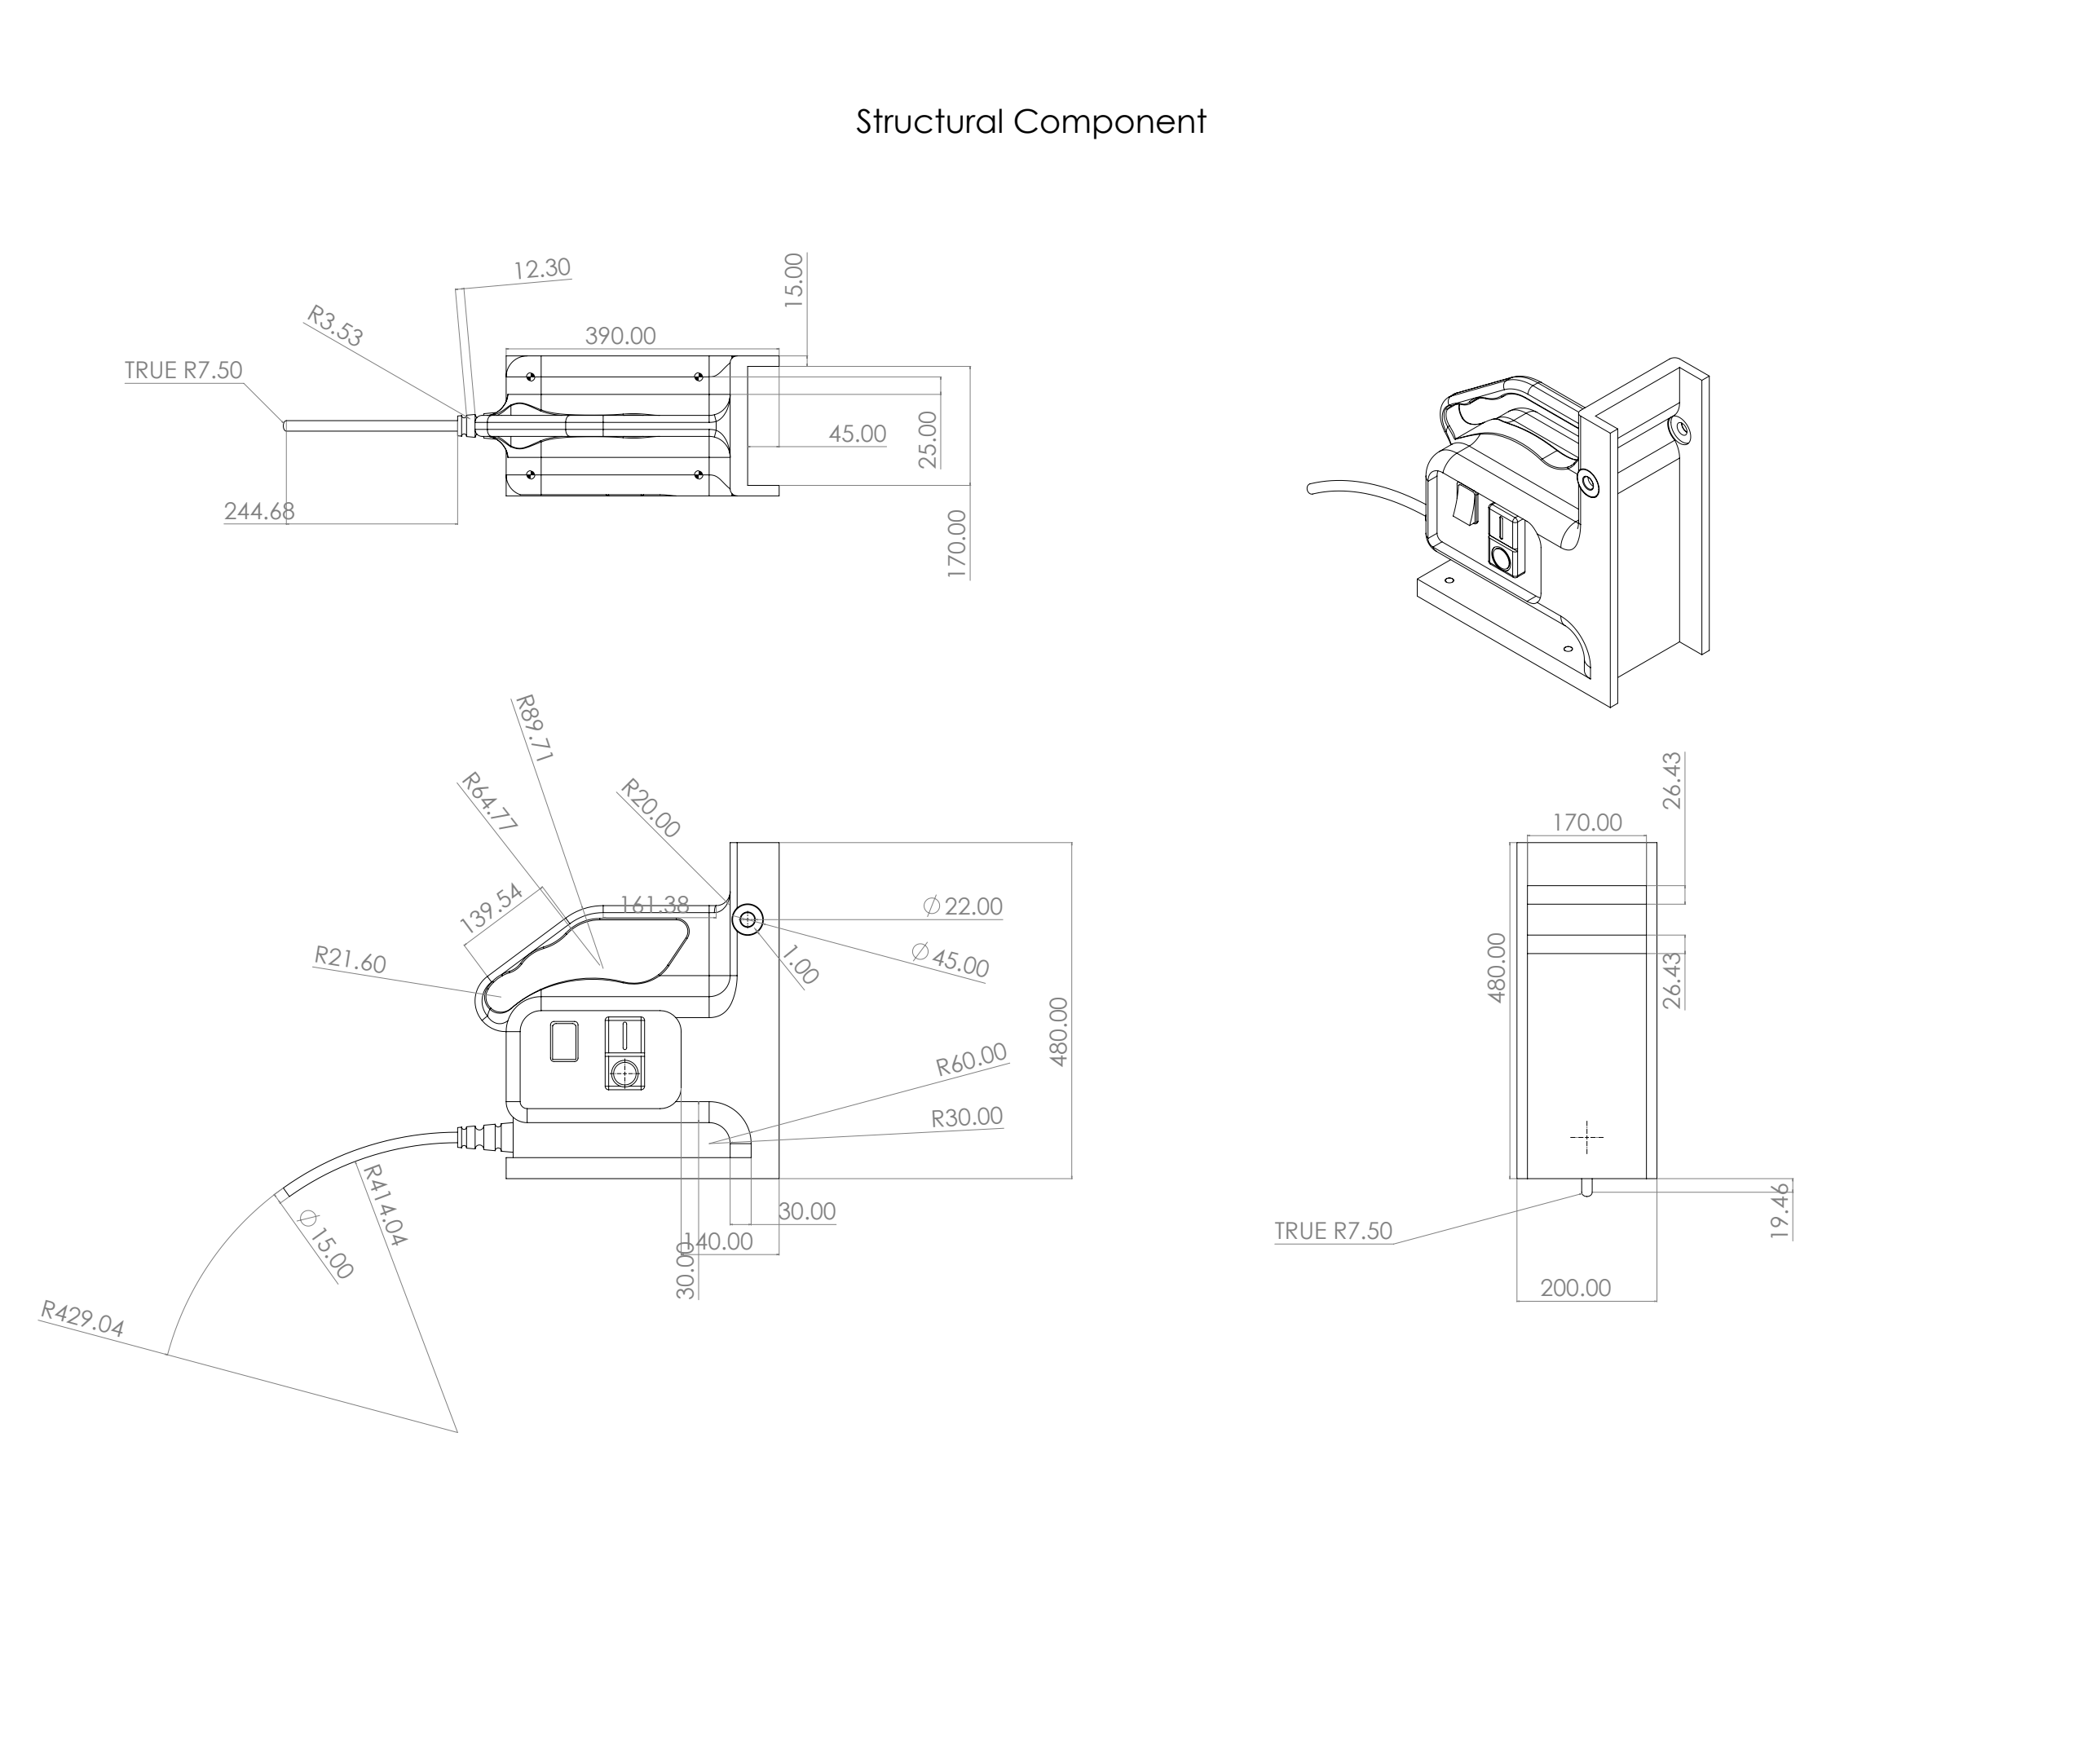
ISO-10303-21;
HEADER;
FILE_DESCRIPTION (('STEP AP214'),
    '1' );
FILE_NAME ('Structural Component.step',
    '2026-10-24T00:09:50',
    ( '' ),
    ( '' ),
    'SwSTEP 2.0',
    'SolidWorks 2025',
    '' );
FILE_SCHEMA (( 'AUTOMOTIVE_DESIGN' ));
ENDSEC;

DATA;
#1=CARTESIAN_POINT ( 'NONE',  ( -209.5848783976569507, 66.48002492874486791, 33.34538701106990288 ) ) ;
#3=DIRECTION ( 'NONE',  ( 0.000000000000000000, 0.000000000000000000, 1.000000000000000000 ) ) ;
#5=EDGE_LOOP ( 'NONE', ( #5978, #27245, #13781, #25937 ) ) ;
#6=CARTESIAN_POINT ( 'NONE',  ( -167.9302994091366088, 116.8073761394556271, 25.31690238253929337 ) ) ;
#7=CARTESIAN_POINT ( 'NONE',  ( -110.7275636018716654, 68.51688903468615877, 83.00000000000001421 ) ) ;
#9=ADVANCED_FACE ( 'NONE', ( #20080 ), #15026, .T. ) ;
#11=ORIENTED_EDGE ( 'NONE', *, *, #16841, .T. ) ;
#13=FACE_OUTER_BOUND ( 'NONE', #24456, .T. ) ;
#15=DIRECTION ( 'NONE',  ( -1.850371707708594316E-16, 1.000000000000000000, 0.000000000000000000 ) ) ;
#18=AXIS2_PLACEMENT_3D ( 'NONE', #21734, #15134, #6353 ) ;
#21=ORIENTED_EDGE ( 'NONE', *, *, #17846, .F. ) ;
#22=CARTESIAN_POINT ( 'NONE',  ( -225.2031547890646266, 89.29438079543466245, 14.16277051160506417 ) ) ;
#24=EDGE_CURVE ( 'NONE', #6807, #15188, #4704, .T. ) ;
#28=AXIS2_PLACEMENT_3D ( 'NONE', #2667, #6838, #19914 ) ;
#38=DIRECTION ( 'NONE',  ( -1.541976423090495387E-16, 1.000000000000000000, -0.000000000000000000 ) ) ;
#43=CARTESIAN_POINT ( 'NONE',  ( -192.2110555254130020, 101.5793329107164027, -32.81765284612617251 ) ) ;
#44=EDGE_LOOP ( 'NONE', ( #26670, #4164, #18942, #22598 ) ) ;
#45=ORIENTED_EDGE ( 'NONE', *, *, #2403, .F. ) ;
#47=AXIS2_PLACEMENT_3D ( 'NONE', #22544, #2851, #8648 ) ;
#50=EDGE_LOOP ( 'NONE', ( #21785, #9635, #7693, #13143 ) ) ;
#52=EDGE_CURVE ( 'NONE', #5857, #12779, #18225, .T. ) ;
#55=DIRECTION ( 'NONE',  ( 1.000000000000000000, 0.000000000000000000, 0.000000000000000000 ) ) ;
#63=CARTESIAN_POINT ( 'NONE',  ( -112.3221550338875687, 74.54464929955099706, 83.00000000000001421 ) ) ;
#66=ORIENTED_EDGE ( 'NONE', *, *, #15793, .T. ) ;
#67=EDGE_CURVE ( 'NONE', #4321, #27397, #9743, .T. ) ;
#69=ORIENTED_EDGE ( 'NONE', *, *, #8545, .T. ) ;
#72=CARTESIAN_POINT ( 'NONE',  ( -242.2383635333241614, 73.34843395317835757, -5.047097023363151358 ) ) ;
#73=CARTESIAN_POINT ( 'NONE',  ( -40.40953891503691153, 36.92584315232891612, 99.00000000000000000 ) ) ;
#84=EDGE_CURVE ( 'NONE', #1460, #15527, #3074, .T. ) ;
#86=DIRECTION ( 'NONE',  ( 0.000000000000000000, 1.000000000000000000, -1.224646799147353207E-16 ) ) ;
#88=VERTEX_POINT ( 'NONE', #22953 ) ;
#90=CARTESIAN_POINT ( 'NONE',  ( 100.8286702512290418, 242.7181571222456284, 23.14229345413787442 ) ) ;
#93=CYLINDRICAL_SURFACE ( 'NONE', #27056, 5.999999999999991118 ) ;
#97=LINE ( 'NONE', #21929, #236 ) ;
#98=CARTESIAN_POINT ( 'NONE',  ( -210.7172313291012529, 103.7585653882801182, 5.000000000000002665 ) ) ;
#99=DIRECTION ( 'NONE',  ( -1.000000000000000000, 0.000000000000000000, 0.000000000000000000 ) ) ;
#101=CARTESIAN_POINT ( 'NONE',  ( 134.9999999999998579, 220.0000000000000284, -99.00000000000001421 ) ) ;
#103=DIRECTION ( 'NONE',  ( 0.5975062131282554700, -0.8018642810807398158, 0.000000000000000000 ) ) ;
#104=ORIENTED_EDGE ( 'NONE', *, *, #18254, .F. ) ;
#115=CARTESIAN_POINT ( 'NONE',  ( -25.41017935548559947, 129.2224694249450181, -15.66087358766781534 ) ) ;
#118=ORIENTED_EDGE ( 'NONE', *, *, #15885, .F. ) ;
#121=ORIENTED_EDGE ( 'NONE', *, *, #12188, .T. ) ;
#122=DIRECTION ( 'NONE',  ( -1.850371707708594316E-16, 1.000000000000000000, -0.000000000000000000 ) ) ;
#124=EDGE_CURVE ( 'NONE', #26591, #26642, #21635, .T. ) ;
#126=DIRECTION ( 'NONE',  ( -1.000000000000000000, 0.000000000000000000, 0.000000000000000000 ) ) ;
#128=CARTESIAN_POINT ( 'NONE',  ( -216.1549772618016334, 59.20708407665082262, 28.62293862808999734 ) ) ;
#132=ADVANCED_FACE ( 'NONE', ( #14200 ), #4989, .F. ) ;
#133=DIRECTION ( 'NONE',  ( 0.000000000000000000, 0.000000000000000000, 1.000000000000000000 ) ) ;
#134=DIRECTION ( 'NONE',  ( -8.673617379884073683E-17, -1.000000000000000000, 0.000000000000000000 ) ) ;
#135=CIRCLE ( 'NONE', #13922, 19.07743405327024888 ) ;
#136=CARTESIAN_POINT ( 'NONE',  ( -203.1779787704217313, 93.05164332230201296, -28.77272332722132475 ) ) ;
#139=DIRECTION ( 'NONE',  ( 0.000000000000000000, 0.000000000000000000, 1.000000000000000000 ) ) ;
#142=EDGE_CURVE ( 'NONE', #11100, #5099, #795, .T. ) ;
#147=LINE ( 'NONE', #4014, #25212 ) ;
#149=EDGE_CURVE ( 'NONE', #7691, #16820, #7209, .T. ) ;
#155=TOROIDAL_SURFACE ( 'NONE', #2900, 39.99999999999999289, 9.999999999999996447 ) ;
#157=CARTESIAN_POINT ( 'NONE',  ( -107.7774523778934253, 133.6573832689441019, 15.67481254453494088 ) ) ;
#158=ORIENTED_EDGE ( 'NONE', *, *, #7014, .F. ) ;
#160=CARTESIAN_POINT ( 'NONE',  ( 94.38583646779612479, 113.6320904522268336, -99.99999999997839950 ) ) ;
#163=CARTESIAN_POINT ( 'NONE',  ( -209.0375512581602493, 88.61097887464748624, 26.00739845333608358 ) ) ;
#165=CARTESIAN_POINT ( 'NONE',  ( -205.7061355896894383, 146.0477147645469813, 12.99999999999999822 ) ) ;
#171=AXIS2_PLACEMENT_3D ( 'NONE', #10028, #18512, #2846 ) ;
#177=CARTESIAN_POINT ( 'NONE',  ( 48.45469728424487244, 192.9461374953035033, 12.99999999999999822 ) ) ;
#182=LINE ( 'NONE', #19713, #24117 ) ;
#183=ORIENTED_EDGE ( 'NONE', *, *, #24834, .F. ) ;
#185=ORIENTED_EDGE ( 'NONE', *, *, #10567, .T. ) ;
#188=CARTESIAN_POINT ( 'NONE',  ( -196.6905515939650400, 98.40619709718011165, -31.75569965019813523 ) ) ;
#192=CARTESIAN_POINT ( 'NONE',  ( -111.8131014667890213, 70.11474204378114905, 82.89209462293977992 ) ) ;
#193=CARTESIAN_POINT ( 'NONE',  ( 109.9999999999998863, 330.0000000000000000, 90.00000000000002842 ) ) ;
#195=ORIENTED_EDGE ( 'NONE', *, *, #27994, .T. ) ;
#197=CARTESIAN_POINT ( 'NONE',  ( -200.0000000000000284, -91.18033988749901653, 21.20097097723064294 ) ) ;
#203=CARTESIAN_POINT ( 'NONE',  ( -209.9813599551185916, 61.38898174817780529, -24.60129468178291035 ) ) ;
#204=CARTESIAN_POINT ( 'NONE',  ( -63.57415822541634043, -18.01420295945611727, 95.00000000000000000 ) ) ;
#205=EDGE_CURVE ( 'NONE', #9863, #2501, #3463, .T. ) ;
#206=EDGE_CURVE ( 'NONE', #17779, #12189, #27834, .T. ) ;
#210=CARTESIAN_POINT ( 'NONE',  ( 184.9999999999999432, 330.0000000000000000, 84.99999999999995737 ) ) ;
#215=EDGE_LOOP ( 'NONE', ( #22439, #1141, #3307, #4955, #12631, #20188 ) ) ;
#218=DIRECTION ( 'NONE',  ( -1.541976423090495387E-16, 1.000000000000000000, 0.000000000000000000 ) ) ;
#223=VERTEX_POINT ( 'NONE', #1394 ) ;
#225=CARTESIAN_POINT ( 'NONE',  ( -210.1746890037166793, 73.83603441591317562, 34.06685219078467242 ) ) ;
#227=ADVANCED_FACE ( 'NONE', ( #3967, #12753 ), #21493, .F. ) ;
#230=VERTEX_POINT ( 'NONE', #6412 ) ;
#235=CARTESIAN_POINT ( 'NONE',  ( -220.9647007329185158, 136.4514858755404987, 12.97939780113086705 ) ) ;
#236=VECTOR ( 'NONE', #2100, 1000.000000000000000 ) ;
#239=CARTESIAN_POINT ( 'NONE',  ( 103.5789823554282947, 245.2557385300782471, 18.86932834259753733 ) ) ;
#240=EDGE_CURVE ( 'NONE', #11439, #27657, #27406, .T. ) ;
#250=DIRECTION ( 'NONE',  ( 8.659560562354934091E-17, 0.7071067811865474617, -0.7071067811865476838 ) ) ;
#253=DIRECTION ( 'NONE',  ( 0.4163300014277677707, -0.9092135777204137792, 0.000000000000000000 ) ) ;
#255=DIRECTION ( 'NONE',  ( 0.000000000000000000, 0.000000000000000000, -1.000000000000000000 ) ) ;
#259=EDGE_CURVE ( 'NONE', #1752, #10216, #14126, .T. ) ;
#261=ORIENTED_EDGE ( 'NONE', *, *, #205, .F. ) ;
#264=AXIS2_PLACEMENT_3D ( 'NONE', #19395, #6183, #2008 ) ;
#266=ORIENTED_EDGE ( 'NONE', *, *, #2989, .F. ) ;
#267=ORIENTED_EDGE ( 'NONE', *, *, #6042, .T. ) ;
#269=DIRECTION ( 'NONE',  ( 0.000000000000000000, 0.000000000000000000, 1.000000000000000000 ) ) ;
#270=CARTESIAN_POINT ( 'NONE',  ( -180.0000000000000284, -40.00000000000004974, 70.00000000000001421 ) ) ;
#277=FACE_OUTER_BOUND ( 'NONE', #22057, .T. ) ;
#279=CARTESIAN_POINT ( 'NONE',  ( -212.2468527728169931, 60.00277588997245459, 15.59298365948827225 ) ) ;
#282=B_SPLINE_CURVE_WITH_KNOTS ( 'NONE', 3,
 ( #2142, #28138, #4579, #11204, #26414, #10916, #13506, #17233, #1, #2281, #25992, #19677, #22257, #19813, #6311, #13087, #23849, #13365 ),
 .UNSPECIFIED., .F., .F.,
 ( 4, 2, 2, 2, 2, 2, 2, 2, 4 ),
 ( -3.464102035643382632E-05, 0.004053789758800030972, 0.008142220537956495682, 0.01223065131711295953, 0.01631908209626942510, 0.02449594365458239789, 0.02654015904416063762, 0.02858437443373887041, 0.03267280521289535333 ),
 .UNSPECIFIED. ) ;
#285=ADVANCED_FACE ( 'NONE', ( #4393 ), #15978, .T. ) ;
#291=CARTESIAN_POINT ( 'NONE',  ( -160.0000000000000284, 119.7660240611718763, 22.85081902853005431 ) ) ;
#292=DIRECTION ( 'NONE',  ( 1.000000000000000000, 0.000000000000000000, 0.000000000000000000 ) ) ;
#294=ORIENTED_EDGE ( 'NONE', *, *, #2530, .T. ) ;
#295=CARTESIAN_POINT ( 'NONE',  ( -222.7702326850704821, 86.58333552780506182, -17.42169760653345634 ) ) ;
#297=CARTESIAN_POINT ( 'NONE',  ( -204.4166662746044665, 91.57150914865317759, -29.20755859028324508 ) ) ;
#303=CARTESIAN_POINT ( 'NONE',  ( -156.4144565615572731, 122.2051147660285579, 19.70699073531202572 ) ) ;
#305=AXIS2_PLACEMENT_3D ( 'NONE', #16749, #21045, #18753 ) ;
#308=CYLINDRICAL_SURFACE ( 'NONE', #13262, 19.07743405327024888 ) ;
#310=ADVANCED_FACE ( 'NONE', ( #4526 ), #6410, .T. ) ;
#311=CARTESIAN_POINT ( 'NONE',  ( -207.4306580894464389, 90.17638659202999918, 25.66226923892150324 ) ) ;
#313=EDGE_CURVE ( 'NONE', #4881, #7087, #25948, .T. ) ;
#318=CIRCLE ( 'NONE', #8106, 1.999999999999994893 ) ;
#319=CARTESIAN_POINT ( 'NONE',  ( -218.1276041038538551, 59.80742093790404112, -25.66002785714302803 ) ) ;
#320=ORIENTED_EDGE ( 'NONE', *, *, #18339, .T. ) ;
#322=CARTESIAN_POINT ( 'NONE',  ( -225.9601317720483280, 132.4444111280268430, -15.07876772300364010 ) ) ;
#323=DIRECTION ( 'NONE',  ( 0.000000000000000000, 0.000000000000000000, 1.000000000000000000 ) ) ;
#328=CARTESIAN_POINT ( 'NONE',  ( -138.6428522700808230, 71.54464929955099706, 82.80879831960034210 ) ) ;
#331=DIRECTION ( 'NONE',  ( -0.6343833064826072121, 0.7730186417261841747, 0.000000000000000000 ) ) ;
#332=CARTESIAN_POINT ( 'NONE',  ( 0.000000000000000000, 0.000000000000000000, 100.0000000000000000 ) ) ;
#335=ORIENTED_EDGE ( 'NONE', *, *, #12580, .F. ) ;
#336=FACE_OUTER_BOUND ( 'NONE', #23638, .T. ) ;
#337=ADVANCED_FACE ( 'NONE', ( #27449 ), #5770, .T. ) ;
#339=DIRECTION ( 'NONE',  ( 0.000000000000000000, 0.000000000000000000, 1.000000000000000000 ) ) ;
#342=DIRECTION ( 'NONE',  ( 1.000000000000000000, 0.000000000000000000, 0.000000000000000000 ) ) ;
#347=CARTESIAN_POINT ( 'NONE',  ( -20.36124356129798940, 129.6266993258962259, -15.48147584998389448 ) ) ;
#349=CARTESIAN_POINT ( 'NONE',  ( -200.0000000000000284, -62.36067977499792647, -25.00000000000000000 ) ) ;
#361=CARTESIAN_POINT ( 'NONE',  ( -212.8228108689317253, 60.01962377528476367, -15.18702394368705910 ) ) ;
#362=DIRECTION ( 'NONE',  ( -0.000000000000000000, -0.000000000000000000, 1.000000000000000000 ) ) ;
#366=VERTEX_POINT ( 'NONE', #3605 ) ;
#373=DIRECTION ( 'NONE',  ( 1.000000000000000000, 0.000000000000000000, 0.000000000000000000 ) ) ;
#377=AXIS2_PLACEMENT_3D ( 'NONE', #16713, #14560, #19139 ) ;
#380=CARTESIAN_POINT ( 'NONE',  ( 93.89426149341781525, 239.9406732612975475, 18.26413231115399682 ) ) ;
#383=DIRECTION ( 'NONE',  ( 0.000000000000000000, 0.000000000000000000, 1.000000000000000000 ) ) ;
#384=DIRECTION ( 'NONE',  ( -0.000000000000000000, -0.000000000000000000, -1.000000000000000000 ) ) ;
#385=DIRECTION ( 'NONE',  ( 0.000000000000000000, 0.000000000000000000, 1.000000000000000000 ) ) ;
#393=DIRECTION ( 'NONE',  ( -0.8498245983676009363, -0.3891357156574876686, 0.3554877590144011057 ) ) ;
#401=DIRECTION ( 'NONE',  ( 0.000000000000000000, 0.000000000000000000, -1.000000000000000000 ) ) ;
#402=ORIENTED_EDGE ( 'NONE', *, *, #11663, .T. ) ;
#406=EDGE_CURVE ( 'NONE', #3986, #26642, #16284, .T. ) ;
#407=VECTOR ( 'NONE', #3303, 1000.000000000000000 ) ;
#408=EDGE_LOOP ( 'NONE', ( #9219, #25469, #5579, #24964 ) ) ;
#411=ORIENTED_EDGE ( 'NONE', *, *, #8546, .F. ) ;
#415=AXIS2_PLACEMENT_3D ( 'NONE', #13536, #20551, #20125 ) ;
#416=CYLINDRICAL_SURFACE ( 'NONE', #20614, 5.000000000000004441 ) ;
#417=CARTESIAN_POINT ( 'NONE',  ( -8.428214953819216149, 132.5195342171013806, 14.39912748063941983 ) ) ;
#419=CARTESIAN_POINT ( 'NONE',  ( -217.7467898461135576, 60.55642267084821384, 12.19614748119721703 ) ) ;
#425=CARTESIAN_POINT ( 'NONE',  ( -42.99650729631200363, 71.03850157808263077, 100.0000000000000000 ) ) ;
#428=AXIS2_PLACEMENT_3D ( 'NONE', #23182, #1479, #8092 ) ;
#429=CARTESIAN_POINT ( 'NONE',  ( 8.117852850209660076, 141.5785587194356481, 12.99999999999999467 ) ) ;
#430=CARTESIAN_POINT ( 'NONE',  ( 109.9999999999999005, 260.0000000000000000, 45.00000000000000000 ) ) ;
#438=VECTOR ( 'NONE', #7033, 1000.000000000000000 ) ;
#439=CARTESIAN_POINT ( 'NONE',  ( -175.0000000000000000, -120.0250000000001904, -76.00000000000000000 ) ) ;
#440=CARTESIAN_POINT ( 'NONE',  ( -203.3278902001933659, 92.92226908766613747, -29.32321494459340627 ) ) ;
#441=ORIENTED_EDGE ( 'NONE', *, *, #25815, .T. ) ;
#442=ORIENTED_EDGE ( 'NONE', *, *, #67, .F. ) ;
#443=ADVANCED_FACE ( 'NONE', ( #16699 ), #5898, .T. ) ;
#445=EDGE_CURVE ( 'NONE', #15077, #27477, #22877, .T. ) ;
#446=CYLINDRICAL_SURFACE ( 'NONE', #26258, 30.00000000000000000 ) ;
#449=ORIENTED_EDGE ( 'NONE', *, *, #2534, .F. ) ;
#453=ORIENTED_EDGE ( 'NONE', *, *, #4349, .T. ) ;
#459=CARTESIAN_POINT ( 'NONE',  ( -213.5622695550096353, 60.06483686772719466, -14.69413405016890017 ) ) ;
#462=CARTESIAN_POINT ( 'NONE',  ( -224.0127348693990257, 134.1242697789267027, -15.11921763785539774 ) ) ;
#466=DIRECTION ( 'NONE',  ( 1.000000000000000000, -0.000000000000000000, 0.000000000000000000 ) ) ;
#467=VECTOR ( 'NONE', #25215, 1000.000000000000000 ) ;
#471=ORIENTED_EDGE ( 'NONE', *, *, #8870, .T. ) ;
#474=VECTOR ( 'NONE', #16394, 1000.000000000000000 ) ;
#476=DIRECTION ( 'NONE',  ( -1.000000000000000000, -9.251858538542961967E-16, 0.000000000000000000 ) ) ;
#480=FACE_OUTER_BOUND ( 'NONE', #21815, .T. ) ;
#483=ORIENTED_EDGE ( 'NONE', *, *, #21141, .F. ) ;
#484=CARTESIAN_POINT ( 'NONE',  ( -40.77925748874363165, 129.1862645484492020, 17.01096724815181460 ) ) ;
#489=CARTESIAN_POINT ( 'NONE',  ( 8.117852850209603233, 141.5785587194356197, -15.00000000000000000 ) ) ;
#490=DIRECTION ( 'NONE',  ( -1.000000000000000000, 0.000000000000000000, 0.000000000000000000 ) ) ;
#492=CIRCLE ( 'NONE', #5533, 1.999999999999996669 ) ;
#493=FACE_OUTER_BOUND ( 'NONE', #792, .T. ) ;
#494=ORIENTED_EDGE ( 'NONE', *, *, #19922, .T. ) ;
#498=DIRECTION ( 'NONE',  ( 1.000000000000000000, -0.000000000000000000, -0.000000000000000000 ) ) ;
#501=LINE ( 'NONE', #24916, #3156 ) ;
#504=FACE_OUTER_BOUND ( 'NONE', #21590, .T. ) ;
#508=EDGE_CURVE ( 'NONE', #26994, #8764, #18328, .T. ) ;
#512=CARTESIAN_POINT ( 'NONE',  ( -207.5836773499184176, 75.53976764568116664, 42.88623166414009091 ) ) ;
#517=ORIENTED_EDGE ( 'NONE', *, *, #21468, .T. ) ;
#520=VECTOR ( 'NONE', #1855, 1000.000000000000000 ) ;
#521=ORIENTED_EDGE ( 'NONE', *, *, #18351, .F. ) ;
#523=CARTESIAN_POINT ( 'NONE',  ( 94.98941689213133088, 231.7050943134730687, 19.00901305069102065 ) ) ;
#527=CARTESIAN_POINT ( 'NONE',  ( -110.3221550338875687, 20.24192588826928585, 83.00000000000001421 ) ) ;
#528=CYLINDRICAL_SURFACE ( 'NONE', #15262, 22.49999999999999289 ) ;
#529=TOROIDAL_SURFACE ( 'NONE', #23467, 19.29759039828519818, 4.355764593064427537 ) ;
#530=CARTESIAN_POINT ( 'NONE',  ( -190.0000000000000284, 59.99999999999995026, 110.0000000000000284 ) ) ;
#533=CARTESIAN_POINT ( 'NONE',  ( 22.58950924271104554, 154.2349915562422780, 12.99999999999999822 ) ) ;
#536=ORIENTED_EDGE ( 'NONE', *, *, #7121, .T. ) ;
#538=CIRCLE ( 'NONE', #24856, 60.90601976618767566 ) ;
#541=CARTESIAN_POINT ( 'NONE',  ( 139.9999999999999716, -120.0000000000000995, 100.0000000000000142 ) ) ;
#544=CARTESIAN_POINT ( 'NONE',  ( 108.8501248000116277, 253.0299650808884735, -36.51570041470898076 ) ) ;
#549=EDGE_CURVE ( 'NONE', #10475, #4407, #3984, .T. ) ;
#554=VECTOR ( 'NONE', #22307, 1000.000000000000000 ) ;
#555=CARTESIAN_POINT ( 'NONE',  ( -92.89766067256680060, 136.4115285999503158, 13.49165197499294599 ) ) ;
#556=DIRECTION ( 'NONE',  ( 1.000000000000000000, 0.000000000000000000, 0.000000000000000000 ) ) ;
#559=CARTESIAN_POINT ( 'NONE',  ( -97.83215868775270962, 136.0971436861518669, -15.20870553203125120 ) ) ;
#562=CARTESIAN_POINT ( 'NONE',  ( -218.4636426211929177, 60.67881959240470735, 11.81164476506740790 ) ) ;
#565=DIRECTION ( 'NONE',  ( 0.5975062131282562472, -0.8018642810807392607, 0.000000000000000000 ) ) ;
#566=CARTESIAN_POINT ( 'NONE',  ( -229.8938360676123978, 91.85985842061924700, -13.11794914285764690 ) ) ;
#567=DIRECTION ( 'NONE',  ( -0.8142945039115421224, -0.5804519453834706688, 0.000000000000000000 ) ) ;
#568=DIRECTION ( 'NONE',  ( 1.000000000000000000, -0.000000000000000000, -0.000000000000000000 ) ) ;
#572=CARTESIAN_POINT ( 'NONE',  ( -18.11108351247773385, 129.9683555792950358, 15.33266781369627907 ) ) ;
#575=CARTESIAN_POINT ( 'NONE',  ( -107.3221550338875687, 17.24192588826928585, 83.00000000000001421 ) ) ;
#576=AXIS2_PLACEMENT_3D ( 'NONE', #27144, #7193, #11366 ) ;
#578=ORIENTED_EDGE ( 'NONE', *, *, #27825, .F. ) ;
#581=DIRECTION ( 'NONE',  ( 1.000000000000000000, 0.000000000000000000, 0.000000000000000000 ) ) ;
#584=EDGE_LOOP ( 'NONE', ( #16630, #25625, #9572, #10611, #8685 ) ) ;
#587=EDGE_CURVE ( 'NONE', #6088, #15077, #9133, .T. ) ;
#589=ORIENTED_EDGE ( 'NONE', *, *, #6265, .F. ) ;
#593=DIRECTION ( 'NONE',  ( 0.000000000000000000, 0.000000000000000000, -1.000000000000000000 ) ) ;
#595=DIRECTION ( 'NONE',  ( 0.000000000000000000, 0.000000000000000000, 1.000000000000000000 ) ) ;
#597=CARTESIAN_POINT ( 'NONE',  ( -205.5646887631684763, 90.70208198090838891, 28.50398098557788273 ) ) ;
#600=EDGE_CURVE ( 'NONE', #17042, #11042, #25180, .T. ) ;
#601=VECTOR ( 'NONE', #28078, 1000.000000000000000 ) ;
#604=CARTESIAN_POINT ( 'NONE',  ( 109.9999999999999005, 240.0000000000000284, 15.00000000000000000 ) ) ;
#605=CARTESIAN_POINT ( 'NONE',  ( -214.3579997887104298, 72.01340221155322752, -27.44224251620622113 ) ) ;
#606=VERTEX_POINT ( 'NONE', #11525 ) ;
#611=CARTESIAN_POINT ( 'NONE',  ( -200.0000000000000284, 0.000000000000000000, -25.00000000000000000 ) ) ;
#614=CARTESIAN_POINT ( 'NONE',  ( 46.79174272583949801, 194.0572550123460474, 12.99999999999999822 ) ) ;
#616=FACE_OUTER_BOUND ( 'NONE', #8502, .T. ) ;
#621=CARTESIAN_POINT ( 'NONE',  ( 81.45493510940914916, 110.0000000000000142, 70.00000000030220804 ) ) ;
#622=CARTESIAN_POINT ( 'NONE',  ( -266.5839533485339530, -91.18033988749901653, -15.26911010665567225 ) ) ;
#623=ORIENTED_EDGE ( 'NONE', *, *, #7231, .T. ) ;
#625=CARTESIAN_POINT ( 'NONE',  ( 134.9999999999998579, 220.0000000000000284, 99.00000000000001421 ) ) ;
#634=DIRECTION ( 'NONE',  ( 0.000000000000000000, 0.000000000000000000, -1.000000000000000000 ) ) ;
#635=CARTESIAN_POINT ( 'NONE',  ( 0.6797495551325769547, 136.5999822166548370, -13.39362083918624968 ) ) ;
#639=CARTESIAN_POINT ( 'NONE',  ( 179.9999999999999147, -150.0000000000000284, 84.99999999999995737 ) ) ;
#644=DIRECTION ( 'NONE',  ( -0.000000000000000000, -0.000000000000000000, -1.000000000000000000 ) ) ;
#647=DIRECTION ( 'NONE',  ( 0.5555587585212683477, 0.8314772792026894344, -0.000000000000000000 ) ) ;
#653=CARTESIAN_POINT ( 'NONE',  ( 109.9999999999999005, 260.0000000000000000, 45.00000000000000000 ) ) ;
#654=ORIENTED_EDGE ( 'NONE', *, *, #6112, .T. ) ;
#656=FACE_OUTER_BOUND ( 'NONE', #25895, .T. ) ;
#657=ORIENTED_EDGE ( 'NONE', *, *, #26807, .T. ) ;
#658=CARTESIAN_POINT ( 'NONE',  ( 91.94652509811839991, 240.0740392588532757, 7.116191647120904129 ) ) ;
#661=ORIENTED_EDGE ( 'NONE', *, *, #5035, .T. ) ;
#665=EDGE_LOOP ( 'NONE', ( #21, #21281, #16990, #8206, #12330, #23398, #10718, #5703 ) ) ;
#667=CARTESIAN_POINT ( 'NONE',  ( 101.4665947576538372, 243.5985648160911410, 15.64809332289330435 ) ) ;
#671=CARTESIAN_POINT ( 'NONE',  ( 65.00000000000000000, -150.0000000000000568, -69.99999999999998579 ) ) ;
#672=CIRCLE ( 'NONE', #14906, 1.999999999999998890 ) ;
#673=ADVANCED_FACE ( 'NONE', ( #13529 ), #308, .F. ) ;
#675=CARTESIAN_POINT ( 'NONE',  ( 81.45493510941093973, 110.0000000000000142, -70.00000000034538061 ) ) ;
#677=FACE_OUTER_BOUND ( 'NONE', #5, .T. ) ;
#682=DIRECTION ( 'NONE',  ( 1.000000000000000000, 0.000000000000000000, 0.000000000000000000 ) ) ;
#683=DIRECTION ( 'NONE',  ( 1.000000000000000000, 0.000000000000000000, 0.000000000000000000 ) ) ;
#687=CYLINDRICAL_SURFACE ( 'NONE', #19940, 10.00000000000000888 ) ;
#688=DIRECTION ( 'NONE',  ( 0.000000000000000000, -1.000000000000000000, 0.000000000000000000 ) ) ;
#691=ORIENTED_EDGE ( 'NONE', *, *, #13967, .F. ) ;
#698=DIRECTION ( 'NONE',  ( 0.000000000000000000, 0.000000000000000000, -1.000000000000000000 ) ) ;
#700=CARTESIAN_POINT ( 'NONE',  ( 87.49999999999990052, 230.0000000000000284, 15.95262490344436657 ) ) ;
#702=ADVANCED_FACE ( 'NONE', ( #13675 ), #26432, .T. ) ;
#703=CARTESIAN_POINT ( 'NONE',  ( -101.5016674773769694, 134.2040548686907755, -15.56499774383584622 ) ) ;
#704=DIRECTION ( 'NONE',  ( -0.000000000000000000, -0.000000000000000000, -1.000000000000000000 ) ) ;
#705=CARTESIAN_POINT ( 'NONE',  ( -195.1986077931981356, 62.83738171803135231, 37.97438512083786577 ) ) ;
#707=CARTESIAN_POINT ( 'NONE',  ( 14.21936997543395798, -49.77566109691134955, 98.36633331184400220 ) ) ;
#708=EDGE_CURVE ( 'NONE', #12779, #28035, #2160, .T. ) ;
#714=VECTOR ( 'NONE', #4678, 1000.000000000000000 ) ;
#715=CARTESIAN_POINT ( 'NONE',  ( 109.9999999999999147, 140.0000000000000000, 90.00000000000002842 ) ) ;
#717=CARTESIAN_POINT ( 'NONE',  ( 65.00000000000000000, -120.0000000000000711, 70.00000000000001421 ) ) ;
#719=CARTESIAN_POINT ( 'NONE',  ( 118.4313905927012343, 122.3304618272157569, -100.0000000000000142 ) ) ;
#724=CARTESIAN_POINT ( 'NONE',  ( -207.1027104522468392, 89.68341047235171004, -27.43904842249505194 ) ) ;
#726=ORIENTED_EDGE ( 'NONE', *, *, #26630, .F. ) ;
#728=CARTESIAN_POINT ( 'NONE',  ( -144.8818860832173527, 126.6487520769749580, 16.84620022481251311 ) ) ;
#731=CARTESIAN_POINT ( 'NONE',  ( -173.1201715254111662, 113.5802963645813151, -28.20029687320744216 ) ) ;
#737=CARTESIAN_POINT ( 'NONE',  ( -203.3278902001933375, 92.92226908766613747, 29.32321494459339561 ) ) ;
#739=LINE ( 'NONE', #24727, #13957 ) ;
#742=CARTESIAN_POINT ( 'NONE',  ( -213.9337484054510128, 55.48171494544713056, -43.35284082257812344 ) ) ;
#746=CARTESIAN_POINT ( 'NONE',  ( -227.8378063125350366, 130.6400894613935577, -13.00000000000000178 ) ) ;
#752=CARTESIAN_POINT ( 'NONE',  ( -236.2622743973914510, 68.21227378728754331, 5.744226217424930780 ) ) ;
#755=AXIS2_PLACEMENT_3D ( 'NONE', #22509, #5114, #11751 ) ;
#757=EDGE_CURVE ( 'NONE', #11653, #6227, #3168, .T. ) ;
#760=FACE_OUTER_BOUND ( 'NONE', #17355, .T. ) ;
#763=CARTESIAN_POINT ( 'NONE',  ( -63.57415822541634043, 0.000000000000000000, 95.00000000000000000 ) ) ;
#764=CARTESIAN_POINT ( 'NONE',  ( -76.25760768171836901, 154.8982798170083299, 12.99999999999999822 ) ) ;
#766=ORIENTED_EDGE ( 'NONE', *, *, #9211, .F. ) ;
#769=CIRCLE ( 'NONE', #28282, 17.46154499483315448 ) ;
#770=DIRECTION ( 'NONE',  ( -0.000000000000000000, -0.000000000000000000, 1.000000000000000000 ) ) ;
#771=CARTESIAN_POINT ( 'NONE',  ( 33.10302365956999182, 219.6666220619077876, -13.00000000000000000 ) ) ;
#773=CARTESIAN_POINT ( 'NONE',  ( -7.443950587159290144, 132.8771115358387931, -14.28760955781909381 ) ) ;
#774=FACE_OUTER_BOUND ( 'NONE', #27445, .T. ) ;
#777=DIRECTION ( 'NONE',  ( 1.000000000000000000, 0.000000000000000000, 0.000000000000000000 ) ) ;
#782=FACE_OUTER_BOUND ( 'NONE', #22813, .T. ) ;
#783=DIRECTION ( 'NONE',  ( 0.000000000000000000, 0.000000000000000000, -1.000000000000000000 ) ) ;
#786=ORIENTED_EDGE ( 'NONE', *, *, #2510, .F. ) ;
#792=EDGE_LOOP ( 'NONE', ( #26456, #9388, #18385, #15458, #18561, #10831 ) ) ;
#795=CIRCLE ( 'NONE', #16840, 9.999999999999994671 ) ;
#796=FACE_OUTER_BOUND ( 'NONE', #27107, .T. ) ;
#801=EDGE_CURVE ( 'NONE', #19503, #8160, #22570, .T. ) ;
#804=EDGE_CURVE ( 'NONE', #2005, #223, #27933, .T. ) ;
#807=CARTESIAN_POINT ( 'NONE',  ( 109.9999999999999005, 259.1520133602594456, 44.26562200907745392 ) ) ;
#808=DIRECTION ( 'NONE',  ( -8.673617379884036705E-17, 1.000000000000000000, 0.000000000000000000 ) ) ;
#811=CARTESIAN_POINT ( 'NONE',  ( 85.90765579575543143, 110.5723347142871091, -70.58593750016461854 ) ) ;
#815=CARTESIAN_POINT ( 'NONE',  ( 65.00000000000000000, -150.0000000000000568, 70.00000000000001421 ) ) ;
#820=ORIENTED_EDGE ( 'NONE', *, *, #24259, .F. ) ;
#822=LINE ( 'NONE', #541, #8481 ) ;
#823=CARTESIAN_POINT ( 'NONE',  ( -273.6211430000234373, -91.18033988749901653, 0.000000000000000000 ) ) ;
#827=ORIENTED_EDGE ( 'NONE', *, *, #20728, .F. ) ;
#830=EDGE_CURVE ( 'NONE', #12559, #10408, #23836, .T. ) ;
#832=ORIENTED_EDGE ( 'NONE', *, *, #20807, .T. ) ;
#834=ORIENTED_EDGE ( 'NONE', *, *, #1618, .F. ) ;
#835=CARTESIAN_POINT ( 'NONE',  ( -151.8667954808881291, 124.0669258736115523, 18.37961917418349955 ) ) ;
#841=CARTESIAN_POINT ( 'NONE',  ( -31.50743868999440167, 129.2243496464543284, 15.65998950894569752 ) ) ;
#842=CARTESIAN_POINT ( 'NONE',  ( -195.0250397031994112, 62.90385929084195737, 38.63509848415888115 ) ) ;
#846=CARTESIAN_POINT ( 'NONE',  ( 79.99999999999994316, 109.9999999999999716, -71.96349540849364246 ) ) ;
#847=VECTOR ( 'NONE', #18718, 1000.000000000000114 ) ;
#848=CARTESIAN_POINT ( 'NONE',  ( -207.3935809773778942, 90.19561752971078761, -25.69361353241580304 ) ) ;
#850=DIRECTION ( 'NONE',  ( 0.000000000000000000, 0.000000000000000000, 1.000000000000000000 ) ) ;
#851=CARTESIAN_POINT ( 'NONE',  ( 87.74278500247204704, 111.0010834413667453, 71.13281249985656984 ) ) ;
#853=CARTESIAN_POINT ( 'NONE',  ( 113.4920585194047078, 104.4775165427241461, -100.0000000000000142 ) ) ;
#859=DIRECTION ( 'NONE',  ( -1.000000000000000000, 0.000000000000000000, 0.000000000000000000 ) ) ;
#861=ORIENTED_EDGE ( 'NONE', *, *, #22149, .F. ) ;
#866=EDGE_CURVE ( 'NONE', #16598, #10685, #5021, .T. ) ;
#871=DIRECTION ( 'NONE',  ( 1.000000000000000000, 3.469446951953614189E-16, -0.000000000000000000 ) ) ;
#877=CARTESIAN_POINT ( 'NONE',  ( -199.5809478526699650, 61.42778479158862126, -28.44561038857050761 ) ) ;
#887=DIRECTION ( 'NONE',  ( -0.000000000000000000, 1.000000000000000000, -0.000000000000000000 ) ) ;
#888=EDGE_LOOP ( 'NONE', ( #23960, #2470, #23686, #8733 ) ) ;
#891=CARTESIAN_POINT ( 'NONE',  ( -279.3160071107327553, -91.18033988749901653, 0.000000000000000000 ) ) ;
#896=AXIS2_PLACEMENT_3D ( 'NONE', #9883, #3402, #7727 ) ;
#903=ORIENTED_EDGE ( 'NONE', *, *, #6405, .T. ) ;
#907=CIRCLE ( 'NONE', #10544, 30.00000000000000000 ) ;
#910=CARTESIAN_POINT ( 'NONE',  ( 7.502017008525952768, 138.6551571308461348, -15.00000000000000000 ) ) ;
#912=EDGE_CURVE ( 'NONE', #25311, #7612, #22460, .T. ) ;
#917=FACE_OUTER_BOUND ( 'NONE', #15898, .T. ) ;
#919=LINE ( 'NONE', #10110, #24476 ) ;
#922=CIRCLE ( 'NONE', #10088, 68.83858790703926900 ) ;
#928=ORIENTED_EDGE ( 'NONE', *, *, #17521, .F. ) ;
#929=DIRECTION ( 'NONE',  ( 1.000000000000000000, 0.000000000000000000, 0.000000000000000000 ) ) ;
#933=EDGE_LOOP ( 'NONE', ( #25332, #26932, #17589, #8882, #1061, #19824, #4317, #18042 ) ) ;
#937=ADVANCED_FACE ( 'NONE', ( #14514, #19097, #8178, #25421, #14651 ), #23838, .F. ) ;
#938=CIRCLE ( 'NONE', #21121, 18.91107291867258411 ) ;
#943=VECTOR ( 'NONE', #21161, 1000.000000000000000 ) ;
#944=DIRECTION ( 'NONE',  ( -0.000000000000000000, -1.000000000000000000, -0.000000000000000000 ) ) ;
#945=DIRECTION ( 'NONE',  ( 1.000000000000000000, 0.000000000000000000, 0.000000000000000000 ) ) ;
#946=EDGE_CURVE ( 'NONE', #12013, #2614, #5471, .T. ) ;
#947=CARTESIAN_POINT ( 'NONE',  ( 104.1118574119011555, 122.0584436052145918, -84.84374999967577935 ) ) ;
#955=ORIENTED_EDGE ( 'NONE', *, *, #8077, .T. ) ;
#960=ADVANCED_FACE ( 'NONE', ( #5736 ), #3715, .T. ) ;
#961=FACE_OUTER_BOUND ( 'NONE', #3277, .T. ) ;
#970=VERTEX_POINT ( 'NONE', #8325 ) ;
#971=CARTESIAN_POINT ( 'NONE',  ( -81.43952348080793513, 136.3896988708861215, 13.49547953233103392 ) ) ;
#977=AXIS2_PLACEMENT_3D ( 'NONE', #1019, #14248, #3304 ) ;
#980=CARTESIAN_POINT ( 'NONE',  ( -122.9477694338266360, 132.7606495686108872, -14.33686514723054373 ) ) ;
#986=CARTESIAN_POINT ( 'NONE',  ( 33.10302365956999182, 203.2034914284457159, -15.00000000000000000 ) ) ;
#987=ADVANCED_FACE ( 'NONE', ( #25840 ), #26568, .T. ) ;
#989=CARTESIAN_POINT ( 'NONE',  ( 119.9999999999999147, 140.0000000000000000, -100.0000000000000142 ) ) ;
#990=DIRECTION ( 'NONE',  ( 0.000000000000000000, 0.000000000000000000, 1.000000000000000000 ) ) ;
#993=CIRCLE ( 'NONE', #27137, 166.0121251338587172 ) ;
#997=EDGE_LOOP ( 'NONE', ( #19109, #27348, #25490, #11756, #45, #10235 ) ) ;
#998=CIRCLE ( 'NONE', #19800, 5.000000000000004441 ) ;
#1000=ORIENTED_EDGE ( 'NONE', *, *, #28394, .T. ) ;
#1001=DIRECTION ( 'NONE',  ( -1.850371707708594316E-16, 1.000000000000000000, 0.000000000000000000 ) ) ;
#1004=DIRECTION ( 'NONE',  ( -0.7892793597178160425, -0.6140342761796236948, 0.000000000000000000 ) ) ;
#1006=CARTESIAN_POINT ( 'NONE',  ( -20.22388308534250712, 128.4000958562204460, -17.33254599016412101 ) ) ;
#1008=DIRECTION ( 'NONE',  ( -0.5555587585212683477, -0.8314772792026894344, -0.000000000000000000 ) ) ;
#1009=EDGE_CURVE ( 'NONE', #27752, #3252, #23271, .T. ) ;
#1010=AXIS2_PLACEMENT_3D ( 'NONE', #4400, #24228, #2669 ) ;
#1014=EDGE_CURVE ( 'NONE', #9382, #18102, #26729, .T. ) ;
#1015=AXIS2_PLACEMENT_3D ( 'NONE', #23644, #1520, #25373 ) ;
#1019=CARTESIAN_POINT ( 'NONE',  ( 139.9999999999999716, -120.0000000000000284, 70.00000000000001421 ) ) ;
#1020=FACE_OUTER_BOUND ( 'NONE', #12119, .T. ) ;
#1024=CARTESIAN_POINT ( 'NONE',  ( -242.2202452113856737, 73.32912780459425051, 5.047888127315641960 ) ) ;
#1026=ORIENTED_EDGE ( 'NONE', *, *, #13555, .T. ) ;
#1030=AXIS2_PLACEMENT_3D ( 'NONE', #19427, #23883, #12979 ) ;
#1031=CARTESIAN_POINT ( 'NONE',  ( 84.91648909967247505, 110.3843228249417479, 70.37109374985131183 ) ) ;
#1036=FACE_OUTER_BOUND ( 'NONE', #18183, .T. ) ;
#1037=TOROIDAL_SURFACE ( 'NONE', #14808, 18.46313063346208239, 2.000000000000000000 ) ;
#1038=DIRECTION ( 'NONE',  ( 0.000000000000000000, 0.000000000000000000, 1.000000000000000000 ) ) ;
#1045=ADVANCED_FACE ( 'NONE', ( #24257 ), #7016, .F. ) ;
#1046=ADVANCED_FACE ( 'NONE', ( #26122 ), #416, .T. ) ;
#1050=FACE_OUTER_BOUND ( 'NONE', #10538, .T. ) ;
#1053=DIRECTION ( 'NONE',  ( 0.000000000000000000, -1.000000000000000000, 0.000000000000000000 ) ) ;
#1054=ORIENTED_EDGE ( 'NONE', *, *, #15982, .F. ) ;
#1055=CIRCLE ( 'NONE', #14355, 15.26911010665567225 ) ;
#1058=CARTESIAN_POINT ( 'NONE',  ( -225.3736415174280978, 135.7651958811247539, 14.97905406095859426 ) ) ;
#1061=ORIENTED_EDGE ( 'NONE', *, *, #4761, .T. ) ;
#1062=LINE ( 'NONE', #26784, #6383 ) ;
#1063=VERTEX_POINT ( 'NONE', #2268 ) ;
#1065=CARTESIAN_POINT ( 'NONE',  ( -110.3221550338875687, 20.24192588826927164, 93.88690167569080813 ) ) ;
#1068=ORIENTED_EDGE ( 'NONE', *, *, #27119, .F. ) ;
#1071=CARTESIAN_POINT ( 'NONE',  ( -107.6172385141402259, 133.6752736189426969, 15.67102466709354935 ) ) ;
#1074=VECTOR ( 'NONE', #4601, 1000.000000000000000 ) ;
#1081=AXIS2_PLACEMENT_3D ( 'NONE', #9761, #10179, #23111 ) ;
#1082=CARTESIAN_POINT ( 'NONE',  ( 109.1380356258735134, 251.5976846382455676, 37.70750237629315649 ) ) ;
#1085=CARTESIAN_POINT ( 'NONE',  ( 9.999999999999738876, -50.00000000000004263, 98.28427124746191623 ) ) ;
#1087=CARTESIAN_POINT ( 'NONE',  ( -180.0000000000000000, -40.00000000000004974, -100.0000000000000142 ) ) ;
#1097=CARTESIAN_POINT ( 'NONE',  ( 90.99996269066551235, 240.0000000000000853, -6.657450422703546700 ) ) ;
#1098=DIRECTION ( 'NONE',  ( 1.000000000000000000, 0.000000000000000000, 0.000000000000000000 ) ) ;
#1100=CARTESIAN_POINT ( 'NONE',  ( -76.25760768171836901, 154.8982798170083299, -15.00000000000000000 ) ) ;
#1107=ADVANCED_FACE ( 'NONE', ( #10905 ), #6589, .F. ) ;
#1112=ORIENTED_EDGE ( 'NONE', *, *, #27771, .F. ) ;
#1113=CARTESIAN_POINT ( 'NONE',  ( -137.6741556889342633, 128.9596988076234823, 15.73777296567075901 ) ) ;
#1116=LINE ( 'NONE', #16360, #2392 ) ;
#1117=CARTESIAN_POINT ( 'NONE',  ( -47.64428992525972717, 132.2658675021500301, -15.94853873366968955 ) ) ;
#1123=DIRECTION ( 'NONE',  ( -0.000000000000000000, -0.000000000000000000, 1.000000000000000000 ) ) ;
#1124=FACE_OUTER_BOUND ( 'NONE', #12500, .T. ) ;
#1128=EDGE_CURVE ( 'NONE', #12217, #24673, #907, .T. ) ;
#1130=CARTESIAN_POINT ( 'NONE',  ( -186.0376809321689393, 105.9168515575387062, 32.47349478036296233 ) ) ;
#1136=ORIENTED_EDGE ( 'NONE', *, *, #1662, .T. ) ;
#1141=ORIENTED_EDGE ( 'NONE', *, *, #26039, .F. ) ;
#1143=ADVANCED_FACE ( 'NONE', ( #13642, #22387 ), #8608, .F. ) ;
#1145=EDGE_CURVE ( 'NONE', #3426, #23655, #17362, .T. ) ;
#1146=B_SPLINE_CURVE_WITH_KNOTS ( 'NONE', 3,
 ( #2986, #11778, #20518, #7017, #841, #18510, #9609, #18369, #24975, #11341, #5288, #27256, #7596, #417, #17936, #16878, #3261, #27389, #1643, #3936, #14876, #10412 ),
 .UNSPECIFIED., .F., .F.,
 ( 4, 2, 2, 2, 2, 2, 2, 2, 2, 2, 4 ),
 ( 0.000000000000000000, 0.006705097167734689993, 0.01341019433546937999, 0.01676274291933672195, 0.02011529150320406911, 0.02682038867093874610, 0.03352548583867343002, 0.03687803442254078412, 0.04023058300640813129, 0.04693568017414279786, 0.05364077734187745750 ),
 .UNSPECIFIED. ) ;
#1150=VECTOR ( 'NONE', #20971, 1000.000000000000000 ) ;
#1153=CARTESIAN_POINT ( 'NONE',  ( -21.33210486176665910, 0.000000000000000000, 99.00000000000000000 ) ) ;
#1156=CARTESIAN_POINT ( 'NONE',  ( -219.5652642369064722, 71.26897287455133778, -22.07429503402158488 ) ) ;
#1159=DIRECTION ( 'NONE',  ( 0.000000000000000000, 0.000000000000000000, -1.000000000000000000 ) ) ;
#1162=CARTESIAN_POINT ( 'NONE',  ( 116.8936292565958439, 233.3691281929210959, -99.51164200157825235 ) ) ;
#1164=EDGE_LOOP ( 'NONE', ( #14157, #27836 ) ) ;
#1166=VECTOR ( 'NONE', #3193, 1000.000000000000000 ) ;
#1174=EDGE_CURVE ( 'NONE', #22407, #11012, #9175, .T. ) ;
#1184=ORIENTED_EDGE ( 'NONE', *, *, #2530, .F. ) ;
#1185=CARTESIAN_POINT ( 'NONE',  ( -37.82257053376181233, 36.92584315232891612, 99.00000000000000000 ) ) ;
#1187=AXIS2_PLACEMENT_3D ( 'NONE', #15807, #5001, #8754 ) ;
#1190=AXIS2_PLACEMENT_3D ( 'NONE', #25235, #16624, #25381 ) ;
#1192=CARTESIAN_POINT ( 'NONE',  ( -185.4366074710545433, 106.2948058035834435, -32.30162111875018383 ) ) ;
#1196=DIRECTION ( 'NONE',  ( -0.000000000000000000, 1.000000000000000000, -1.387778780781445429E-16 ) ) ;
#1199=ORIENTED_EDGE ( 'NONE', *, *, #6700, .F. ) ;
#1206=ORIENTED_EDGE ( 'NONE', *, *, #3981, .T. ) ;
#1211=DIRECTION ( 'NONE',  ( 0.000000000000000000, 0.000000000000000000, 1.000000000000000000 ) ) ;
#1214=AXIS2_PLACEMENT_3D ( 'NONE', #8774, #10932, #19691 ) ;
#1219=ADVANCED_FACE ( 'NONE', ( #9748 ), #9363, .T. ) ;
#1222=ORIENTED_EDGE ( 'NONE', *, *, #3961, .F. ) ;
#1225=DIRECTION ( 'NONE',  ( 2.312964634635742464E-16, -1.000000000000000000, 2.139922160430262010E-31 ) ) ;
#1226=FACE_OUTER_BOUND ( 'NONE', #27486, .T. ) ;
#1227=CARTESIAN_POINT ( 'NONE',  ( 90.92319367352099846, 112.0484670279005570, -72.65625000014701129 ) ) ;
#1233=DIRECTION ( 'NONE',  ( 1.000000000000000000, 0.000000000000000000, 0.000000000000000000 ) ) ;
#1236=CARTESIAN_POINT ( 'NONE',  ( -20.04511428896995895, 128.4222523959858222, 17.32321537865083982 ) ) ;
#1239=CYLINDRICAL_SURFACE ( 'NONE', #18735, 49.99999999999998579 ) ;
#1241=EDGE_CURVE ( 'NONE', #27002, #15645, #1541, .T. ) ;
#1244=CARTESIAN_POINT ( 'NONE',  ( 134.9999999999998579, 220.0000000000000284, -84.99999999999997158 ) ) ;
#1249=ADVANCED_FACE ( 'NONE', ( #27949 ), #10306, .F. ) ;
#1250=ORIENTED_EDGE ( 'NONE', *, *, #17544, .T. ) ;
#1252=CARTESIAN_POINT ( 'NONE',  ( 115.1343022193454146, 230.6109841179907960, 98.75454612047967373 ) ) ;
#1254=FACE_OUTER_BOUND ( 'NONE', #3361, .T. ) ;
#1256=VECTOR ( 'NONE', #4847, 1000.000000000000000 ) ;
#1258=CARTESIAN_POINT ( 'NONE',  ( -151.7779492149703913, 124.0884682837862556, -18.38425441931939375 ) ) ;
#1266=CARTESIAN_POINT ( 'NONE',  ( -200.0000000000000284, -91.18033988749901653, 21.20097097723064294 ) ) ;
#1269=CIRCLE ( 'NONE', #23741, 30.00000000000000000 ) ;
#1270=DIRECTION ( 'NONE',  ( 1.000000000000000000, 0.000000000000000000, 0.000000000000000000 ) ) ;
#1271=CARTESIAN_POINT ( 'NONE',  ( -195.0490684805821502, 99.44477443395156513, 32.51470260376371613 ) ) ;
#1272=ORIENTED_EDGE ( 'NONE', *, *, #22671, .T. ) ;
#1275=ADVANCED_FACE ( 'NONE', ( #6416 ), #19630, .F. ) ;
#1277=ORIENTED_EDGE ( 'NONE', *, *, #5268, .T. ) ;
#1281=ORIENTED_EDGE ( 'NONE', *, *, #5887, .F. ) ;
#1285=AXIS2_PLACEMENT_3D ( 'NONE', #5855, #5577, #9897 ) ;
#1286=EDGE_CURVE ( 'NONE', #7257, #11179, #2231, .T. ) ;
#1288=DIRECTION ( 'NONE',  ( 0.000000000000000000, -1.387778780781445429E-16, -1.000000000000000000 ) ) ;
#1289=( BOUNDED_SURFACE ( )  B_SPLINE_SURFACE ( 3, 2, ( 
 ( #15390, #440, #21979 ),
 ( #2576, #8913, #24144 ),
 ( #297, #22269, #11067 ),
 ( #9054, #19823, #17667 ),
 ( #17808, #24277, #22122 ),
 ( #6892, #15673, #24422 ),
 ( #4731, #13516, #11361 ),
 ( #26712, #15822, #1683 ),
 ( #14914, #2101, #26237 ),
 ( #1819, #10451, #6564 ),
 ( #19636, #28098, #10881 ),
 ( #28373, #23668, #15196 ),
 ( #17055, #27954, #8720 ),
 ( #4262, #25670, #12625 ),
 ( #14770, #4117, #8297 ),
 ( #10311, #25812, #13047 ),
 ( #5993, #23809, #8584 ),
 ( #8442, #17473, #12482 ),
 ( #6139, #17198, #3974 ),
 ( #19070, #12761, #21501 ),
 ( #12902, #28240, #15051 ),
 ( #19209, #10593, #19349 ),
 ( #25956, #15342, #21796 ),
 ( #21363, #23523, #3689 ),
 ( #21222, #6277, #21649 ),
 ( #1545, #27815, #8153 ),
 ( #16914, #1959, #3836 ),
 ( #10742, #19496, #17333 ) ),
 .UNSPECIFIED., .F., .F., .F. ) 
 B_SPLINE_SURFACE_WITH_KNOTS ( ( 4, 2, 2, 2, 2, 2, 2, 2, 2, 2, 2, 2, 2, 4 ),
 ( 3, 3 ),
 ( -4.336808689942017736E-19, 0.002390588749581671821, 0.004781177499163344509, 0.007171766248745017197, 0.009562354998326689018, 0.01434353249749003439, 0.01912470999665337804, 0.02151529874623504812, 0.02390588749581672168, 0.02629647624539839523, 0.02868706499498006879, 0.03346824249414341590, 0.03585883124372508945, 0.03824941999330675607 ),
 ( 0.000000000000000000, 1.000000000000000000 ),
 .UNSPECIFIED. ) 
 GEOMETRIC_REPRESENTATION_ITEM ( )  RATIONAL_B_SPLINE_SURFACE ( (
 ( 1.000000000000000000, 0.9597817246759324794, 1.000000000000000000),
 ( 1.000000000000000000, 0.9562412905049657574, 1.000000000000000000),
 ( 1.000000000000000000, 0.9518158024554053132, 1.000000000000000000),
 ( 1.000000000000000000, 0.9416816922015391889, 1.000000000000000000),
 ( 1.000000000000000000, 0.9359714045868776644, 1.000000000000000000),
 ( 1.000000000000000000, 0.9235548114045784018, 1.000000000000000000),
 ( 1.000000000000000000, 0.9168457509165021113, 1.000000000000000000),
 ( 1.000000000000000000, 0.9026276550354167538, 1.000000000000000000),
 ( 1.000000000000000000, 0.8950913600786598590, 1.000000000000000000),
 ( 1.000000000000000000, 0.8718270562173044969, 1.000000000000000000),
 ( 1.000000000000000000, 0.8553941770535198330, 1.000000000000000000),
 ( 1.000000000000000000, 0.8221312774674292001, 1.000000000000000000),
 ( 1.000000000000000000, 0.8052879325280857259, 1.000000000000000000),
 ( 1.000000000000000000, 0.7809787548410676017, 1.000000000000000000),
 ( 1.000000000000000000, 0.7730264403491060587, 1.000000000000000000),
 ( 1.000000000000000000, 0.7580280365901805872, 1.000000000000000000),
 ( 1.000000000000000000, 0.7509406410103288687, 1.000000000000000000),
 ( 1.000000000000000000, 0.7378319876417124279, 1.000000000000000000),
 ( 1.000000000000000000, 0.7318106482057810114, 1.000000000000000000),
 ( 1.000000000000000000, 0.7210845397427231296, 1.000000000000000000),
 ( 1.000000000000000000, 0.7163689906379826500, 1.000000000000000000),
 ( 1.000000000000000000, 0.7048488289897706371, 1.000000000000000000),
 ( 1.000000000000000000, 0.7005414584674227729, 1.000000000000000000),
 ( 1.000000000000000000, 0.6992757048208856352, 1.000000000000000000),
 ( 1.000000000000000000, 0.6997273220235887825, 1.000000000000000000),
 ( 1.000000000000000000, 0.7022627928042818324, 1.000000000000000000),
 ( 1.000000000000000000, 0.7043340258885323335, 1.000000000000000000),
 ( 1.000000000000000000, 0.7071067811865493491, 1.000000000000000000) ) ) 
 REPRESENTATION_ITEM ( '' )  SURFACE ( )  );
#1294=CARTESIAN_POINT ( 'NONE',  ( -194.3369914945607491, 63.17511408073718826, -42.65718952139617670 ) ) ;
#1295=EDGE_CURVE ( 'NONE', #18743, #15118, #13304, .T. ) ;
#1300=FACE_OUTER_BOUND ( 'NONE', #3508, .T. ) ;
#1304=AXIS2_PLACEMENT_3D ( 'NONE', #14317, #27788, #3096 ) ;
#1305=AXIS2_PLACEMENT_3D ( 'NONE', #15444, #19733, #490 ) ;
#1306=FACE_OUTER_BOUND ( 'NONE', #8945, .T. ) ;
#1309=ORIENTED_EDGE ( 'NONE', *, *, #3636, .T. ) ;
#1311=CARTESIAN_POINT ( 'NONE',  ( 100.8904249506254018, 86.57652225510716448, 100.0000000000000142 ) ) ;
#1315=CARTESIAN_POINT ( 'NONE',  ( -175.0000000000000000, -150.0000000000000853, 70.00000000000001421 ) ) ;
#1316=DIRECTION ( 'NONE',  ( 1.000000000000000000, 0.000000000000000000, 0.000000000000000000 ) ) ;
#1321=CARTESIAN_POINT ( 'NONE',  ( 96.76194576697650973, 83.89264379418858653, 100.0000000000000142 ) ) ;
#1323=DIRECTION ( 'NONE',  ( -1.000000000000000000, 0.000000000000000000, 0.000000000000000000 ) ) ;
#1324=AXIS2_PLACEMENT_3D ( 'NONE', #25707, #23704, #14811 ) ;
#1326=CARTESIAN_POINT ( 'NONE',  ( 6.071532165918828775E-15, -70.00000000000002842, 25.00000000000000000 ) ) ;
#1331=LINE ( 'NONE', #16710, #7843 ) ;
#1333=VERTEX_POINT ( 'NONE', #6835 ) ;
#1335=DIRECTION ( 'NONE',  ( 0.000000000000000000, 0.000000000000000000, -1.000000000000000000 ) ) ;
#1342=VERTEX_POINT ( 'NONE', #15617 ) ;
#1343=CIRCLE ( 'NONE', #4083, 70.83858790703926900 ) ;
#1344=CARTESIAN_POINT ( 'NONE',  ( -173.6192398023450494, 113.7611339081862667, 27.04214115208617031 ) ) ;
#1346=FACE_OUTER_BOUND ( 'NONE', #4307, .T. ) ;
#1348=CARTESIAN_POINT ( 'NONE',  ( -37.82257053376181233, 71.03850157808263077, 100.0000000000000000 ) ) ;
#1352=AXIS2_PLACEMENT_3D ( 'NONE', #2714, #11503, #20243 ) ;
#1354=CARTESIAN_POINT ( 'NONE',  ( 109.9999999999998721, 259.8688628429572987, 44.77286377382201010 ) ) ;
#1357=AXIS2_PLACEMENT_3D ( 'NONE', #25698, #14796, #12504 ) ;
#1358=CARTESIAN_POINT ( 'NONE',  ( 22.58950924271108107, 154.2349915562422495, -15.00000000000000000 ) ) ;
#1359=ORIENTED_EDGE ( 'NONE', *, *, #25587, .T. ) ;
#1362=VERTEX_POINT ( 'NONE', #24090 ) ;
#1364=CIRCLE ( 'NONE', #18795, 9.999999999999994671 ) ;
#1369=CIRCLE ( 'NONE', #17420, 11.00000000000001066 ) ;
#1372=LINE ( 'NONE', #25920, #24620 ) ;
#1374=CARTESIAN_POINT ( 'NONE',  ( 9.999999999999749534, 90.00000000000001421, 98.28427124746191623 ) ) ;
#1376=DIRECTION ( 'NONE',  ( -1.000000000000000000, 0.000000000000000000, 0.000000000000000000 ) ) ;
#1381=CARTESIAN_POINT ( 'NONE',  ( 102.1958639858411004, 244.1335791876568919, -16.70126253799778482 ) ) ;
#1383=DIRECTION ( 'NONE',  ( -0.000000000000000000, -0.000000000000000000, -1.000000000000000000 ) ) ;
#1390=VERTEX_POINT ( 'NONE', #8577 ) ;
#1391=CARTESIAN_POINT ( 'NONE',  ( -75.10678314939089262, 136.1130475173332570, 15.20604832699645392 ) ) ;
#1393=VERTEX_POINT ( 'NONE', #17329 ) ;
#1394=CARTESIAN_POINT ( 'NONE',  ( -71.37541315349507443, 240.0000000000000000, -5.000000000000004441 ) ) ;
#1395=CARTESIAN_POINT ( 'NONE',  ( 79.99999999999990052, 140.0000000000000000, 45.00000000000000000 ) ) ;
#1396=DIRECTION ( 'NONE',  ( 0.000000000000000000, -1.000000000000000000, 0.000000000000000000 ) ) ;
#1397=CARTESIAN_POINT ( 'NONE',  ( -135.1444269713557560, 129.7101293712805443, -15.41478258222857001 ) ) ;
#1402=VECTOR ( 'NONE', #9107, 1000.000000000000000 ) ;
#1404=LINE ( 'NONE', #18932, #21349 ) ;
#1408=ORIENTED_EDGE ( 'NONE', *, *, #26865, .F. ) ;
#1409=VECTOR ( 'NONE', #10667, 1000.000000000000000 ) ;
#1412=ORIENTED_EDGE ( 'NONE', *, *, #24891, .T. ) ;
#1415=DIRECTION ( 'NONE',  ( 0.000000000000000000, 1.000000000000000000, 0.000000000000000000 ) ) ;
#1419=VECTOR ( 'NONE', #18095, 1000.000000000000000 ) ;
#1422=EDGE_LOOP ( 'NONE', ( #15865, #11931 ) ) ;
#1430=DIRECTION ( 'NONE',  ( 0.000000000000000000, -1.000000000000000000, 0.000000000000000000 ) ) ;
#1435=PLANE ( 'NONE',  #17938 ) ;
#1439=LINE ( 'NONE', #20844, #20621 ) ;
#1440=VECTOR ( 'NONE', #10465, 1000.000000000000000 ) ;
#1442=EDGE_CURVE ( 'NONE', #13173, #17645, #9851, .T. ) ;
#1443=CARTESIAN_POINT ( 'NONE',  ( -40.40953891503691153, 36.92584315232891612, 99.00000000000000000 ) ) ;
#1447=ORIENTED_EDGE ( 'NONE', *, *, #1879, .F. ) ;
#1448=CARTESIAN_POINT ( 'NONE',  ( 90.92319367350451387, 112.0484670279762440, 100.0000000000108429 ) ) ;
#1450=ORIENTED_EDGE ( 'NONE', *, *, #24142, .F. ) ;
#1451=EDGE_LOOP ( 'NONE', ( #18837, #7191, #7969 ) ) ;
#1457=CARTESIAN_POINT ( 'NONE',  ( -180.5998324953250176, 109.6502091928870328, -29.97430207196073937 ) ) ;
#1460=VERTEX_POINT ( 'NONE', #9437 ) ;
#1463=CARTESIAN_POINT ( 'NONE',  ( -68.57415822541635464, 29.64876300893806516, 95.00000000000000000 ) ) ;
#1467=PLANE ( 'NONE',  #6625 ) ;
#1476=CYLINDRICAL_SURFACE ( 'NONE', #6613, 5.999999999999991118 ) ;
#1479=DIRECTION ( 'NONE',  ( 1.000000000000000000, -0.000000000000000000, -0.000000000000000000 ) ) ;
#1481=CIRCLE ( 'NONE', #11600, 16.07743405327025243 ) ;
#1482=CARTESIAN_POINT ( 'NONE',  ( -191.5126735617889437, 102.3039448627891659, 32.04604572034998711 ) ) ;
#1491=LINE ( 'NONE', #19440, #19816 ) ;
#1492=CARTESIAN_POINT ( 'NONE',  ( 109.9579984081460680, 258.6776769496694897, 42.70939860559244750 ) ) ;
#1493=VERTEX_POINT ( 'NONE', #18474 ) ;
#1497=EDGE_LOOP ( 'NONE', ( #15130, #928, #10438, #25905 ) ) ;
#1501=ADVANCED_FACE ( 'NONE', ( #26947 ), #11741, .F. ) ;
#1504=ADVANCED_FACE ( 'NONE', ( #27224 ), #17208, .T. ) ;
#1510=CARTESIAN_POINT ( 'NONE',  ( -237.0233935005625483, 68.72940251376158471, -14.95240471282613193 ) ) ;
#1514=CARTESIAN_POINT ( 'NONE',  ( 112.5174913703661446, 218.9750123000742121, -96.63436734148044138 ) ) ;
#1515=VERTEX_POINT ( 'NONE', #3229 ) ;
#1518=CARTESIAN_POINT ( 'NONE',  ( 12.09558415809990883, 89.94522053857441790, 98.30381960812032105 ) ) ;
#1519=CARTESIAN_POINT ( 'NONE',  ( -160.0000000000000284, 59.99999999999994316, 100.0000000000000142 ) ) ;
#1520=DIRECTION ( 'NONE',  ( -1.850371707708594316E-16, 1.000000000000000000, 0.000000000000000000 ) ) ;
#1523=CIRCLE ( 'NONE', #17573, 1.000000000000000888 ) ;
#1524=CARTESIAN_POINT ( 'NONE',  ( -17.24491960465745777, -18.01420295945611727, 95.00000000000000000 ) ) ;
#1527=DIRECTION ( 'NONE',  ( 1.000000000000000000, -0.000000000000000000, -0.000000000000000000 ) ) ;
#1532=EDGE_LOOP ( 'NONE', ( #1222, #7249, #21467, #6614 ) ) ;
#1535=CARTESIAN_POINT ( 'NONE',  ( 112.5712424644273426, 217.9445819143301435, 96.69730840357098600 ) ) ;
#1536=CARTESIAN_POINT ( 'NONE',  ( -157.8051893169759126, 120.7082176335777177, -21.99009546054191944 ) ) ;
#1538=EDGE_CURVE ( 'NONE', #13911, #7659, #15377, .T. ) ;
#1541=LINE ( 'NONE', #19065, #27950 ) ;
#1544=CARTESIAN_POINT ( 'NONE',  ( 24.17452580132986739, -46.52307359567973322, 99.29556765389919804 ) ) ;
#1545=CARTESIAN_POINT ( 'NONE',  ( -232.1637141486664575, 91.03144149473433799, -15.02585134956874668 ) ) ;
#1549=CARTESIAN_POINT ( 'NONE',  ( -232.1720359504865883, 90.98239771430922929, 14.99999999999994849 ) ) ;
#1552=DIRECTION ( 'NONE',  ( 0.000000000000000000, 0.000000000000000000, 1.000000000000000000 ) ) ;
#1559=CARTESIAN_POINT ( 'NONE',  ( 98.16608178754364644, 241.2913188899317163, -20.91842009986573814 ) ) ;
#1563=EDGE_CURVE ( 'NONE', #10183, #19021, #8058, .T. ) ;
#1564=EDGE_CURVE ( 'NONE', #18588, #18031, #10134, .T. ) ;
#1569=DIRECTION ( 'NONE',  ( -0.7348549764921098459, 0.6782242722910915012, 4.000673683678708817E-14 ) ) ;
#1572=CARTESIAN_POINT ( 'NONE',  ( -225.7036482868739427, -91.18033988749901653, 0.000000000000000000 ) ) ;
#1577=CARTESIAN_POINT ( 'NONE',  ( -216.5430934856041745, 71.49318776575898937, -24.90892144430478794 ) ) ;
#1582=DIRECTION ( 'NONE',  ( -0.000000000000000000, -0.000000000000000000, -1.000000000000000000 ) ) ;
#1586=FACE_OUTER_BOUND ( 'NONE', #20704, .T. ) ;
#1588=ORIENTED_EDGE ( 'NONE', *, *, #16351, .F. ) ;
#1595=CIRCLE ( 'NONE', #25913, 30.00000000000000000 ) ;
#1601=CARTESIAN_POINT ( 'NONE',  ( 95.20156243614241021, 83.09913198708241566, 100.0000000000000142 ) ) ;
#1604=FACE_OUTER_BOUND ( 'NONE', #3933, .T. ) ;
#1607=DIRECTION ( 'NONE',  ( 1.000000000000000000, 0.000000000000000000, 0.000000000000000000 ) ) ;
#1609=DIRECTION ( 'NONE',  ( -0.7082136108520787898, -0.7059982162894324897, -0.000000000000000000 ) ) ;
#1616=EDGE_LOOP ( 'NONE', ( #18989, #23428, #19375, #25548 ) ) ;
#1617=AXIS2_PLACEMENT_3D ( 'NONE', #5431, #16231, #11784 ) ;
#1618=EDGE_CURVE ( 'NONE', #16979, #5099, #5678, .T. ) ;
#1619=LINE ( 'NONE', #23740, #6834 ) ;
#1622=DIRECTION ( 'NONE',  ( 1.000000000000000000, 0.000000000000000000, 0.000000000000000000 ) ) ;
#1624=ORIENTED_EDGE ( 'NONE', *, *, #10974, .T. ) ;
#1634=ORIENTED_EDGE ( 'NONE', *, *, #22159, .T. ) ;
#1635=AXIS2_PLACEMENT_3D ( 'NONE', #16913, #25532, #23808 ) ;
#1641=EDGE_CURVE ( 'NONE', #5984, #20120, #8115, .T. ) ;
#1643=CARTESIAN_POINT ( 'NONE',  ( 0.6945804017089570737, 136.6086003902396158, 13.39232072666088769 ) ) ;
#1647=CARTESIAN_POINT ( 'NONE',  ( -232.3018049223840364, 76.77033509348976281, -15.55816966298101178 ) ) ;
#1649=DIRECTION ( 'NONE',  ( 1.000000000000000000, 0.000000000000000000, 0.000000000000000000 ) ) ;
#1651=CARTESIAN_POINT ( 'NONE',  ( -248.1546605714623013, -91.18033988749901653, 16.91094714394370158 ) ) ;
#1654=EDGE_CURVE ( 'NONE', #3789, #4321, #7583, .T. ) ;
#1657=CARTESIAN_POINT ( 'NONE',  ( 96.24933711586670881, 240.9969687801728639, -9.998578604269592773 ) ) ;
#1658=DIRECTION ( 'NONE',  ( -0.000000000000000000, -0.000000000000000000, 1.000000000000000000 ) ) ;
#1661=VECTOR ( 'NONE', #17745, 1000.000000000000000 ) ;
#1662=EDGE_CURVE ( 'NONE', #14427, #8519, #11250, .T. ) ;
#1667=ORIENTED_EDGE ( 'NONE', *, *, #9784, .T. ) ;
#1669=VECTOR ( 'NONE', #26953, 1000.000000000000000 ) ;
#1673=EDGE_LOOP ( 'NONE', ( #5843, #13373 ) ) ;
#1675=FACE_BOUND ( 'NONE', #2044, .T. ) ;
#1677=CARTESIAN_POINT ( 'NONE',  ( -158.6398931503276515, 121.2395900921240610, -20.46722486591957946 ) ) ;
#1678=ADVANCED_FACE ( 'NONE', ( #28054 ), #10553, .F. ) ;
#1679=AXIS2_PLACEMENT_3D ( 'NONE', #10968, #21595, #28047 ) ;
#1680=LINE ( 'NONE', #10448, #20191 ) ;
#1682=CARTESIAN_POINT ( 'NONE',  ( 31.66302550918311809, -40.78000118157726916, 100.0000000000000000 ) ) ;
#1683=CARTESIAN_POINT ( 'NONE',  ( -208.4928213732883080, 89.66777255638292843, -24.75805542544560112 ) ) ;
#1689=ORIENTED_EDGE ( 'NONE', *, *, #11782, .T. ) ;
#1691=LINE ( 'NONE', #13060, #21313 ) ;
#1693=ORIENTED_EDGE ( 'NONE', *, *, #14822, .F. ) ;
#1695=EDGE_CURVE ( 'NONE', #7257, #2661, #23650, .T. ) ;
#1697=CARTESIAN_POINT ( 'NONE',  ( 93.32984351717588822, 231.0185867901169274, -18.11991709984777188 ) ) ;
#1699=ORIENTED_EDGE ( 'NONE', *, *, #2899, .F. ) ;
#1708=CARTESIAN_POINT ( 'NONE',  ( -138.6428522700808230, 71.54464929955099706, 80.00000000000001421 ) ) ;
#1711=DIRECTION ( 'NONE',  ( -1.000000000000000000, 0.000000000000000000, 0.000000000000000000 ) ) ;
#1712=TOROIDAL_SURFACE ( 'NONE', #9993, 21.49999999999998224, 1.000000000000000000 ) ;
#1714=AXIS2_PLACEMENT_3D ( 'NONE', #13179, #26225, #17323 ) ;
#1716=DIRECTION ( 'NONE',  ( 0.000000000000000000, 0.000000000000000000, 1.000000000000000000 ) ) ;
#1718=CARTESIAN_POINT ( 'NONE',  ( 134.9999999999998579, 220.0000000000000284, -99.00000000000001421 ) ) ;
#1720=CARTESIAN_POINT ( 'NONE',  ( -201.6083822205884815, 94.40621216759335255, 29.51015678107877349 ) ) ;
#1721=EDGE_CURVE ( 'NONE', #21449, #20037, #4217, .T. ) ;
#1725=VERTEX_POINT ( 'NONE', #15440 ) ;
#1728=CARTESIAN_POINT ( 'NONE',  ( 118.4313905926795769, 122.3304618272157285, 100.0000000000000142 ) ) ;
#1730=AXIS2_PLACEMENT_3D ( 'NONE', #10382, #16986, #5648 ) ;
#1731=ORIENTED_EDGE ( 'NONE', *, *, #27128, .T. ) ;
#1733=CARTESIAN_POINT ( 'NONE',  ( 109.5756401952514523, 134.3783162855169451, -89.68749999975639753 ) ) ;
#1735=CARTESIAN_POINT ( 'NONE',  ( -196.6111576902316358, 98.46805465545536151, -31.30665360858167645 ) ) ;
#1737=CARTESIAN_POINT ( 'NONE',  ( -233.2943309833551382, 92.06151970357234404, 15.00000000000000000 ) ) ;
#1745=ADVANCED_FACE ( 'NONE', ( #25909 ), #8958, .T. ) ;
#1750=CARTESIAN_POINT ( 'NONE',  ( 109.9999999999999574, -120.0000000000000568, -25.00000000000000711 ) ) ;
#1752=VERTEX_POINT ( 'NONE', #17155 ) ;
#1753=CARTESIAN_POINT ( 'NONE',  ( 119.1248245724174524, 235.9877291319237429, 100.0000000000000142 ) ) ;
#1756=CARTESIAN_POINT ( 'NONE',  ( -203.1779787704217313, 93.05164332230201296, 28.77272332722132120 ) ) ;
#1764=CARTESIAN_POINT ( 'NONE',  ( -173.2914958970121404, 113.9438874222513789, -27.61821649288708969 ) ) ;
#1766=ORIENTED_EDGE ( 'NONE', *, *, #18746, .T. ) ;
#1767=DIRECTION ( 'NONE',  ( 0.000000000000000000, 0.000000000000000000, -1.000000000000000000 ) ) ;
#1768=ORIENTED_EDGE ( 'NONE', *, *, #2402, .T. ) ;
#1773=EDGE_CURVE ( 'NONE', #3789, #4186, #11736, .T. ) ;
#1777=DIRECTION ( 'NONE',  ( 0.000000000000000000, 0.000000000000000000, -1.000000000000000000 ) ) ;
#1780=CARTESIAN_POINT ( 'NONE',  ( -231.9024517383451212, 76.40908368390745409, -15.65418338381065944 ) ) ;
#1784=CIRCLE ( 'NONE', #24289, 6.000000000000005329 ) ;
#1785=CARTESIAN_POINT ( 'NONE',  ( -217.2892621185082760, 109.4029876883478352, -15.00000000000000000 ) ) ;
#1799=VERTEX_POINT ( 'NONE', #22029 ) ;
#1802=ORIENTED_EDGE ( 'NONE', *, *, #22126, .T. ) ;
#1803=ORIENTED_EDGE ( 'NONE', *, *, #23982, .T. ) ;
#1804=CARTESIAN_POINT ( 'NONE',  ( -140.1213116003368668, 122.5384136796733827, -15.00000000000000000 ) ) ;
#1808=VERTEX_POINT ( 'NONE', #19593 ) ;
#1809=CARTESIAN_POINT ( 'NONE',  ( 0.000000000000000000, 0.000000000000000000, 100.0000000000000000 ) ) ;
#1811=CARTESIAN_POINT ( 'NONE',  ( -97.59841077035456181, 134.4761401613473879, -15.51281503506764814 ) ) ;
#1814=EDGE_CURVE ( 'NONE', #1940, #20107, #4489, .T. ) ;
#1815=CARTESIAN_POINT ( 'NONE',  ( -142.1390311221107368, 127.5729955578239156, -17.65724288274918763 ) ) ;
#1816=AXIS2_PLACEMENT_3D ( 'NONE', #8716, #6696, #21924 ) ;
#1819=CARTESIAN_POINT ( 'NONE',  ( -211.3790541256307733, 87.57060272315374050, -24.25130854840332617 ) ) ;
#1822=EDGE_CURVE ( 'NONE', #24930, #20966, #20446, .T. ) ;
#1824=CARTESIAN_POINT ( 'NONE',  ( -160.0000000000000284, 59.99999999999994316, -15.00000000000000000 ) ) ;
#1826=ORIENTED_EDGE ( 'NONE', *, *, #5486, .F. ) ;
#1832=ORIENTED_EDGE ( 'NONE', *, *, #12580, .T. ) ;
#1834=CARTESIAN_POINT ( 'NONE',  ( 103.7569845406462861, 245.1294976011695894, -26.47883977339530759 ) ) ;
#1842=AXIS2_PLACEMENT_3D ( 'NONE', #7567, #9854, #18200 ) ;
#1843=DIRECTION ( 'NONE',  ( 0.000000000000000000, 0.000000000000000000, -1.000000000000000000 ) ) ;
#1848=LINE ( 'NONE', #17364, #5052 ) ;
#1852=CARTESIAN_POINT ( 'NONE',  ( -31.50759449548381497, 129.2243747201668214, 15.65997819548621628 ) ) ;
#1853=B_SPLINE_CURVE_WITH_KNOTS ( 'NONE', 3,
 ( #989, #3273, #3419, #18524, #719, #24846, #7468, #9765, #853, #14083, #12213, #20814, #11927, #20952, #14499, #22833, #3558, #16097, #27268, #5722, #20528, #7609 ),
 .UNSPECIFIED., .F., .F.,
 ( 4, 2, 2, 2, 2, 2, 2, 2, 2, 2, 4 ),
 ( 0.000000000000000000, 0.1249999999999999306, 0.2500000000000000555, 0.3750000000000000000, 0.5000000000000000000, 0.6250000000000000000, 0.7500000000000000000, 0.8125000000000000000, 0.8750000000000001110, 0.9374999999999998890, 1.000000000000000000 ),
 .UNSPECIFIED. ) ;
#1854=DIRECTION ( 'NONE',  ( 0.000000000000000000, 0.000000000000000000, 1.000000000000000000 ) ) ;
#1855=DIRECTION ( 'NONE',  ( 0.000000000000000000, -1.387778780781445429E-16, -1.000000000000000000 ) ) ;
#1856=CARTESIAN_POINT ( 'NONE',  ( 65.00000000000000000, -150.0000000000000568, 76.00000000000001421 ) ) ;
#1858=CARTESIAN_POINT ( 'NONE',  ( 119.9999999999998863, 330.0000000000000000, 90.00000000000002842 ) ) ;
#1861=ORIENTED_EDGE ( 'NONE', *, *, #10332, .T. ) ;
#1863=ORIENTED_EDGE ( 'NONE', *, *, #6822, .T. ) ;
#1866=CARTESIAN_POINT ( 'NONE',  ( 81.45493510947169113, 110.0000000031298981, 100.0000000000000142 ) ) ;
#1871=CARTESIAN_POINT ( 'NONE',  ( 96.76194576697405125, 83.89264379418708018, -100.0000000000000284 ) ) ;
#1876=CARTESIAN_POINT ( 'NONE',  ( -227.8046702420875533, 90.53362311475710555, 13.46331733193806102 ) ) ;
#1878=CARTESIAN_POINT ( 'NONE',  ( -46.68942599940377391, -18.01420295945611727, 100.0000000000000000 ) ) ;
#1879=EDGE_CURVE ( 'NONE', #16598, #25488, #13714, .T. ) ;
#1889=DIRECTION ( 'NONE',  ( 1.000000000000000000, 0.000000000000000000, -0.000000000000000000 ) ) ;
#1895=FACE_OUTER_BOUND ( 'NONE', #25198, .T. ) ;
#1896=CARTESIAN_POINT ( 'NONE',  ( -17.24491960465745777, -18.01420295945611727, 95.00000000000000000 ) ) ;
#1903=DIRECTION ( 'NONE',  ( 0.000000000000000000, 0.000000000000000000, 1.000000000000000000 ) ) ;
#1904=CARTESIAN_POINT ( 'NONE',  ( -188.5440957081713407, 104.2034936733272161, -32.76882375805663372 ) ) ;
#1907=AXIS2_PLACEMENT_3D ( 'NONE', #13162, #26068, #19181 ) ;
#1909=CARTESIAN_POINT ( 'NONE',  ( -110.7275636018716654, 68.51688903468615877, 83.00000000000001421 ) ) ;
#1910=ORIENTED_EDGE ( 'NONE', *, *, #5300, .F. ) ;
#1912=ORIENTED_EDGE ( 'NONE', *, *, #259, .F. ) ;
#1913=VERTEX_POINT ( 'NONE', #17861 ) ;
#1914=FACE_OUTER_BOUND ( 'NONE', #10500, .T. ) ;
#1919=CARTESIAN_POINT ( 'NONE',  ( -207.7359966080777554, 74.87654876227064449, -43.86827885981523423 ) ) ;
#1921=CARTESIAN_POINT ( 'NONE',  ( -226.6109647993037868, 62.69877383611189003, -18.44381613004360432 ) ) ;
#1924=FACE_OUTER_BOUND ( 'NONE', #19298, .T. ) ;
#1927=DIRECTION ( 'NONE',  ( -0.000000000000000000, -1.000000000000000000, -0.000000000000000000 ) ) ;
#1930=ORIENTED_EDGE ( 'NONE', *, *, #21678, .T. ) ;
#1931=CARTESIAN_POINT ( 'NONE',  ( -86.45101491668415861, -42.20485572845630884, -15.00000000000000000 ) ) ;
#1936=LINE ( 'NONE', #8836, #19345 ) ;
#1939=DIRECTION ( 'NONE',  ( 0.000000000000000000, 0.000000000000000000, -1.000000000000000000 ) ) ;
#1940=VERTEX_POINT ( 'NONE', #771 ) ;
#1941=CARTESIAN_POINT ( 'NONE',  ( 112.4999999999998863, 220.0000000000000284, -90.00000000000002842 ) ) ;
#1944=CARTESIAN_POINT ( 'NONE',  ( 112.4999999999998863, 220.0000000000000284, 90.00000000000002842 ) ) ;
#1946=EDGE_CURVE ( 'NONE', #15640, #16689, #12202, .T. ) ;
#1947=CIRCLE ( 'NONE', #20308, 5.000000000000004441 ) ;
#1948=EDGE_LOOP ( 'NONE', ( #12224, #23472, #16271, #17867 ) ) ;
#1950=VECTOR ( 'NONE', #12093, 1000.000000000000227 ) ;
#1951=DIRECTION ( 'NONE',  ( 0.000000000000000000, 0.000000000000000000, 1.000000000000000000 ) ) ;
#1959=CARTESIAN_POINT ( 'NONE',  ( -231.4227546898554522, 93.05579960084709512, -15.01574783250532974 ) ) ;
#1966=DIRECTION ( 'NONE',  ( 1.000000000000000000, 0.000000000000000000, 0.000000000000000000 ) ) ;
#1967=ORIENTED_EDGE ( 'NONE', *, *, #9632, .T. ) ;
#1969=AXIS2_PLACEMENT_3D ( 'NONE', #5932, #12840, #14856 ) ;
#1971=DIRECTION ( 'NONE',  ( 0.000000000000000000, 0.000000000000000000, 1.000000000000000000 ) ) ;
#1973=VECTOR ( 'NONE', #25367, 1000.000000000000000 ) ;
#1978=CARTESIAN_POINT ( 'NONE',  ( 94.04374108504291030, 240.3974664687522420, -8.346404539541740775 ) ) ;
#1980=DIRECTION ( 'NONE',  ( 1.000000000000000000, -0.000000000000000000, -0.000000000000000000 ) ) ;
#1992=DIRECTION ( 'NONE',  ( 1.000000000000000000, -0.000000000000000000, -0.000000000000000000 ) ) ;
#1995=LINE ( 'NONE', #1326, #26382 ) ;
#1997=LINE ( 'NONE', #4574, #7104 ) ;
#2000=CARTESIAN_POINT ( 'NONE',  ( -23.49204859636672893, 128.1179884427479294, 17.45313152111423705 ) ) ;
#2001=DIRECTION ( 'NONE',  ( 1.000000000000000000, 0.000000000000000000, 0.000000000000000000 ) ) ;
#2004=ORIENTED_EDGE ( 'NONE', *, *, #27343, .T. ) ;
#2005=VERTEX_POINT ( 'NONE', #9677 ) ;
#2007=CARTESIAN_POINT ( 'NONE',  ( -173.0260071355321543, 113.6300340977356029, 28.16161390424484878 ) ) ;
#2008=DIRECTION ( 'NONE',  ( 1.000000000000000000, 0.000000000000000000, 0.000000000000000000 ) ) ;
#2009=VERTEX_POINT ( 'NONE', #7382 ) ;
#2012=VERTEX_POINT ( 'NONE', #18437 ) ;
#2016=CARTESIAN_POINT ( 'NONE',  ( 134.9999999999998579, 220.0000000000000284, -84.99999999999997158 ) ) ;
#2021=CARTESIAN_POINT ( 'NONE',  ( 98.15430812627619162, 116.0637945822588364, -100.0000000000433005 ) ) ;
#2024=CARTESIAN_POINT ( 'NONE',  ( -169.9623962693859482, 115.7491617292054826, -25.38483726571820753 ) ) ;
#2026=CARTESIAN_POINT ( 'NONE',  ( -224.4716126166392485, 89.01384884033475942, 16.47823558538952682 ) ) ;
#2027=EDGE_LOOP ( 'NONE', ( #9558, #1359, #12496, #26792 ) ) ;
#2030=CARTESIAN_POINT ( 'NONE',  ( -146.6428522700808230, 69.54464929955099706, 80.00000000000001421 ) ) ;
#2035=CARTESIAN_POINT ( 'NONE',  ( 115.9304285313496905, 208.0449276593521688, 99.14012769162644645 ) ) ;
#2038=DIRECTION ( 'NONE',  ( 0.000000000000000000, 0.000000000000000000, 1.000000000000000000 ) ) ;
#2040=CARTESIAN_POINT ( 'NONE',  ( 9.345921402568901470, 140.0000000000000000, 15.00000000000000000 ) ) ;
#2042=DIRECTION ( 'NONE',  ( -1.000000000000000000, 6.938893903907227392E-16, 0.000000000000000000 ) ) ;
#2043=CARTESIAN_POINT ( 'NONE',  ( -40.40953891503691153, 71.03850157808263077, 100.0000000000000000 ) ) ;
#2044=EDGE_LOOP ( 'NONE', ( #13113, #23691 ) ) ;
#2046=ORIENTED_EDGE ( 'NONE', *, *, #15839, .T. ) ;
#2049=EDGE_CURVE ( 'NONE', #88, #24530, #1995, .T. ) ;
#2050=CARTESIAN_POINT ( 'NONE',  ( -185.8938050120760295, 106.2234131628355414, -31.95887621392303046 ) ) ;
#2055=ORIENTED_EDGE ( 'NONE', *, *, #22306, .F. ) ;
#2056=CARTESIAN_POINT ( 'NONE',  ( -146.6428522700808230, 17.24192588826928585, 83.00000000000001421 ) ) ;
#2057=ORIENTED_EDGE ( 'NONE', *, *, #18923, .T. ) ;
#2060=CARTESIAN_POINT ( 'NONE',  ( 93.99999999999985789, 268.4896896257338312, -105.0000000000000284 ) ) ;
#2063=CIRCLE ( 'NONE', #16327, 5.999999999999991118 ) ;
#2066=CARTESIAN_POINT ( 'NONE',  ( -229.4479296852199752, 74.49644851801838286, -16.38316105114333965 ) ) ;
#2069=CIRCLE ( 'NONE', #264, 10.00000000000000888 ) ;
#2070=DIRECTION ( 'NONE',  ( 1.000000000000000000, 0.000000000000000000, 0.000000000000000000 ) ) ;
#2071=CARTESIAN_POINT ( 'NONE',  ( -2.081668171172168513E-14, 79.99999999999998579, -100.0000000000000142 ) ) ;
#2082=EDGE_CURVE ( 'NONE', #24246, #19138, #25959, .T. ) ;
#2083=DIRECTION ( 'NONE',  ( 1.000000000000000000, 0.000000000000000000, 0.000000000000000000 ) ) ;
#2090=DIRECTION ( 'NONE',  ( -0.000000000000000000, 0.000000000000000000, -1.000000000000000000 ) ) ;
#2092=CIRCLE ( 'NONE', #3938, 5.000000000000004441 ) ;
#2094=CARTESIAN_POINT ( 'NONE',  ( -223.0199379110806035, 134.9200334684876168, 15.12837422688625644 ) ) ;
#2095=CARTESIAN_POINT ( 'NONE',  ( -136.8324479085035250, 127.9412362963770704, -17.51947590493717044 ) ) ;
#2100=DIRECTION ( 'NONE',  ( 1.541976423090495387E-16, -1.000000000000000000, 0.000000000000000000 ) ) ;
#2101=CARTESIAN_POINT ( 'NONE',  ( -209.5896013737285273, 89.20569115677373873, -25.08817329724644551 ) ) ;
#2103=AXIS2_PLACEMENT_3D ( 'NONE', #3755, #21143, #12265 ) ;
#2106=DIRECTION ( 'NONE',  ( 1.000000000000000000, 0.000000000000000000, 0.000000000000000000 ) ) ;
#2108=CARTESIAN_POINT ( 'NONE',  ( 139.9999999999999716, -100.0000000000000000, 70.00000000000001421 ) ) ;
#2116=ORIENTED_EDGE ( 'NONE', *, *, #5364, .T. ) ;
#2118=CARTESIAN_POINT ( 'NONE',  ( 87.50000000000012790, 240.0000000000000000, -15.95262490344442874 ) ) ;
#2120=EDGE_CURVE ( 'NONE', #4808, #25545, #12669, .T. ) ;
#2126=EDGE_LOOP ( 'NONE', ( #10887, #1967, #16409, #23505 ) ) ;
#2129=DIRECTION ( 'NONE',  ( -0.000000000000000000, 1.000000000000000000, -1.387778780781445429E-16 ) ) ;
#2133=CARTESIAN_POINT ( 'NONE',  ( -216.3679220181659275, 71.52319660855000905, 25.09443459582798042 ) ) ;
#2135=CARTESIAN_POINT ( 'NONE',  ( -17.24491960465745777, -18.01420295945611727, 100.0000000000000000 ) ) ;
#2137=CARTESIAN_POINT ( 'NONE',  ( -143.2374437020967264, 68.51688903468615877, 83.00000000000001421 ) ) ;
#2139=CARTESIAN_POINT ( 'NONE',  ( -223.7930071774131022, 71.88803283280797984, -19.06147322994570459 ) ) ;
#2142=CARTESIAN_POINT ( 'NONE',  ( -207.5044420441007560, 75.59897387903042443, 45.00000000000000000 ) ) ;
#2144=DIRECTION ( 'NONE',  ( -0.000000000000000000, 1.000000000000000000, -1.387778780781445429E-16 ) ) ;
#2148=CARTESIAN_POINT ( 'NONE',  ( -164.5564299301625226, 118.4912152583887490, 22.95374496050424895 ) ) ;
#2153=EDGE_LOOP ( 'NONE', ( #18531, #17494, #11357, #20141 ) ) ;
#2155=EDGE_CURVE ( 'NONE', #25901, #13173, #28242, .T. ) ;
#2156=CARTESIAN_POINT ( 'NONE',  ( -219.9082363642617679, 137.1815813412194700, -12.98324324876687363 ) ) ;
#2159=CARTESIAN_POINT ( 'NONE',  ( 91.70829090828171104, 81.72138244998292578, -100.0000000000000284 ) ) ;
#2160=LINE ( 'NONE', #10939, #20589 ) ;
#2162=CARTESIAN_POINT ( 'NONE',  ( -214.4302377132927404, 86.70854347113640870, 22.08344159346780344 ) ) ;
#2168=CARTESIAN_POINT ( 'NONE',  ( -270.1025481742786951, -91.18033988749901653, 0.000000000000000000 ) ) ;
#2170=ORIENTED_EDGE ( 'NONE', *, *, #26246, .T. ) ;
#2174=CARTESIAN_POINT ( 'NONE',  ( -254.3350114625770289, -91.18033988749901653, 0.000000000000000000 ) ) ;
#2175=LINE ( 'NONE', #17987, #5245 ) ;
#2178=CIRCLE ( 'NONE', #27455, 53.86582179324592090 ) ;
#2179=FACE_OUTER_BOUND ( 'NONE', #21456, .T. ) ;
#2180=DIRECTION ( 'NONE',  ( -1.000000000000000000, 0.000000000000000000, 0.000000000000000000 ) ) ;
#2182=ORIENTED_EDGE ( 'NONE', *, *, #15398, .F. ) ;
#2184=CARTESIAN_POINT ( 'NONE',  ( -191.3061555549459740, 102.2427340594756799, -32.85867620729514016 ) ) ;
#2187=CARTESIAN_POINT ( 'NONE',  ( -110.9204421502694089, 68.96622493949561772, 82.96750001901793325 ) ) ;
#2191=CARTESIAN_POINT ( 'NONE',  ( -24.75198612830871525, 128.0415922265599988, 17.48639942061494779 ) ) ;
#2200=DIRECTION ( 'NONE',  ( 0.000000000000000000, 0.000000000000000000, 1.000000000000000000 ) ) ;
#2201=DIRECTION ( 'NONE',  ( 0.000000000000000000, 0.7071067811865476838, 0.7071067811865474617 ) ) ;
#2206=DIRECTION ( 'NONE',  ( -0.000000000000000000, -1.000000000000000000, -0.000000000000000000 ) ) ;
#2211=CARTESIAN_POINT ( 'NONE',  ( -243.4285414610288001, 74.63108012613849951, -5.000000000000003553 ) ) ;
#2217=CARTESIAN_POINT ( 'NONE',  ( -208.0993096659099706, 75.16660988589454462, 39.82168146137254183 ) ) ;
#2224=DIRECTION ( 'NONE',  ( 0.000000000000000000, 0.000000000000000000, 1.000000000000000000 ) ) ;
#2226=EDGE_LOOP ( 'NONE', ( #21509, #4971, #16679, #25481, #14713, #23538 ) ) ;
#2228=CARTESIAN_POINT ( 'NONE',  ( -226.9194714820147851, 131.5555516077983498, 12.99999999956374275 ) ) ;
#2229=CARTESIAN_POINT ( 'NONE',  ( 98.85598102459226766, 241.6222630368753528, 21.45481330788183527 ) ) ;
#2231=LINE ( 'NONE', #24359, #12852 ) ;
#2236=CIRCLE ( 'NONE', #15547, 9.999999999999991118 ) ;
#2239=ADVANCED_FACE ( 'NONE', ( #24693 ), #4571, .T. ) ;
#2242=DIRECTION ( 'NONE',  ( 1.000000000000000000, 4.163336342344337027E-16, 0.000000000000000000 ) ) ;
#2245=VECTOR ( 'NONE', #17439, 1000.000000000000000 ) ;
#2247=FACE_OUTER_BOUND ( 'NONE', #3999, .T. ) ;
#2248=AXIS2_PLACEMENT_3D ( 'NONE', #4320, #595, #24157 ) ;
#2249=DIRECTION ( 'NONE',  ( 0.000000000000000000, 0.000000000000000000, 1.000000000000000000 ) ) ;
#2254=CARTESIAN_POINT ( 'NONE',  ( 109.9730600663540372, 258.3045051371750560, -43.53165882719768831 ) ) ;
#2255=EDGE_LOOP ( 'NONE', ( #1277, #11284, #6297, #21132 ) ) ;
#2260=B_SPLINE_CURVE_WITH_KNOTS ( 'NONE', 3,
 ( #23158, #20993, #8356, #27588, #18985, #27447, #25579, #5906, #7791, #16974, #25726, #6051, #14832, #17116, #23583, #12682, #10509, #25870, #6196, #23721, #5632, #3467, #4031, #14404, #12818, #12257, #9946, #18703, #15113, #20373, #8498, #6330, #21712, #700 ),
 .UNSPECIFIED., .F., .F.,
 ( 4, 2, 2, 2, 2, 2, 2, 2, 2, 2, 2, 2, 2, 2, 2, 2, 4 ),
 ( -3.473018576686760843E-05, 0.003158948505162983023, 0.006352627196092834258, 0.01273998457795253066, 0.01912734195981235022, 0.02232102065074227995, 0.02551469934167219233, 0.03190205672353205180, 0.03509573541446200928, 0.03669257475992701578, 0.03828941410539202228, 0.04148309279632195895, 0.04307993214178691688, 0.04467677148725186786, 0.04627361083271682579, 0.04787045017818177678, 0.05106412886911163712 ),
 .UNSPECIFIED. ) ;
#2262=ORIENTED_EDGE ( 'NONE', *, *, #13884, .T. ) ;
#2263=CARTESIAN_POINT ( 'NONE',  ( -141.6428522700808230, 74.54464929955099706, 83.00000000000001421 ) ) ;
#2264=AXIS2_PLACEMENT_3D ( 'NONE', #2700, #11190, #6725 ) ;
#2266=EDGE_CURVE ( 'NONE', #14227, #20107, #3930, .T. ) ;
#2268=CARTESIAN_POINT ( 'NONE',  ( 79.99999999999990052, 139.9999999999999716, -15.00000000000000000 ) ) ;
#2270=CARTESIAN_POINT ( 'NONE',  ( -223.4403667166160972, 71.79593500864935152, 19.27754551403305427 ) ) ;
#2274=EDGE_CURVE ( 'NONE', #14725, #19755, #13595, .T. ) ;
#2278=CARTESIAN_POINT ( 'NONE',  ( 9.999999999999749534, 90.00000000000001421, 80.00000000000001421 ) ) ;
#2279=TOROIDAL_SURFACE ( 'NONE', #22015, 16.91094714394370158, 6.204828372381208546 ) ;
#2280=CARTESIAN_POINT ( 'NONE',  ( -28.14009829505550542, 129.1550027291188201, 16.99829214959097357 ) ) ;
#2281=CARTESIAN_POINT ( 'NONE',  ( -209.8597537650321385, 64.07535392826727616, 30.05220721473784806 ) ) ;
#2285=ORIENTED_EDGE ( 'NONE', *, *, #6104, .T. ) ;
#2286=CARTESIAN_POINT ( 'NONE',  ( -181.5195305165591435, 109.0652686644031633, 30.80202506621170855 ) ) ;
#2290=VERTEX_POINT ( 'NONE', #9182 ) ;
#2295=CARTESIAN_POINT ( 'NONE',  ( 87.74278500253673485, 111.0010834410971370, -100.0000000000000284 ) ) ;
#2298=ADVANCED_FACE ( 'NONE', ( #2706, #19668 ), #7021, .F. ) ;
#2301=CARTESIAN_POINT ( 'NONE',  ( -223.8494703126554271, 88.80400106072828237, 16.69934009789151830 ) ) ;
#2306=EDGE_CURVE ( 'NONE', #11545, #366, #17504, .T. ) ;
#2307=CIRCLE ( 'NONE', #1842, 4.355764593064429313 ) ;
#2310=B_SPLINE_CURVE_WITH_KNOTS ( 'NONE', 3,
 ( #23603, #10254, #23321, #8376, #12423, #25892, #1482, #21016, #14993, #21160, #23742, #10675, #28177, #8522, #17274, #23889, #1344, #14706, #2461, #28315, #8660, #26447 ),
 .UNSPECIFIED., .F., .F.,
 ( 4, 2, 2, 2, 2, 2, 2, 2, 2, 2, 4 ),
 ( 0.000000000000000000, 0.006532603454143737914, 0.01306520690828747583, 0.01633150863535932917, 0.01959781036243118946, 0.02613041381657490309, 0.02939671554364671480, 0.03266301727071851957, 0.03919562072486217075, 0.04572822417900581499, 0.05226082763314945923 ),
 .UNSPECIFIED. ) ;
#2311=CARTESIAN_POINT ( 'NONE',  ( -220.9676528974451060, 136.4492860810281343, -15.12837422688741462 ) ) ;
#2313=DIRECTION ( 'NONE',  ( -0.000000000000000000, -0.000000000000000000, -1.000000000000000000 ) ) ;
#2317=DIRECTION ( 'NONE',  ( 0.000000000000000000, 0.000000000000000000, -1.000000000000000000 ) ) ;
#2318=CARTESIAN_POINT ( 'NONE',  ( 134.9999999999998579, -327.2004514666934369, -84.99999999999997158 ) ) ;
#2319=ORIENTED_EDGE ( 'NONE', *, *, #20746, .T. ) ;
#2320=DIRECTION ( 'NONE',  ( 0.000000000000000000, 0.000000000000000000, 1.000000000000000000 ) ) ;
#2321=ORIENTED_EDGE ( 'NONE', *, *, #27279, .T. ) ;
#2325=CARTESIAN_POINT ( 'NONE',  ( -187.1339768309721876, 105.1645070492825482, -32.59344809072628379 ) ) ;
#2327=ORIENTED_EDGE ( 'NONE', *, *, #17388, .T. ) ;
#2329=VECTOR ( 'NONE', #14493, 1000.000000000000000 ) ;
#2331=EDGE_CURVE ( 'NONE', #3986, #10475, #14982, .T. ) ;
#2333=ORIENTED_EDGE ( 'NONE', *, *, #19276, .F. ) ;
#2340=CARTESIAN_POINT ( 'NONE',  ( -210.0005531822249338, 60.15481880046607444, -20.01098946152725944 ) ) ;
#2342=VERTEX_POINT ( 'NONE', #5291 ) ;
#2346=DIRECTION ( 'NONE',  ( 0.000000000000000000, 0.000000000000000000, 1.000000000000000000 ) ) ;
#2347=CARTESIAN_POINT ( 'NONE',  ( 123.9999999999998579, 220.0000000000000284, -100.0000000000000142 ) ) ;
#2353=DIRECTION ( 'NONE',  ( 0.000000000000000000, 1.000000000000000000, 0.000000000000000000 ) ) ;
#2358=ORIENTED_EDGE ( 'NONE', *, *, #10579, .F. ) ;
#2359=CIRCLE ( 'NONE', #18432, 30.00000000000000000 ) ;
#2360=TOROIDAL_SURFACE ( 'NONE', #9727, 66.76834224489934400, 2.000000000000000000 ) ;
#2370=VERTEX_POINT ( 'NONE', #18649 ) ;
#2372=CARTESIAN_POINT ( 'NONE',  ( -224.0246150495877089, 134.1142769380900290, 12.98324324887168224 ) ) ;
#2373=CARTESIAN_POINT ( 'NONE',  ( 87.49999999999988631, 240.0000000000000284, 15.95262490344436479 ) ) ;
#2374=AXIS2_PLACEMENT_3D ( 'NONE', #11423, #18021, #2070 ) ;
#2377=CIRCLE ( 'NONE', #6507, 14.13483123440684253 ) ;
#2381=CYLINDRICAL_SURFACE ( 'NONE', #5605, 5.000000000000004441 ) ;
#2385=LINE ( 'NONE', #17911, #6577 ) ;
#2386=EDGE_LOOP ( 'NONE', ( #20127, #13253, #27932, #9202 ) ) ;
#2389=CARTESIAN_POINT ( 'NONE',  ( 123.9999999999998579, 220.0000000000000284, 100.0000000000000142 ) ) ;
#2391=ORIENTED_EDGE ( 'NONE', *, *, #3143, .T. ) ;
#2392=VECTOR ( 'NONE', #25105, 1000.000000000000000 ) ;
#2393=CIRCLE ( 'NONE', #7466, 6.000000000000005329 ) ;
#2396=CARTESIAN_POINT ( 'NONE',  ( -27.08958435577652679, 129.1630609446471283, -15.68767212615508555 ) ) ;
#2397=ORIENTED_EDGE ( 'NONE', *, *, #1538, .T. ) ;
#2402=EDGE_CURVE ( 'NONE', #17181, #7680, #13623, .T. ) ;
#2403=EDGE_CURVE ( 'NONE', #4097, #7691, #23380, .T. ) ;
#2404=VERTEX_POINT ( 'NONE', #21362 ) ;
#2406=CARTESIAN_POINT ( 'NONE',  ( 119.9999999999999432, 2.220446049250311819E-14, -100.0000000000000142 ) ) ;
#2409=DIRECTION ( 'NONE',  ( 0.000000000000000000, 0.000000000000000000, -1.000000000000000000 ) ) ;
#2411=CARTESIAN_POINT ( 'NONE',  ( -223.4642351922133230, 61.48957812540078294, 20.50364820523368081 ) ) ;
#2414=AXIS2_PLACEMENT_3D ( 'NONE', #575, #22834, #990 ) ;
#2416=CARTESIAN_POINT ( 'NONE',  ( -221.3650667873343139, -91.18033988749901653, -19.29759039828519818 ) ) ;
#2421=CARTESIAN_POINT ( 'NONE',  ( 4.597555261273185145, 138.9914208893002012, 14.95400808356685829 ) ) ;
#2424=DIRECTION ( 'NONE',  ( 0.000000000000000000, 0.000000000000000000, 1.000000000000000000 ) ) ;
#2426=ORIENTED_EDGE ( 'NONE', *, *, #23498, .F. ) ;
#2427=CARTESIAN_POINT ( 'NONE',  ( -230.9082317474560284, 90.07627812137737067, -15.14563771791813807 ) ) ;
#2428=EDGE_CURVE ( 'NONE', #8538, #20676, #17197, .T. ) ;
#2429=EDGE_CURVE ( 'NONE', #24936, #20648, #8441, .T. ) ;
#2434=AXIS2_PLACEMENT_3D ( 'NONE', #16289, #18295, #25042 ) ;
#2436=EDGE_CURVE ( 'NONE', #17217, #19021, #14055, .T. ) ;
#2439=LINE ( 'NONE', #22708, #19095 ) ;
#2442=CIRCLE ( 'NONE', #9801, 6.000000000000005329 ) ;
#2443=DIRECTION ( 'NONE',  ( 1.000000000000000000, 0.000000000000000000, 0.000000000000000000 ) ) ;
#2446=CARTESIAN_POINT ( 'NONE',  ( -225.8597555539711266, 89.56459113752090673, 13.95703860800441198 ) ) ;
#2448=DIRECTION ( 'NONE',  ( 0.2845658198851049314, -0.9586565047779721516, 0.000000000000000000 ) ) ;
#2450=AXIS2_PLACEMENT_3D ( 'NONE', #27703, #23273, #19099 ) ;
#2454=CARTESIAN_POINT ( 'NONE',  ( -270.1025481742786951, -91.18033988749901653, 0.000000000000000000 ) ) ;
#2456=VECTOR ( 'NONE', #2206, 1000.000000000000000 ) ;
#2457=DIRECTION ( 'NONE',  ( 0.000000000000000000, -1.000000000000000000, 0.000000000000000000 ) ) ;
#2461=CARTESIAN_POINT ( 'NONE',  ( -168.2164813390208735, 116.6601697747547774, 24.58600857313708943 ) ) ;
#2462=CARTESIAN_POINT ( 'NONE',  ( -140.3161500669093300, 71.26253677735444114, 82.82425304866107751 ) ) ;
#2467=CARTESIAN_POINT ( 'NONE',  ( -203.3278902001933659, 92.92226908766613747, -29.32321494459339561 ) ) ;
#2470=ORIENTED_EDGE ( 'NONE', *, *, #16341, .T. ) ;
#2477=CARTESIAN_POINT ( 'NONE',  ( -4.673085614201822224, 132.3311587643906080, 15.99381942260592915 ) ) ;
#2480=CARTESIAN_POINT ( 'NONE',  ( -4.177201536621815592, 134.2095850109177775, -15.52423248666405620 ) ) ;
#2486=PLANE ( 'NONE',  #26428 ) ;
#2488=CARTESIAN_POINT ( 'NONE',  ( -71.37541315349507443, 150.2892445414773590, 15.00000000000000000 ) ) ;
#2493=ORIENTED_EDGE ( 'NONE', *, *, #5631, .F. ) ;
#2496=CARTESIAN_POINT ( 'NONE',  ( -227.3759666274727635, 63.27997354833448185, -7.997465051287307780 ) ) ;
#2498=ORIENTED_EDGE ( 'NONE', *, *, #19631, .F. ) ;
#2501=VERTEX_POINT ( 'NONE', #26654 ) ;
#2504=CARTESIAN_POINT ( 'NONE',  ( 106.4997226413335767, 248.6818526014546933, 25.16395533540803697 ) ) ;
#2508=FACE_BOUND ( 'NONE', #21235, .T. ) ;
#2510=EDGE_CURVE ( 'NONE', #26112, #27164, #15341, .T. ) ;
#2513=AXIS2_PLACEMENT_3D ( 'NONE', #27989, #16672, #14520 ) ;
#2514=CARTESIAN_POINT ( 'NONE',  ( 100.3999191023796129, 235.3978472240583528, 22.98606999220467628 ) ) ;
#2517=CIRCLE ( 'NONE', #6650, 29.99999999999999645 ) ;
#2521=DIRECTION ( 'NONE',  ( 3.469446951953614189E-16, -1.000000000000000000, 0.000000000000000000 ) ) ;
#2528=EDGE_LOOP ( 'NONE', ( #4936, #24683, #23676, #15932 ) ) ;
#2530=EDGE_CURVE ( 'NONE', #20966, #20254, #4399, .T. ) ;
#2533=AXIS2_PLACEMENT_3D ( 'NONE', #12161, #19311, #8400 ) ;
#2534=EDGE_CURVE ( 'NONE', #26994, #7257, #97, .T. ) ;
#2537=CIRCLE ( 'NONE', #19975, 6.025000000000002132 ) ;
#2549=EDGE_LOOP ( 'NONE', ( #25187, #4897, #16302, #11872 ) ) ;
#2550=DIRECTION ( 'NONE',  ( 1.000000000000000000, 0.000000000000000000, 0.000000000000000000 ) ) ;
#2557=CARTESIAN_POINT ( 'NONE',  ( -213.5622695550087258, 60.06483686772712360, 14.69413405016535989 ) ) ;
#2565=CARTESIAN_POINT ( 'NONE',  ( 109.5756401952765486, 134.3783162856070703, 89.68749999971406339 ) ) ;
#2567=EDGE_CURVE ( 'NONE', #8949, #19837, #20429, .T. ) ;
#2572=ORIENTED_EDGE ( 'NONE', *, *, #18724, .F. ) ;
#2573=EDGE_LOOP ( 'NONE', ( #3042, #14337, #8142, #14582, #16339, #2285, #2327, #26159 ) ) ;
#2574=CARTESIAN_POINT ( 'NONE',  ( -204.3509971620249246, 91.62525467510273813, -29.24375089551106299 ) ) ;
#2575=FACE_OUTER_BOUND ( 'NONE', #5410, .T. ) ;
#2576=CARTESIAN_POINT ( 'NONE',  ( -203.8386979721259422, 92.04489626552744141, -29.52689898475847485 ) ) ;
#2577=ORIENTED_EDGE ( 'NONE', *, *, #27411, .F. ) ;
#2586=CIRCLE ( 'NONE', #20946, 1.999999999999998890 ) ;
#2590=CARTESIAN_POINT ( 'NONE',  ( -202.3849748766693892, 93.73600923071712998, -29.14529524674100003 ) ) ;
#2591=EDGE_LOOP ( 'NONE', ( #12892, #8005, #27859, #10565, #27979 ) ) ;
#2596=DIRECTION ( 'NONE',  ( -1.850371707708594316E-16, 1.000000000000000000, 0.000000000000000000 ) ) ;
#2598=CARTESIAN_POINT ( 'NONE',  ( -206.8153965817337223, 60.16463287088505751, -19.99797379519590379 ) ) ;
#2603=DIRECTION ( 'NONE',  ( 0.000000000000000000, -1.000000000000000000, 0.000000000000000000 ) ) ;
#2605=DIRECTION ( 'NONE',  ( 1.000000000000000000, 1.657962687179363279E-15, 0.000000000000000000 ) ) ;
#2614=VERTEX_POINT ( 'NONE', #18479 ) ;
#2615=AXIS2_PLACEMENT_3D ( 'NONE', #5318, #16666, #9920 ) ;
#2617=LINE ( 'NONE', #11833, #17754 ) ;
#2620=ORIENTED_EDGE ( 'NONE', *, *, #8426, .T. ) ;
#2623=CARTESIAN_POINT ( 'NONE',  ( -38.51941377410816614, 128.7763188256022318, 17.17685746774373357 ) ) ;
#2626=LINE ( 'NONE', #2772, #22679 ) ;
#2627=CARTESIAN_POINT ( 'NONE',  ( -31.54578268729987656, 129.2273646750841181, -15.65862884027403190 ) ) ;
#2628=DIRECTION ( 'NONE',  ( 0.000000000000000000, 0.000000000000000000, -1.000000000000000000 ) ) ;
#2635=B_SPLINE_CURVE_WITH_KNOTS ( 'NONE', 3,
 ( #6213, #1753, #10388, #14703, #27471, #25744, #6072, #10531 ),
 .UNSPECIFIED., .F., .F.,
 ( 4, 2, 2, 4 ),
 ( 0.000000000000000000, 0.003477520733619417822, 0.005216281100429110036, 0.006955041467238803551 ),
 .UNSPECIFIED. ) ;
#2639=AXIS2_PLACEMENT_3D ( 'NONE', #16359, #23239, #27115 ) ;
#2640=VERTEX_POINT ( 'NONE', #25218 ) ;
#2641=CARTESIAN_POINT ( 'NONE',  ( -220.3653290071073059, 61.04242272473437936, 10.83006322850142311 ) ) ;
#2651=CARTESIAN_POINT ( 'NONE',  ( -208.9953786179366091, 74.56197851221769213, 36.88754066616979799 ) ) ;
#2652=ORIENTED_EDGE ( 'NONE', *, *, #27128, .F. ) ;
#2660=ORIENTED_EDGE ( 'NONE', *, *, #8195, .T. ) ;
#2661=VERTEX_POINT ( 'NONE', #1087 ) ;
#2662=CARTESIAN_POINT ( 'NONE',  ( 96.75280658369925391, 240.7143248587420317, 19.91790936282351865 ) ) ;
#2663=EDGE_CURVE ( 'NONE', #17425, #12131, #7147, .T. ) ;
#2667=CARTESIAN_POINT ( 'NONE',  ( -63.57415822541634043, -18.01420295945611727, 80.00000000000001421 ) ) ;
#2669=DIRECTION ( 'NONE',  ( -1.000000000000000000, 0.000000000000000000, 0.000000000000000000 ) ) ;
#2670=FACE_OUTER_BOUND ( 'NONE', #9794, .T. ) ;
#2671=DIRECTION ( 'NONE',  ( 1.321694076934710155E-16, -1.000000000000000000, 0.000000000000000000 ) ) ;
#2672=CARTESIAN_POINT ( 'NONE',  ( 6.071532165918828775E-15, -70.00000000000002842, -25.00000000000000000 ) ) ;
#2673=CARTESIAN_POINT ( 'NONE',  ( -196.7918453702777128, 68.51688903468615877, 83.00000000000001421 ) ) ;
#2674=CARTESIAN_POINT ( 'NONE',  ( 134.9999999999998579, 220.0000000000000284, 100.0000000000000142 ) ) ;
#2675=VERTEX_POINT ( 'NONE', #5537 ) ;
#2682=DIRECTION ( 'NONE',  ( -0.5790253867566337309, -0.8153095126952284444, -1.131469241487697676E-14 ) ) ;
#2684=ORIENTED_EDGE ( 'NONE', *, *, #17239, .F. ) ;
#2693=ORIENTED_EDGE ( 'NONE', *, *, #24007, .F. ) ;
#2695=CARTESIAN_POINT ( 'NONE',  ( -86.54034876329639303, 136.4599515387363624, 13.48322035540682151 ) ) ;
#2700=CARTESIAN_POINT ( 'NONE',  ( -210.0000000000000284, -3.238150488490040751E-14, 100.0000000000000142 ) ) ;
#2704=CARTESIAN_POINT ( 'NONE',  ( -225.5840809296988141, 72.49952595023175661, 18.07266724760005516 ) ) ;
#2706=FACE_BOUND ( 'NONE', #16319, .T. ) ;
#2708=CARTESIAN_POINT ( 'NONE',  ( -215.2757279354555919, 87.86214960428041820, -19.31485547342763098 ) ) ;
#2713=DIRECTION ( 'NONE',  ( 1.000000000000000000, 0.000000000000000000, 0.000000000000000000 ) ) ;
#2714=CARTESIAN_POINT ( 'NONE',  ( -2.862293735361731706E-14, 109.9999999999999858, 100.0000000000000142 ) ) ;
#2716=CARTESIAN_POINT ( 'NONE',  ( 79.99999999999992895, 240.0000000000000284, 45.00000000000000000 ) ) ;
#2718=ORIENTED_EDGE ( 'NONE', *, *, #708, .F. ) ;
#2720=CARTESIAN_POINT ( 'NONE',  ( 109.9999999999998863, 330.0000000000000000, 90.00000000000002842 ) ) ;
#2728=CARTESIAN_POINT ( 'NONE',  ( -149.5659937850672634, 124.9543708090996574, 17.81989871787508051 ) ) ;
#2730=EDGE_LOOP ( 'NONE', ( #18731, #8266, #3213, #4515 ) ) ;
#2734=CARTESIAN_POINT ( 'NONE',  ( -199.9534965974906697, 95.77273073869348252, -30.16924269412446336 ) ) ;
#2735=ORIENTED_EDGE ( 'NONE', *, *, #11773, .T. ) ;
#2736=CARTESIAN_POINT ( 'NONE',  ( -203.2481855153401966, 92.57460631283321106, 29.78692811926997663 ) ) ;
#2737=DIRECTION ( 'NONE',  ( -0.000000000000000000, -0.000000000000000000, 1.000000000000000000 ) ) ;
#2741=CARTESIAN_POINT ( 'NONE',  ( -213.6504899993060747, 58.00877466446873143, -34.94433424773174579 ) ) ;
#2751=CARTESIAN_POINT ( 'NONE',  ( -233.5270925706182084, 66.28764270640111533, 15.64035431904695805 ) ) ;
#2757=DIRECTION ( 'NONE',  ( -0.000000000000000000, -0.000000000000000000, -1.000000000000000000 ) ) ;
#2758=ORIENTED_EDGE ( 'NONE', *, *, #11844, .T. ) ;
#2761=ADVANCED_FACE ( 'NONE', ( #10279, #21327 ), #25499, .T. ) ;
#2772=CARTESIAN_POINT ( 'NONE',  ( -68.57415822541635464, -23.01420295945612082, 95.00000000000000000 ) ) ;
#2773=CARTESIAN_POINT ( 'NONE',  ( -23.72765020131021529, 129.3221281329265366, -15.61619972759512720 ) ) ;
#2778=ORIENTED_EDGE ( 'NONE', *, *, #25500, .T. ) ;
#2784=CARTESIAN_POINT ( 'NONE',  ( -77.29631966220713934, 4.740818392941742232, -13.00000000000000000 ) ) ;
#2787=CARTESIAN_POINT ( 'NONE',  ( 179.9999999999999147, 0.000000000000000000, 100.0000000000000142 ) ) ;
#2793=EDGE_CURVE ( 'NONE', #10017, #14295, #2537, .T. ) ;
#2804=EDGE_CURVE ( 'NONE', #16689, #13440, #17159, .T. ) ;
#2807=CARTESIAN_POINT ( 'NONE',  ( 95.18208312637723623, 240.6790578601105892, 9.159889466451698325 ) ) ;
#2808=CARTESIAN_POINT ( 'NONE',  ( -224.0246150495857478, 134.1142769380917343, 12.98324324876687719 ) ) ;
#2812=DIRECTION ( 'NONE',  ( 0.000000000000000000, 0.000000000000000000, -1.000000000000000000 ) ) ;
#2813=AXIS2_PLACEMENT_3D ( 'NONE', #28244, #23957, #2106 ) ;
#2818=VECTOR ( 'NONE', #7258, 1000.000000000000000 ) ;
#2822=CARTESIAN_POINT ( 'NONE',  ( -175.8417606860892874, 246.9430296707336652, -15.00000000000000000 ) ) ;
#2824=DIRECTION ( 'NONE',  ( 1.000000000000000000, 0.000000000000000000, 0.000000000000000000 ) ) ;
#2827=CARTESIAN_POINT ( 'NONE',  ( 109.7839892703133984, 255.7665025292603787, -41.33169715142309997 ) ) ;
#2828=VERTEX_POINT ( 'NONE', #14453 ) ;
#2829=DIRECTION ( 'NONE',  ( 4.625929269271485914E-16, -1.000000000000000000, 0.000000000000000000 ) ) ;
#2831=EDGE_LOOP ( 'NONE', ( #442, #8029, #18174, #19658 ) ) ;
#2832=CIRCLE ( 'NONE', #5586, 5.000000000000004441 ) ;
#2835=VERTEX_POINT ( 'NONE', #3802 ) ;
#2837=DIRECTION ( 'NONE',  ( 0.000000000000000000, 0.000000000000000000, -1.000000000000000000 ) ) ;
#2842=EDGE_CURVE ( 'NONE', #10961, #11100, #8119, .T. ) ;
#2844=CARTESIAN_POINT ( 'NONE',  ( -100.4013316720778874, 135.9145549716820938, -13.58265865227119029 ) ) ;
#2846=DIRECTION ( 'NONE',  ( 1.000000000000000000, 0.000000000000000000, 0.000000000000000000 ) ) ;
#2848=CARTESIAN_POINT ( 'NONE',  ( -113.0191929279866230, 134.5409307879479002, -13.86300596970152377 ) ) ;
#2849=CARTESIAN_POINT ( 'NONE',  ( 79.99999999999991473, 109.0404994605766831, -77.77847705527373989 ) ) ;
#2851=DIRECTION ( 'NONE',  ( -0.000000000000000000, 1.000000000000000000, 0.000000000000000000 ) ) ;
#2852=DIRECTION ( 'NONE',  ( 1.000000000000000000, -0.000000000000000000, -0.000000000000000000 ) ) ;
#2854=ADVANCED_FACE ( 'NONE', ( #3940 ), #18750, .T. ) ;
#2858=CARTESIAN_POINT ( 'NONE',  ( 8.117852850209661852, 141.5785587194356481, 14.99999999999999467 ) ) ;
#2860=CARTESIAN_POINT ( 'NONE',  ( -163.8466752748964836, 118.1093140208040069, 24.36087108768327880 ) ) ;
#2862=AXIS2_PLACEMENT_3D ( 'NONE', #20346, #22362, #11460 ) ;
#2863=ORIENTED_EDGE ( 'NONE', *, *, #27885, .T. ) ;
#2864=ORIENTED_EDGE ( 'NONE', *, *, #21490, .F. ) ;
#2865=CARTESIAN_POINT ( 'NONE',  ( -205.4480570425783412, 90.78711157365827944, -28.57879582564067533 ) ) ;
#2866=VECTOR ( 'NONE', #9491, 1000.000000000000000 ) ;
#2872=CARTESIAN_POINT ( 'NONE',  ( -112.9120396111939897, 134.5581283993135173, 15.44207887828286552 ) ) ;
#2874=ORIENTED_EDGE ( 'NONE', *, *, #18254, .T. ) ;
#2879=ADVANCED_FACE ( 'NONE', ( #6241 ), #23209, .F. ) ;
#2884=CIRCLE ( 'NONE', #25359, 22.49999999999999289 ) ;
#2885=CARTESIAN_POINT ( 'NONE',  ( 88.54392521371902092, 230.0000000000000000, -16.22216523460573256 ) ) ;
#2886=AXIS2_PLACEMENT_3D ( 'NONE', #15750, #13738, #2083 ) ;
#2889=CARTESIAN_POINT ( 'NONE',  ( -213.2358879321101313, 57.03087831670951147, -38.93822867433466683 ) ) ;
#2891=CARTESIAN_POINT ( 'NONE',  ( -2.862293735361731706E-14, 109.9999999999999858, -70.00000000000001421 ) ) ;
#2893=DIRECTION ( 'NONE',  ( -1.000000000000000000, 0.000000000000000000, 0.000000000000000000 ) ) ;
#2895=ORIENTED_EDGE ( 'NONE', *, *, #8348, .T. ) ;
#2897=AXIS2_PLACEMENT_3D ( 'NONE', #9814, #27318, #12824 ) ;
#2898=CARTESIAN_POINT ( 'NONE',  ( 144.9999999999998863, 220.0000000000000284, -99.00000000000001421 ) ) ;
#2899=EDGE_CURVE ( 'NONE', #9431, #16453, #26057, .T. ) ;
#2900=AXIS2_PLACEMENT_3D ( 'NONE', #5795, #12279, #19011 ) ;
#2901=CARTESIAN_POINT ( 'NONE',  ( -236.2188936948037110, 81.35702876104957681, 15.00000000000000000 ) ) ;
#2903=ORIENTED_EDGE ( 'NONE', *, *, #600, .F. ) ;
#2904=EDGE_CURVE ( 'NONE', #12426, #17375, #26619, .T. ) ;
#2905=TOROIDAL_SURFACE ( 'NONE', #4718, 19.29759039828519818, 4.355764593064427537 ) ;
#2906=VERTEX_POINT ( 'NONE', #10703 ) ;
#2907=CARTESIAN_POINT ( 'NONE',  ( 79.99999999999991473, 110.0000000000000142, 70.00000000000001421 ) ) ;
#2908=DIRECTION ( 'NONE',  ( -0.000000000000000000, 1.000000000000000000, -1.387778780781445429E-16 ) ) ;
#2912=CARTESIAN_POINT ( 'NONE',  ( -215.4886702565632106, 139.8420026707765942, 13.00000000000000000 ) ) ;
#2913=ORIENTED_EDGE ( 'NONE', *, *, #801, .T. ) ;
#2915=EDGE_LOOP ( 'NONE', ( #12043, #16735, #15307, #27801 ) ) ;
#2916=TOROIDAL_SURFACE ( 'NONE', #12571, 16.91094714394370158, 6.204828372381208546 ) ;
#2921=CARTESIAN_POINT ( 'NONE',  ( -24.81898458245972350, 129.2519120894625644, -16.96078301911394703 ) ) ;
#2922=CIRCLE ( 'NONE', #20808, 2.586968381275096984 ) ;
#2924=DIRECTION ( 'NONE',  ( 0.000000000000000000, 0.000000000000000000, 1.000000000000000000 ) ) ;
#2929=CARTESIAN_POINT ( 'NONE',  ( 139.9999999999999147, -120.0000000000000284, 100.0000000000000142 ) ) ;
#2937=CARTESIAN_POINT ( 'NONE',  ( 134.9999999999998579, 220.0000000000000284, 153.1081322850112940 ) ) ;
#2938=DIRECTION ( 'NONE',  ( 0.000000000000000000, -1.000000000000000000, 0.000000000000000000 ) ) ;
#2941=CARTESIAN_POINT ( 'NONE',  ( 134.9999999999998579, 220.0000000000000284, 99.00000000000001421 ) ) ;
#2948=VERTEX_POINT ( 'NONE', #4786 ) ;
#2954=CARTESIAN_POINT ( 'NONE',  ( -189.8086322075389774, 92.49158130768422836, -15.00000000000000000 ) ) ;
#2956=CIRCLE ( 'NONE', #22235, 10.00000000000000000 ) ;
#2960=DIRECTION ( 'NONE',  ( 0.000000000000000000, 0.000000000000000000, -1.000000000000000000 ) ) ;
#2967=ADVANCED_FACE ( 'NONE', ( #11122 ), #19879, .T. ) ;
#2979=VECTOR ( 'NONE', #13163, 1000.000000000000000 ) ;
#2980=ORIENTED_EDGE ( 'NONE', *, *, #16533, .T. ) ;
#2984=CARTESIAN_POINT ( 'NONE',  ( -92.73537453553964838, 136.3631398600097100, -15.17402401083296404 ) ) ;
#2986=CARTESIAN_POINT ( 'NONE',  ( -42.53273978471831640, 130.9733465240572627, 14.93735646117640847 ) ) ;
#2987=CARTESIAN_POINT ( 'NONE',  ( -213.9337484054510128, 55.48171494544478577, 43.35284082257812344 ) ) ;
#2989=EDGE_CURVE ( 'NONE', #1063, #15830, #8684, .T. ) ;
#2990=CARTESIAN_POINT ( 'NONE',  ( -92.74367724329803764, 136.3628496310008131, -13.49999433412610728 ) ) ;
#2991=CARTESIAN_POINT ( 'NONE',  ( 79.99999999999997158, 103.8532287674466374, -88.29969375664609288 ) ) ;
#2996=DIRECTION ( 'NONE',  ( -0.000000000000000000, -0.000000000000000000, -1.000000000000000000 ) ) ;
#2997=VECTOR ( 'NONE', #19639, 1000.000000000000000 ) ;
#2999=CARTESIAN_POINT ( 'NONE',  ( -200.0643534088114848, 95.37219532206381700, 31.11168591751386714 ) ) ;
#3000=CARTESIAN_POINT ( 'NONE',  ( 125.3433571860710600, 197.9412384757604570, -84.99999999999997158 ) ) ;
#3001=CIRCLE ( 'NONE', #20434, 5.000000000000004441 ) ;
#3004=CARTESIAN_POINT ( 'NONE',  ( -160.0000000000000568, 230.0000000000000000, 5.000000000000002665 ) ) ;
#3009=CARTESIAN_POINT ( 'NONE',  ( -52.56693897510013613, 133.2842826589903495, 15.71165752789189440 ) ) ;
#3010=ORIENTED_EDGE ( 'NONE', *, *, #6883, .F. ) ;
#3011=AXIS2_PLACEMENT_3D ( 'NONE', #23167, #8076, #5915 ) ;
#3019=AXIS2_PLACEMENT_3D ( 'NONE', #5917, #23445, #1607 ) ;
#3022=CARTESIAN_POINT ( 'NONE',  ( -175.0000000000000000, -120.0000000000001705, 63.97500000000001563 ) ) ;
#3023=FACE_OUTER_BOUND ( 'NONE', #17893, .T. ) ;
#3024=CARTESIAN_POINT ( 'NONE',  ( -203.1048999767863563, 60.64878749907617816, -23.79654850876571359 ) ) ;
#3026=CARTESIAN_POINT ( 'NONE',  ( 3.469446951953618133E-15, -40.00000000000003553, 70.00000000000001421 ) ) ;
#3027=CARTESIAN_POINT ( 'NONE',  ( -160.0000000000000284, 109.9999999999999432, -45.00000000000000000 ) ) ;
#3029=EDGE_LOOP ( 'NONE', ( #17346, #1832, #6012, #8093 ) ) ;
#3033=CARTESIAN_POINT ( 'NONE',  ( -231.9024517383455475, 76.40908368391228578, 15.65418338381032193 ) ) ;
#3037=ORIENTED_EDGE ( 'NONE', *, *, #1009, .T. ) ;
#3040=CARTESIAN_POINT ( 'NONE',  ( -63.57415822541634043, 24.64876300893806160, 100.0000000000000000 ) ) ;
#3042=ORIENTED_EDGE ( 'NONE', *, *, #23294, .T. ) ;
#3043=ADVANCED_FACE ( 'NONE', ( #493 ), #22324, .F. ) ;
#3044=DIRECTION ( 'NONE',  ( 1.000000000000000000, 0.000000000000000000, 0.000000000000000000 ) ) ;
#3048=CARTESIAN_POINT ( 'NONE',  ( 0.000000000000000000, 0.000000000000000000, 95.00000000000000000 ) ) ;
#3056=CARTESIAN_POINT ( 'NONE',  ( -23.16458623837309716, 129.3662862396423350, -15.59652033367907364 ) ) ;
#3057=PLANE ( 'NONE',  #11894 ) ;
#3060=ORIENTED_EDGE ( 'NONE', *, *, #8204, .F. ) ;
#3068=PLANE ( 'NONE',  #5509 ) ;
#3069=CARTESIAN_POINT ( 'NONE',  ( -231.9378824387731299, 93.53122965655670384, 12.99999999999999822 ) ) ;
#3071=CARTESIAN_POINT ( 'NONE',  ( -42.99650729631200363, 71.03850157808263077, 99.00000000000000000 ) ) ;
#3074=CIRCLE ( 'NONE', #9512, 2.586968381275096984 ) ;
#3075=CYLINDRICAL_SURFACE ( 'NONE', #18500, 19.99999999999998934 ) ;
#3076=CARTESIAN_POINT ( 'NONE',  ( 100.4596905818591921, 242.9371963736508917, 14.31527322455832518 ) ) ;
#3077=ORIENTED_EDGE ( 'NONE', *, *, #26807, .F. ) ;
#3080=ORIENTED_EDGE ( 'NONE', *, *, #12830, .T. ) ;
#3089=AXIS2_PLACEMENT_3D ( 'NONE', #11013, #1951, #28231 ) ;
#3090=CARTESIAN_POINT ( 'NONE',  ( 96.92716526682083611, 115.1868982021453149, -77.49999999976235188 ) ) ;
#3093=CARTESIAN_POINT ( 'NONE',  ( 125.3433571860711453, 242.0587615242396566, 0.000000000000000000 ) ) ;
#3096=DIRECTION ( 'NONE',  ( 0.000000000000000000, 0.000000000000000000, -1.000000000000000000 ) ) ;
#3097=CARTESIAN_POINT ( 'NONE',  ( 114.1093725872594575, 211.6289295222773603, -98.08429852854942510 ) ) ;
#3109=ORIENTED_EDGE ( 'NONE', *, *, #22979, .F. ) ;
#3111=EDGE_CURVE ( 'NONE', #17042, #24468, #21512, .T. ) ;
#3113=CARTESIAN_POINT ( 'NONE',  ( -127.8827038603104143, 131.6591692175807964, 14.66642017785206598 ) ) ;
#3114=FACE_OUTER_BOUND ( 'NONE', #9055, .T. ) ;
#3120=CARTESIAN_POINT ( 'NONE',  ( -90.19822669564636897, 136.4341346054573876, -15.16547208303790484 ) ) ;
#3121=CARTESIAN_POINT ( 'NONE',  ( 157.4999999999998579, 220.0000000000000284, 84.99999999999995737 ) ) ;
#3124=DIRECTION ( 'NONE',  ( -0.000000000000000000, 1.000000000000000000, 0.000000000000000000 ) ) ;
#3125=CARTESIAN_POINT ( 'NONE',  ( -100.3939829605125880, 135.9151291309332521, -13.58254898561143342 ) ) ;
#3126=PLANE ( 'NONE',  #12679 ) ;
#3130=CARTESIAN_POINT ( 'NONE',  ( 134.9999999999998579, -327.2004514666934369, -84.99999999999997158 ) ) ;
#3132=DIRECTION ( 'NONE',  ( 0.000000000000000000, -0.000000000000000000, 1.000000000000000000 ) ) ;
#3143=EDGE_CURVE ( 'NONE', #14018, #27164, #13719, .T. ) ;
#3145=EDGE_CURVE ( 'NONE', #19755, #3920, #20727, .T. ) ;
#3146=CIRCLE ( 'NONE', #6824, 6.000000000000005329 ) ;
#3148=ORIENTED_EDGE ( 'NONE', *, *, #2429, .T. ) ;
#3151=VECTOR ( 'NONE', #3185, 1000.000000000000000 ) ;
#3152=EDGE_CURVE ( 'NONE', #11439, #7854, #6559, .T. ) ;
#3154=CARTESIAN_POINT ( 'NONE',  ( 92.44908716912959790, 230.7276285284523567, -17.70004843202667644 ) ) ;
#3156=VECTOR ( 'NONE', #20598, 1000.000000000000000 ) ;
#3160=CARTESIAN_POINT ( 'NONE',  ( -219.3331038875180639, 71.26739478977619058, -22.27060053768705217 ) ) ;
#3163=CARTESIAN_POINT ( 'NONE',  ( -200.0000000000000284, -120.0000000000001279, -25.00000000000000000 ) ) ;
#3164=CARTESIAN_POINT ( 'NONE',  ( 145.9999999999998863, 220.0000000000000284, -99.00000000000001421 ) ) ;
#3166=ORIENTED_EDGE ( 'NONE', *, *, #9750, .T. ) ;
#3168=CIRCLE ( 'NONE', #12828, 30.00000000000000000 ) ;
#3169=CARTESIAN_POINT ( 'NONE',  ( -229.6735579984113258, 64.27833679895920227, 7.258985754582258032 ) ) ;
#3170=LINE ( 'NONE', #11822, #9439 ) ;
#3176=CARTESIAN_POINT ( 'NONE',  ( 98.15430812615089451, 116.0637945823775112, 78.75000000031268144 ) ) ;
#3179=ORIENTED_EDGE ( 'NONE', *, *, #22787, .F. ) ;
#3183=AXIS2_PLACEMENT_3D ( 'NONE', #17308, #4510, #8559 ) ;
#3185=DIRECTION ( 'NONE',  ( -0.000000000000000000, -0.000000000000000000, 1.000000000000000000 ) ) ;
#3187=DIRECTION ( 'NONE',  ( 1.850371707708594316E-16, -1.000000000000000000, 0.000000000000000000 ) ) ;
#3189=CARTESIAN_POINT ( 'NONE',  ( -266.5839533485339530, -91.18033988749901653, 15.26911010665567225 ) ) ;
#3190=AXIS2_PLACEMENT_3D ( 'NONE', #11487, #8749, #20229 ) ;
#3191=EDGE_CURVE ( 'NONE', #25446, #25995, #13931, .T. ) ;
#3193=DIRECTION ( 'NONE',  ( 1.000000000000000000, 2.602085213965211135E-16, -0.000000000000000000 ) ) ;
#3210=DIRECTION ( 'NONE',  ( -1.000000000000000000, 0.000000000000000000, 0.000000000000000000 ) ) ;
#3211=FACE_OUTER_BOUND ( 'NONE', #6243, .T. ) ;
#3213=ORIENTED_EDGE ( 'NONE', *, *, #16118, .F. ) ;
#3217=CARTESIAN_POINT ( 'NONE',  ( -85.18883433891745938, 134.8019439274000604, 15.45375652165002656 ) ) ;
#3218=CARTESIAN_POINT ( 'NONE',  ( -160.0000000000000284, 119.7660240611718621, -22.85081902853005431 ) ) ;
#3220=ORIENTED_EDGE ( 'NONE', *, *, #8000, .T. ) ;
#3226=CARTESIAN_POINT ( 'NONE',  ( 108.4669391321881591, 252.2354088787809303, 31.48703123558444616 ) ) ;
#3229=CARTESIAN_POINT ( 'NONE',  ( -175.0000000000000000, -150.0000000000000853, 76.00000000000001421 ) ) ;
#3230=B_SPLINE_CURVE_WITH_KNOTS ( 'NONE', 3,
 ( #15011, #21601, #4778, #17430, #8956, #26190, #2477, #22459, #11264, #15721, #6515, #15574, #18009, #19592, #2191, #4486, #19728, #22317, #24052, #2623, #484, #10975 ),
 .UNSPECIFIED., .F., .F.,
 ( 4, 2, 2, 2, 2, 2, 2, 2, 2, 2, 4 ),
 ( 0.000000000000000000, 0.006858469009249849001, 0.01371693801849969800, 0.01714617252312462120, 0.02057540702774954613, 0.02743387603699941335, 0.03429234504624928404, 0.03772157955087421938, 0.04115081405549916860, 0.04800928306474905316, 0.05486775207399893772 ),
 .UNSPECIFIED. ) ;
#3238=CARTESIAN_POINT ( 'NONE',  ( -76.25760768171835480, 219.6666220619077876, -13.00000000000000000 ) ) ;
#3239=VERTEX_POINT ( 'NONE', #18396 ) ;
#3241=DIRECTION ( 'NONE',  ( -1.000000000000000000, 0.000000000000000000, 0.000000000000000000 ) ) ;
#3243=DIRECTION ( 'NONE',  ( 0.000000000000000000, 0.000000000000000000, -1.000000000000000000 ) ) ;
#3249=ORIENTED_EDGE ( 'NONE', *, *, #14777, .T. ) ;
#3252=VERTEX_POINT ( 'NONE', #16254 ) ;
#3253=ORIENTED_EDGE ( 'NONE', *, *, #19725, .T. ) ;
#3256=DIRECTION ( 'NONE',  ( -0.000000000000000000, -0.000000000000000000, 1.000000000000000000 ) ) ;
#3260=CARTESIAN_POINT ( 'NONE',  ( -67.51396541345637559, 135.5198389557239693, -15.28949482634511092 ) ) ;
#3261=CARTESIAN_POINT ( 'NONE',  ( -4.279947336434443805, 134.1643719796016683, 13.92784264465264776 ) ) ;
#3267=CARTESIAN_POINT ( 'NONE',  ( -217.1524024359874545, 87.79586245209446815, -18.07482474875216738 ) ) ;
#3270=DIRECTION ( 'NONE',  ( 0.000000000000000000, 0.000000000000000000, 1.000000000000000000 ) ) ;
#3273=CARTESIAN_POINT ( 'NONE',  ( 119.9999999987673220, 136.1131920016294714, -100.0000000000000142 ) ) ;
#3275=CARTESIAN_POINT ( 'NONE',  ( -266.5839533485339530, -91.18033988749901653, 0.000000000000000000 ) ) ;
#3277=EDGE_LOOP ( 'NONE', ( #10786, #8996, #69, #22975 ) ) ;
#3278=EDGE_CURVE ( 'NONE', #7087, #17712, #9918, .T. ) ;
#3285=( GEOMETRIC_REPRESENTATION_CONTEXT ( 3 ) GLOBAL_UNCERTAINTY_ASSIGNED_CONTEXT ( ( #15803 ) ) GLOBAL_UNIT_ASSIGNED_CONTEXT ( ( #5516, #19150, #3633 ) ) REPRESENTATION_CONTEXT ( 'NONE', 'WORKASPACE' ) );
#3287=TOROIDAL_SURFACE ( 'NONE', #25764, 18.46313063346208239, 2.000000000000000000 ) ;
#3293=CARTESIAN_POINT ( 'NONE',  ( 99.70648414290917572, 234.7927111797802695, -22.37570813572899553 ) ) ;
#3297=VECTOR ( 'NONE', #14092, 1000.000000000000000 ) ;
#3299=CARTESIAN_POINT ( 'NONE',  ( -218.7748983233592526, 71.27581659157533522, -22.75434709466339100 ) ) ;
#3303=DIRECTION ( 'NONE',  ( 0.000000000000000000, 0.000000000000000000, -1.000000000000000000 ) ) ;
#3304=DIRECTION ( 'NONE',  ( 1.000000000000000000, 4.625929269271485914E-16, 0.000000000000000000 ) ) ;
#3307=ORIENTED_EDGE ( 'NONE', *, *, #6883, .T. ) ;
#3308=CARTESIAN_POINT ( 'NONE',  ( -254.4816742664885965, 103.7585653882801182, -5.000000000000004441 ) ) ;
#3313=ORIENTED_EDGE ( 'NONE', *, *, #1174, .F. ) ;
#3314=VECTOR ( 'NONE', #26838, 1000.000000000000000 ) ;
#3330=FACE_OUTER_BOUND ( 'NONE', #22023, .T. ) ;
#3341=AXIS2_PLACEMENT_3D ( 'NONE', #22300, #21733, #24034 ) ;
#3348=LINE ( 'NONE', #22476, #11906 ) ;
#3352=DIRECTION ( 'NONE',  ( 0.000000000000000000, 0.000000000000000000, -1.000000000000000000 ) ) ;
#3359=CARTESIAN_POINT ( 'NONE',  ( -138.1489073431982320, 127.5559642418054267, 17.69987763149199722 ) ) ;
#3361=EDGE_LOOP ( 'NONE', ( #9405, #14442, #28120, #24244 ) ) ;
#3362=CONICAL_SURFACE ( 'NONE', #6586, 6.025000000000002132, 0.7853981633974482790 ) ;
#3364=CARTESIAN_POINT ( 'NONE',  ( -24.33210486176665910, 0.000000000000000000, 99.00000000000000000 ) ) ;
#3366=AXIS2_PLACEMENT_3D ( 'NONE', #19576, #26175, #15703 ) ;
#3370=ADVANCED_FACE ( 'NONE', ( #9039 ), #26545, .T. ) ;
#3372=DIRECTION ( 'NONE',  ( 1.000000000000000000, -0.000000000000000000, -0.000000000000000000 ) ) ;
#3374=CARTESIAN_POINT ( 'NONE',  ( 90.17595424773269031, 111.7661400908363731, -72.22656249986501109 ) ) ;
#3378=DIRECTION ( 'NONE',  ( -0.000000000000000000, -0.000000000000000000, 1.000000000000000000 ) ) ;
#3379=CARTESIAN_POINT ( 'NONE',  ( 65.00000000000000000, -120.0000000000000711, 64.00000000000002842 ) ) ;
#3382=ORIENTED_EDGE ( 'NONE', *, *, #14777, .F. ) ;
#3384=CARTESIAN_POINT ( 'NONE',  ( -13.28039411106728629, 129.6310766613705709, 16.84488389623813376 ) ) ;
#3385=DIRECTION ( 'NONE',  ( -0.000000000000000000, -0.000000000000000000, 1.000000000000000000 ) ) ;
#3387=PLANE ( 'NONE',  #7430 ) ;
#3394=DIRECTION ( 'NONE',  ( 0.000000000000000000, 0.000000000000000000, -1.000000000000000000 ) ) ;
#3396=ORIENTED_EDGE ( 'NONE', *, *, #5098, .F. ) ;
#3400=VECTOR ( 'NONE', #7057, 1000.000000000000000 ) ;
#3402=DIRECTION ( 'NONE',  ( 0.000000000000000000, -0.000000000000000000, -1.000000000000000000 ) ) ;
#3403=DIRECTION ( 'NONE',  ( 0.000000000000000000, -0.000000000000000000, -1.000000000000000000 ) ) ;
#3404=CARTESIAN_POINT ( 'NONE',  ( -96.57547103839915792, 136.1729178183695694, -13.53436789263006190 ) ) ;
#3408=CARTESIAN_POINT ( 'NONE',  ( -213.4823095283139196, 56.20074567116226660, 41.47858424781075115 ) ) ;
#3419=CARTESIAN_POINT ( 'NONE',  ( 119.7545560452836639, 132.4900181920934870, -100.0000000000000142 ) ) ;
#3423=VECTOR ( 'NONE', #134, 1000.000000000000000 ) ;
#3426=VERTEX_POINT ( 'NONE', #9181 ) ;
#3432=ORIENTED_EDGE ( 'NONE', *, *, #18706, .F. ) ;
#3433=CARTESIAN_POINT ( 'NONE',  ( -175.0000000000000000, -120.0000000000001847, -69.99999999999998579 ) ) ;
#3437=SPHERICAL_SURFACE ( 'NONE', #2450, 30.00000000000000000 ) ;
#3442=AXIS2_PLACEMENT_3D ( 'NONE', #23186, #14022, #23043 ) ;
#3444=CARTESIAN_POINT ( 'NONE',  ( -208.0931995358751863, 75.17094939810765197, -39.84805955944327138 ) ) ;
#3447=CARTESIAN_POINT ( 'NONE',  ( -215.4886702565632390, 139.8420026707765942, -13.00000000000000178 ) ) ;
#3452=CARTESIAN_POINT ( 'NONE',  ( 134.9999999999998579, 268.4896896257338881, -84.99999999999997158 ) ) ;
#3454=VECTOR ( 'NONE', #15155, 1000.000000000000114 ) ;
#3455=EDGE_LOOP ( 'NONE', ( #5249, #2055, #691, #19902 ) ) ;
#3463=B_SPLINE_CURVE_WITH_KNOTS ( 'NONE', 3,
 ( #8746, #1252, #16493, #18779, #23238, #23371, #3539, #3683, #12470, #8143, #21213, #16633, #21356, #10586, #1535, #14760, #25524, #10443, #23097, #19198, #27945, #10302, #12194, #8290 ),
 .UNSPECIFIED., .F., .F.,
 ( 4, 2, 2, 2, 2, 2, 2, 2, 2, 2, 2, 4 ),
 ( 0.006955041467238803551, 0.01003080572916759117, 0.01156868786013197543, 0.01310656999109636144, 0.01618233425302515599, 0.01772021638398955240, 0.01925809851495395228, 0.02233386277688266877, 0.02387174490784706865, 0.02540962703881146506, 0.02848539130074026482, 0.03156115556266906458 ),
 .UNSPECIFIED. ) ;
#3464=AXIS2_PLACEMENT_3D ( 'NONE', #19455, #19595, #28197 ) ;
#3466=CARTESIAN_POINT ( 'NONE',  ( -138.6428522700808230, 71.54464929955099706, 82.80879831960034210 ) ) ;
#3467=CARTESIAN_POINT ( 'NONE',  ( 97.56710499309299678, 233.1474776945298117, 20.66392395443024554 ) ) ;
#3474=EDGE_CURVE ( 'NONE', #2828, #24530, #21956, .T. ) ;
#3480=CARTESIAN_POINT ( 'NONE',  ( 134.9999999999998579, 220.0000000000000284, 100.0000000000000142 ) ) ;
#3486=AXIS2_PLACEMENT_3D ( 'NONE', #11054, #133, #15516 ) ;
#3488=CARTESIAN_POINT ( 'NONE',  ( 134.9999999999998579, 220.0000000000000284, 90.00000000000002842 ) ) ;
#3493=LINE ( 'NONE', #14020, #23551 ) ;
#3499=EDGE_LOOP ( 'NONE', ( #19416, #24121, #13915, #13198 ) ) ;
#3502=ORIENTED_EDGE ( 'NONE', *, *, #27503, .T. ) ;
#3503=AXIS2_PLACEMENT_3D ( 'NONE', #11553, #22741, #5205 ) ;
#3504=ORIENTED_EDGE ( 'NONE', *, *, #8822, .F. ) ;
#3505=CARTESIAN_POINT ( 'NONE',  ( -110.3221550338875687, 20.24192588826928585, 83.00000000000001421 ) ) ;
#3508=EDGE_LOOP ( 'NONE', ( #24713, #9489, #4551, #13021, #17287, #19091 ) ) ;
#3509=TOROIDAL_SURFACE ( 'NONE', #4412, 80.00000000000000000, 30.00000000000000000 ) ;
#3514=CARTESIAN_POINT ( 'NONE',  ( -210.0000000000000000, -150.0000000000001990, -100.0000000000000142 ) ) ;
#3515=CARTESIAN_POINT ( 'NONE',  ( 33.10302365956999182, 203.2034914284457159, -15.00000000000000000 ) ) ;
#3516=CARTESIAN_POINT ( 'NONE',  ( 22.58950924271104554, 154.2349915562422780, 12.99999999999999822 ) ) ;
#3521=DIRECTION ( 'NONE',  ( 0.000000000000000000, 1.000000000000000000, -1.224646799147353207E-16 ) ) ;
#3522=AXIS2_PLACEMENT_3D ( 'NONE', #24892, #24609, #27178 ) ;
#3525=CARTESIAN_POINT ( 'NONE',  ( 108.6430499291109300, 252.6779224945142062, -32.26435679400692180 ) ) ;
#3526=CARTESIAN_POINT ( 'NONE',  ( 13.66561450649970944, 89.77986226977256479, 98.36120057361384283 ) ) ;
#3533=ORIENTED_EDGE ( 'NONE', *, *, #16413, .F. ) ;
#3534=ORIENTED_EDGE ( 'NONE', *, *, #17358, .F. ) ;
#3535=CARTESIAN_POINT ( 'NONE',  ( -62.54230505217808656, 134.9219987258869651, 15.37840988405203291 ) ) ;
#3536=EDGE_CURVE ( 'NONE', #1808, #23293, #22417, .T. ) ;
#3539=CARTESIAN_POINT ( 'NONE',  ( 113.4521041897136229, 226.4953945451709387, 97.56026172913377081 ) ) ;
#3542=CARTESIAN_POINT ( 'NONE',  ( -68.57415822541635464, 24.64876300893806160, 95.00000000000000000 ) ) ;
#3553=CARTESIAN_POINT ( 'NONE',  ( 9.999999999999957367, -20.00000000000004974, 80.00000000000001421 ) ) ;
#3557=CARTESIAN_POINT ( 'NONE',  ( -36.17830286759925684, -18.63254119118422025, 99.96486317258090537 ) ) ;
#3558=CARTESIAN_POINT ( 'NONE',  ( 95.20156243613460845, 83.09913198707280912, -100.0000000000000284 ) ) ;
#3563=ADVANCED_FACE ( 'NONE', ( #14073 ), #12199, .T. ) ;
#3568=ORIENTED_EDGE ( 'NONE', *, *, #10775, .T. ) ;
#3572=CARTESIAN_POINT ( 'NONE',  ( -2.081668171172168513E-14, 90.00000000000001421, 98.28427124746191623 ) ) ;
#3582=AXIS2_PLACEMENT_3D ( 'NONE', #27371, #1383, #23501 ) ;
#3584=DIRECTION ( 'NONE',  ( 1.000000000000000000, 8.673617379884036705E-17, 0.000000000000000000 ) ) ;
#3586=FACE_OUTER_BOUND ( 'NONE', #20709, .T. ) ;
#3589=VECTOR ( 'NONE', #250, 1000.000000000000000 ) ;
#3592=ORIENTED_EDGE ( 'NONE', *, *, #11348, .F. ) ;
#3597=CARTESIAN_POINT ( 'NONE',  ( 116.3389527601132869, 113.0483370489294543, 100.0000000000000142 ) ) ;
#3598=DIRECTION ( 'NONE',  ( -1.000000000000000000, 0.000000000000000000, 0.000000000000000000 ) ) ;
#3605=CARTESIAN_POINT ( 'NONE',  ( -180.0000000000000284, -70.00000000000004263, -70.00000000000001421 ) ) ;
#3607=CARTESIAN_POINT ( 'NONE',  ( 106.3487426207432804, 91.82653269718771583, 100.0000000000000142 ) ) ;
#3614=DIRECTION ( 'NONE',  ( 1.000000000000000000, 0.000000000000000000, 0.000000000000000000 ) ) ;
#3621=CARTESIAN_POINT ( 'NONE',  ( -225.7036482868739427, -91.18033988749901653, 18.91107291867258411 ) ) ;
#3622=DIRECTION ( 'NONE',  ( 0.000000000000000000, 0.000000000000000000, -1.000000000000000000 ) ) ;
#3630=DIRECTION ( 'NONE',  ( 1.000000000000000000, 0.000000000000000000, 0.000000000000000000 ) ) ;
#3633=( NAMED_UNIT ( * ) SI_UNIT ( $, .STERADIAN. ) SOLID_ANGLE_UNIT ( ) );
#3636=EDGE_CURVE ( 'NONE', #9167, #10678, #5893, .T. ) ;
#3637=ORIENTED_EDGE ( 'NONE', *, *, #27273, .F. ) ;
#3647=FACE_OUTER_BOUND ( 'NONE', #28052, .T. ) ;
#3651=CARTESIAN_POINT ( 'NONE',  ( -189.8086322075389774, 92.49158130768422836, 12.99999999999999822 ) ) ;
#3653=CARTESIAN_POINT ( 'NONE',  ( -63.57415822541634043, -23.01420295945612082, 100.0000000000000000 ) ) ;
#3654=DIRECTION ( 'NONE',  ( 1.000000000000000000, 0.000000000000000000, 0.000000000000000000 ) ) ;
#3657=CARTESIAN_POINT ( 'NONE',  ( 65.00000000000000000, -120.0000000000000995, -69.99999999999998579 ) ) ;
#3658=CARTESIAN_POINT ( 'NONE',  ( -217.7467898461132449, 60.55642267084816410, -12.19614748119898806 ) ) ;
#3659=FACE_OUTER_BOUND ( 'NONE', #19649, .T. ) ;
#3671=CIRCLE ( 'NONE', #5973, 9.999999999999982236 ) ;
#3676=ORIENTED_EDGE ( 'NONE', *, *, #9940, .T. ) ;
#3678=CARTESIAN_POINT ( 'NONE',  ( -77.62175523848470959, 136.2553702788594592, 13.51932229135349495 ) ) ;
#3680=EDGE_CURVE ( 'NONE', #18978, #12426, #15550, .T. ) ;
#3683=CARTESIAN_POINT ( 'NONE',  ( 113.0497540245548009, 225.0442599269872233, 97.19889357486866288 ) ) ;
#3685=CARTESIAN_POINT ( 'NONE',  ( -137.5548842902434501, 129.0090337181558482, -15.70719399148576301 ) ) ;
#3688=CARTESIAN_POINT ( 'NONE',  ( 29.35687238133360211, -42.92577930318808654, 99.85888104713946234 ) ) ;
#3689=CARTESIAN_POINT ( 'NONE',  ( -229.0218807171185631, 91.25446205539969924, -13.22975565712915191 ) ) ;
#3693=DIRECTION ( 'NONE',  ( -0.000000000000000000, 1.000000000000000000, -1.387778780781445429E-16 ) ) ;
#3694=CARTESIAN_POINT ( 'NONE',  ( -37.82257053376181233, 71.03850157808263077, 99.00000000000000000 ) ) ;
#3703=CARTESIAN_POINT ( 'NONE',  ( 103.5789823554392655, 245.2557385300870862, -18.86932834261562064 ) ) ;
#3706=VERTEX_POINT ( 'NONE', #20016 ) ;
#3709=EDGE_CURVE ( 'NONE', #11369, #20037, #10498, .T. ) ;
#3714=VECTOR ( 'NONE', #24271, 1000.000000000000000 ) ;
#3715=CYLINDRICAL_SURFACE ( 'NONE', #1357, 5.000000000000004441 ) ;
#3722=CARTESIAN_POINT ( 'NONE',  ( -207.5108889574473494, 75.59417117316073131, -44.26576816510100798 ) ) ;
#3723=AXIS2_PLACEMENT_3D ( 'NONE', #20491, #11610, #22797 ) ;
#3730=CARTESIAN_POINT ( 'NONE',  ( -201.6781708543087461, 93.98296363999494929, 30.47827602183687290 ) ) ;
#3731=CONICAL_SURFACE ( 'NONE', #23475, 14.64217782292691261, 0.08885387018394190484 ) ;
#3732=DIRECTION ( 'NONE',  ( 1.000000000000000000, 0.000000000000000000, 0.000000000000000000 ) ) ;
#3733=ORIENTED_EDGE ( 'NONE', *, *, #13882, .T. ) ;
#3739=CARTESIAN_POINT ( 'NONE',  ( 96.92716526681839184, 115.1868982021709229, 100.0000000000216573 ) ) ;
#3748=CARTESIAN_POINT ( 'NONE',  ( 109.6721745451680334, 96.60743919220468001, 100.0000000000000142 ) ) ;
#3752=CYLINDRICAL_SURFACE ( 'NONE', #22641, 49.99999999999998579 ) ;
#3753=EDGE_CURVE ( 'NONE', #2370, #22168, #26540, .T. ) ;
#3755=CARTESIAN_POINT ( 'NONE',  ( -175.8417606860892874, 246.9430296707336652, 15.00000000000000000 ) ) ;
#3760=ADVANCED_FACE ( 'NONE', ( #1050 ), #20725, .F. ) ;
#3762=CARTESIAN_POINT ( 'NONE',  ( -188.6733706988670463, 104.1136723946300577, -32.77950115724235047 ) ) ;
#3763=ORIENTED_EDGE ( 'NONE', *, *, #4876, .F. ) ;
#3765=ADVANCED_FACE ( 'NONE', ( #774 ), #3057, .F. ) ;
#3769=ORIENTED_EDGE ( 'NONE', *, *, #15701, .F. ) ;
#3774=CARTESIAN_POINT ( 'NONE',  ( -33.99100231024505803, 128.1996048026844903, -17.41651714595930045 ) ) ;
#3775=CARTESIAN_POINT ( 'NONE',  ( -227.7254947214920264, 90.48960550153041993, 13.48035701177004597 ) ) ;
#3776=ORIENTED_EDGE ( 'NONE', *, *, #22140, .F. ) ;
#3777=DIRECTION ( 'NONE',  ( 0.000000000000000000, 0.000000000000000000, -1.000000000000000000 ) ) ;
#3778=CYLINDRICAL_SURFACE ( 'NONE', #23068, 10.00000000000000888 ) ;
#3779=AXIS2_PLACEMENT_3D ( 'NONE', #6616, #19551, #8773 ) ;
#3789=VERTEX_POINT ( 'NONE', #9821 ) ;
#3794=DIRECTION ( 'NONE',  ( 0.000000000000000000, 0.000000000000000000, -1.000000000000000000 ) ) ;
#3796=LINE ( 'NONE', #12586, #21105 ) ;
#3797=CIRCLE ( 'NONE', #19858, 18.46313063346208239 ) ;
#3801=DIRECTION ( 'NONE',  ( 1.000000000000000000, 0.000000000000000000, 0.000000000000000000 ) ) ;
#3802=CARTESIAN_POINT ( 'NONE',  ( -203.1779787704217313, 93.05164332230201296, 28.77272332722132120 ) ) ;
#3803=CARTESIAN_POINT ( 'NONE',  ( -234.1955688336022092, 78.70261838805063803, -15.19002172608862899 ) ) ;
#3807=FACE_OUTER_BOUND ( 'NONE', #2226, .T. ) ;
#3808=CARTESIAN_POINT ( 'NONE',  ( 134.9999999999998579, 220.0000000000000284, -100.0000000000000142 ) ) ;
#3816=CIRCLE ( 'NONE', #19869, 15.26911010665567225 ) ;
#3817=VECTOR ( 'NONE', #13161, 1000.000000000000114 ) ;
#3818=CARTESIAN_POINT ( 'NONE',  ( -233.7137317802251175, 78.16591391987653026, 15.26566376705435069 ) ) ;
#3821=ORIENTED_EDGE ( 'NONE', *, *, #24249, .T. ) ;
#3825=VERTEX_POINT ( 'NONE', #16153 ) ;
#3830=CARTESIAN_POINT ( 'NONE',  ( -151.0466515240400440, 123.3377277206981120, -20.04773851805323659 ) ) ;
#3835=CARTESIAN_POINT ( 'NONE',  ( 18.30893690202339741, -48.84579300681143366, 98.66826089724658289 ) ) ;
#3836=CARTESIAN_POINT ( 'NONE',  ( -231.3914616533584763, 93.02691812379475778, -12.99999999981396215 ) ) ;
#3840=DIRECTION ( 'NONE',  ( -0.000000000000000000, 1.000000000000000000, -1.387778780781445429E-16 ) ) ;
#3846=DIRECTION ( 'NONE',  ( 0.7123733896039575741, 0.6147814225729705262, -0.3384788859638410141 ) ) ;
#3851=CARTESIAN_POINT ( 'NONE',  ( 105.7038310726791650, 247.5990904218954540, -23.20200675068357299 ) ) ;
#3855=ORIENTED_EDGE ( 'NONE', *, *, #2842, .T. ) ;
#3857=AXIS2_PLACEMENT_3D ( 'NONE', #26170, #22295, #15848 ) ;
#3859=ORIENTED_EDGE ( 'NONE', *, *, #7580, .T. ) ;
#3864=DIRECTION ( 'NONE',  ( 1.000000000000000000, 0.000000000000000000, 0.000000000000000000 ) ) ;
#3869=CARTESIAN_POINT ( 'NONE',  ( -208.6543519075750908, 74.78670680337248200, -37.88580841379594233 ) ) ;
#3872=CARTESIAN_POINT ( 'NONE',  ( -26.99706921587402775, 129.1643607319973626, 16.99462959852061772 ) ) ;
#3875=DIRECTION ( 'NONE',  ( 0.000000000000000000, 0.000000000000000000, 1.000000000000000000 ) ) ;
#3876=VECTOR ( 'NONE', #10463, 1000.000000000000000 ) ;
#3878=CARTESIAN_POINT ( 'NONE',  ( 119.9999999999999147, 236.7705098312484893, -100.0000000000000284 ) ) ;
#3883=EDGE_CURVE ( 'NONE', #9161, #18691, #3146, .T. ) ;
#3889=AXIS2_PLACEMENT_3D ( 'NONE', #2416, #21964, #19808 ) ;
#3891=CARTESIAN_POINT ( 'NONE',  ( 79.99999999999991473, 80.00000000000001421, -100.0000000000000142 ) ) ;
#3893=LINE ( 'NONE', #18842, #12982 ) ;
#3896=CARTESIAN_POINT ( 'NONE',  ( 111.0641325991587252, 99.15168937823351314, 100.0000000000000142 ) ) ;
#3897=ORIENTED_EDGE ( 'NONE', *, *, #25902, .F. ) ;
#3898=AXIS2_PLACEMENT_3D ( 'NONE', #73, #1658, #10715 ) ;
#3904=EDGE_CURVE ( 'NONE', #7140, #18691, #16429, .T. ) ;
#3905=EDGE_CURVE ( 'NONE', #9382, #12221, #9402, .T. ) ;
#3916=CARTESIAN_POINT ( 'NONE',  ( -225.0835117808284451, 89.24749510747318482, 14.20199329800427002 ) ) ;
#3918=CARTESIAN_POINT ( 'NONE',  ( -2.081668171172168513E-14, 79.99999999999998579, -70.00000000000001421 ) ) ;
#3919=CIRCLE ( 'NONE', #11278, 2.586968381275096984 ) ;
#3920=VERTEX_POINT ( 'NONE', #25459 ) ;
#3924=CARTESIAN_POINT ( 'NONE',  ( -167.4464202405217463, 116.4377010620362967, -25.83866841605921749 ) ) ;
#3925=ORIENTED_EDGE ( 'NONE', *, *, #13099, .F. ) ;
#3930=CIRCLE ( 'NONE', #8536, 16.46313063346208239 ) ;
#3932=ORIENTED_EDGE ( 'NONE', *, *, #5069, .T. ) ;
#3933=EDGE_LOOP ( 'NONE', ( #14131, #3253, #17856, #19936 ) ) ;
#3936=CARTESIAN_POINT ( 'NONE',  ( 4.491205691019747093, 138.9213844498120238, 13.09540051078805156 ) ) ;
#3937=CYLINDRICAL_SURFACE ( 'NONE', #11944, 70.83858790703926900 ) ;
#3938=AXIS2_PLACEMENT_3D ( 'NONE', #18516, #5292, #13795 ) ;
#3939=DIRECTION ( 'NONE',  ( 0.000000000000000000, 0.000000000000000000, 1.000000000000000000 ) ) ;
#3940=FACE_OUTER_BOUND ( 'NONE', #665, .T. ) ;
#3941=CARTESIAN_POINT ( 'NONE',  ( -229.6735579984113258, 64.27833679895920227, -7.258985754582258920 ) ) ;
#3945=CARTESIAN_POINT ( 'NONE',  ( -180.0000000000000284, -40.00000000000004974, -70.00000000000001421 ) ) ;
#3948=LINE ( 'NONE', #6110, #6810 ) ;
#3954=ORIENTED_EDGE ( 'NONE', *, *, #22390, .F. ) ;
#3955=CIRCLE ( 'NONE', #1214, 14.64217782292691261 ) ;
#3961=EDGE_CURVE ( 'NONE', #8160, #3252, #16412, .T. ) ;
#3963=EDGE_CURVE ( 'NONE', #366, #2661, #1269, .T. ) ;
#3964=CARTESIAN_POINT ( 'NONE',  ( -67.54154682840413670, 135.5235962012238815, 15.28890748345223116 ) ) ;
#3967=FACE_OUTER_BOUND ( 'NONE', #3029, .T. ) ;
#3968=CARTESIAN_POINT ( 'NONE',  ( -160.0000000000000284, 119.7660240611718905, -22.85081902853004721 ) ) ;
#3970=CARTESIAN_POINT ( 'NONE',  ( -127.6926693028035089, 131.7039880331085158, -16.10276958539054704 ) ) ;
#3971=VECTOR ( 'NONE', #11595, 1000.000000000000000 ) ;
#3974=CARTESIAN_POINT ( 'NONE',  ( -221.8631419436352985, 88.28315383663137084, -15.48010842192074854 ) ) ;
#3976=CARTESIAN_POINT ( 'NONE',  ( -228.3351344443410653, 88.50822704663181639, 15.59479036512446370 ) ) ;
#3977=FACE_OUTER_BOUND ( 'NONE', #18018, .T. ) ;
#3978=DIRECTION ( 'NONE',  ( 0.000000000000000000, 0.000000000000000000, 1.000000000000000000 ) ) ;
#3979=DIRECTION ( 'NONE',  ( 0.000000000000000000, -0.000000000000000000, -1.000000000000000000 ) ) ;
#3981=EDGE_CURVE ( 'NONE', #10749, #23784, #18763, .T. ) ;
#3984=B_SPLINE_CURVE_WITH_KNOTS ( 'NONE', 3,
 ( #12540, #6478, #10654, #21713, #2024, #10799, #19556, #8641, #1457, #5909, #14684, #21280, #10370, #27868, #8211, #14833, #16976, #6052, #23584, #21421, #1735, #10511, #2734, #19978, #2590, #17535 ),
 .UNSPECIFIED., .F., .F.,
 ( 4, 2, 2, 2, 2, 2, 2, 2, 2, 2, 2, 2, 4 ),
 ( 0.000000000000000000, 0.006543047306792185158, 0.01308609461358437032, 0.01962914192037655201, 0.02617218922716874063, 0.02944371288056481933, 0.03107947470726283787, 0.03271523653396085640, 0.03598676018735695592, 0.03925828384075306238, 0.04580133114754529611, 0.04907285480094141644, 0.05234437845433753678 ),
 .UNSPECIFIED. ) ;
#3985=CARTESIAN_POINT ( 'NONE',  ( -112.3221550338875687, 22.24192588826928585, 83.00000000000001421 ) ) ;
#3986=VERTEX_POINT ( 'NONE', #27878 ) ;
#3988=CARTESIAN_POINT ( 'NONE',  ( 99.07849735471324948, 234.2556710009628489, -21.83147064533557113 ) ) ;
#3989=EDGE_LOOP ( 'NONE', ( #578, #18448, #17971 ) ) ;
#3992=AXIS2_PLACEMENT_3D ( 'NONE', #6903, #871, #15832 ) ;
#3993=ORIENTED_EDGE ( 'NONE', *, *, #11307, .F. ) ;
#3994=EDGE_CURVE ( 'NONE', #5384, #18983, #8612, .T. ) ;
#3999=EDGE_LOOP ( 'NONE', ( #6471, #2426, #10047, #5403 ) ) ;
#4000=EDGE_LOOP ( 'NONE', ( #13487, #12109, #8141 ) ) ;
#4001=LINE ( 'NONE', #12785, #9068 ) ;
#4008=CARTESIAN_POINT ( 'NONE',  ( -234.3956316663174277, 78.94038675297558427, -15.16326400926280904 ) ) ;
#4009=CARTESIAN_POINT ( 'NONE',  ( -31.62490448008894361, 128.0247143377008285, 17.49372955826459020 ) ) ;
#4012=FACE_OUTER_BOUND ( 'NONE', #25102, .T. ) ;
#4014=CARTESIAN_POINT ( 'NONE',  ( 134.9999999999998579, -327.2004514666934369, 84.99999999999995737 ) ) ;
#4023=CARTESIAN_POINT ( 'NONE',  ( 117.1152841538673073, 116.0550883417529207, 100.0000000000000142 ) ) ;
#4029=CARTESIAN_POINT ( 'NONE',  ( 85.90765579568754617, 110.5723347145559785, -100.0000000000000284 ) ) ;
#4031=CARTESIAN_POINT ( 'NONE',  ( 96.79688798037243203, 232.6553591674251606, 20.12433470795689772 ) ) ;
#4034=CARTESIAN_POINT ( 'NONE',  ( -228.1057710792337616, 90.70189914778829632, 15.47288924712567848 ) ) ;
#4038=DIRECTION ( 'NONE',  ( 1.000000000000000000, -0.000000000000000000, 0.000000000000000000 ) ) ;
#4043=CARTESIAN_POINT ( 'NONE',  ( -12.24491960465745599, 24.64876300893806160, 95.00000000000000000 ) ) ;
#4045=CARTESIAN_POINT ( 'NONE',  ( -140.1213116003368668, 122.5384136796733827, 12.99999999999999822 ) ) ;
#4047=DIRECTION ( 'NONE',  ( -0.000000000000000000, 1.000000000000000000, -1.387778780781445429E-16 ) ) ;
#4050=ADVANCED_FACE ( 'NONE', ( #25880 ), #11371, .F. ) ;
#4053=CARTESIAN_POINT ( 'NONE',  ( -205.8189311304054172, 91.09162128824407034, 26.99035118652719589 ) ) ;
#4054=VERTEX_POINT ( 'NONE', #10946 ) ;
#4057=ORIENTED_EDGE ( 'NONE', *, *, #240, .F. ) ;
#4060=CARTESIAN_POINT ( 'NONE',  ( -178.8230272009045336, 110.7367001878539270, -29.27854200063107015 ) ) ;
#4061=EDGE_LOOP ( 'NONE', ( #18002, #23361 ) ) ;
#4062=ORIENTED_EDGE ( 'NONE', *, *, #13766, .T. ) ;
#4069=AXIS2_PLACEMENT_3D ( 'NONE', #7938, #8079, #25321 ) ;
#4072=CARTESIAN_POINT ( 'NONE',  ( -68.57415822541635464, 75.97823757117562593, 100.0000000000000000 ) ) ;
#4074=DIRECTION ( 'NONE',  ( -1.000000000000000000, 0.000000000000000000, 0.000000000000000000 ) ) ;
#4079=DIRECTION ( 'NONE',  ( -0.000000000000000000, 1.000000000000000000, -1.387778780781445429E-16 ) ) ;
#4080=CARTESIAN_POINT ( 'NONE',  ( -242.2202452114001971, 73.32912780460810609, -5.047888127322691432 ) ) ;
#4081=VERTEX_POINT ( 'NONE', #17261 ) ;
#4083=AXIS2_PLACEMENT_3D ( 'NONE', #26593, #22151, #22005 ) ;
#4088=CARTESIAN_POINT ( 'NONE',  ( 113.0677398990926150, 225.0479495651688069, -97.20864094219261631 ) ) ;
#4097=VERTEX_POINT ( 'NONE', #5039 ) ;
#4107=CIRCLE ( 'NONE', #16068, 21.20097097723064294 ) ;
#4108=ORIENTED_EDGE ( 'NONE', *, *, #20852, .T. ) ;
#4111=CARTESIAN_POINT ( 'NONE',  ( -279.3160071107327553, -77.04550865309217045, 0.000000000000000000 ) ) ;
#4113=CARTESIAN_POINT ( 'NONE',  ( -160.0000000000000284, 119.7660240611718763, -22.85081902853004365 ) ) ;
#4116=CARTESIAN_POINT ( 'NONE',  ( 20.31647538124909502, -48.17530653888324821, 98.86525827369392516 ) ) ;
#4117=CARTESIAN_POINT ( 'NONE',  ( -218.7452477155994757, 87.82940237244157800, -19.01335168521931607 ) ) ;
#4121=DIRECTION ( 'NONE',  ( -4.625929269271483942E-16, 1.000000000000000000, 0.000000000000000000 ) ) ;
#4122=EDGE_CURVE ( 'NONE', #15118, #28119, #4993, .T. ) ;
#4123=EDGE_LOOP ( 'NONE', ( #16163, #3080, #25060, #14868 ) ) ;
#4124=EDGE_CURVE ( 'NONE', #27076, #2661, #15980, .T. ) ;
#4125=AXIS2_PLACEMENT_3D ( 'NONE', #18888, #5679, #3654 ) ;
#4127=DIRECTION ( 'NONE',  ( 0.000000000000000000, -1.000000000000000000, 0.000000000000000000 ) ) ;
#4128=ADVANCED_FACE ( 'NONE', ( #26883 ), #18265, .F. ) ;
#4133=CARTESIAN_POINT ( 'NONE',  ( 106.3805259670840258, 243.6561646000984922, -30.69292865457993713 ) ) ;
#4134=EDGE_LOOP ( 'NONE', ( #23618, #19022, #185, #24923, #8663, #16702, #28248, #7472 ) ) ;
#4135=CARTESIAN_POINT ( 'NONE',  ( -8.491711918032281758, 132.4972918898329226, -14.40622109717888755 ) ) ;
#4137=ORIENTED_EDGE ( 'NONE', *, *, #9940, .F. ) ;
#4139=ORIENTED_EDGE ( 'NONE', *, *, #19725, .F. ) ;
#4141=DIRECTION ( 'NONE',  ( -0.000000000000000000, 0.000000000000000000, 1.000000000000000000 ) ) ;
#4143=B_SPLINE_CURVE_WITH_KNOTS ( 'NONE', 3,
 ( #28178, #8523, #17275, #3774, #12563, #4195, #16994, #21110, #8042, #1006, #14800, #16671, #23132, #10202, #5880, #9923, #18961, #10340, #20970, #25423, #23556, #8182 ),
 .UNSPECIFIED., .F., .F.,
 ( 4, 2, 2, 2, 2, 2, 2, 2, 2, 2, 4 ),
 ( 0.000000000000000000, 0.006853915506645740473, 0.01370783101329148095, 0.01713478876661434641, 0.02056174651993721014, 0.02741566202658293067, 0.03426957753322865119, 0.03769653528655152186, 0.04112349303987439253, 0.04797740854652013387, 0.05483132405316587521 ),
 .UNSPECIFIED. ) ;
#4144=CARTESIAN_POINT ( 'NONE',  ( -412.2374841615667833, -120.0000000000002842, -100.0000000000000142 ) ) ;
#4147=LINE ( 'NONE', #21831, #3423 ) ;
#4148=ADVANCED_FACE ( 'NONE', ( #7206 ), #9647, .T. ) ;
#4155=CARTESIAN_POINT ( 'NONE',  ( -248.1546605714623013, -91.18033988749901653, 0.000000000000000000 ) ) ;
#4159=CARTESIAN_POINT ( 'NONE',  ( -175.3965446499522045, 112.7547980845980646, 27.84039695627248889 ) ) ;
#4164=ORIENTED_EDGE ( 'NONE', *, *, #21247, .F. ) ;
#4167=CARTESIAN_POINT ( 'NONE',  ( -215.4886702565632390, 139.8420026707766226, -13.00000000000000000 ) ) ;
#4168=DIRECTION ( 'NONE',  ( 0.000000000000000000, 0.000000000000000000, -1.000000000000000000 ) ) ;
#4169=ORIENTED_EDGE ( 'NONE', *, *, #11206, .F. ) ;
#4170=ORIENTED_EDGE ( 'NONE', *, *, #21490, .T. ) ;
#4171=CARTESIAN_POINT ( 'NONE',  ( 118.9718481642231609, 125.5986290015685398, -100.0000000000000142 ) ) ;
#4173=DIRECTION ( 'NONE',  ( 2.312964634635742464E-16, -1.000000000000000000, 0.000000000000000000 ) ) ;
#4174=ORIENTED_EDGE ( 'NONE', *, *, #1814, .T. ) ;
#4175=CARTESIAN_POINT ( 'NONE',  ( -228.1203047800660215, 90.71301417736495409, 13.39797158503563779 ) ) ;
#4180=FACE_OUTER_BOUND ( 'NONE', #9917, .T. ) ;
#4185=AXIS2_PLACEMENT_3D ( 'NONE', #10009, #16064, #22666 ) ;
#4186=VERTEX_POINT ( 'NONE', #22720 ) ;
#4188=ADVANCED_FACE ( 'NONE', ( #3023 ), #11810, .F. ) ;
#4193=DIRECTION ( 'NONE',  ( 1.000000000000000000, 0.000000000000000000, -0.000000000000000000 ) ) ;
#4194=DIRECTION ( 'NONE',  ( 0.000000000000000000, 1.000000000000000000, 0.000000000000000000 ) ) ;
#4195=CARTESIAN_POINT ( 'NONE',  ( -28.28141033279510808, 127.9583036527814386, -17.52276859028009071 ) ) ;
#4196=CARTESIAN_POINT ( 'NONE',  ( -221.0638194754022265, 88.12640624682363466, 15.86102591047146682 ) ) ;
#4203=CARTESIAN_POINT ( 'NONE',  ( -162.6948170962391487, 119.3828354928103579, -22.14444076542767448 ) ) ;
#4211=DIRECTION ( 'NONE',  ( -1.000000000000000000, -1.530283246943720875E-16, 0.000000000000000000 ) ) ;
#4213=EDGE_CURVE ( 'NONE', #11481, #18743, #6304, .T. ) ;
#4217=LINE ( 'NONE', #10978, #3454 ) ;
#4219=LINE ( 'NONE', #28337, #6670 ) ;
#4220=( BOUNDED_CURVE ( )  B_SPLINE_CURVE ( 2, ( #23313, #19002, #12695 ),
 .UNSPECIFIED., .F., .F. ) 
 B_SPLINE_CURVE_WITH_KNOTS ( ( 3, 3 ),
 ( 0.000000000000000000, 1.000000000000000000 ),
 .UNSPECIFIED. ) 
 CURVE ( )  GEOMETRIC_REPRESENTATION_ITEM ( )  RATIONAL_B_SPLINE_CURVE ( ( 1.000000000000000000, 0.7071067811865475727, 1.000000000000000000 ) ) 
 REPRESENTATION_ITEM ( '' )  );
#4222=DIRECTION ( 'NONE',  ( -1.000000000000000000, 0.000000000000000000, 0.000000000000000000 ) ) ;
#4223=CARTESIAN_POINT ( 'NONE',  ( -244.5479615644635487, 75.99513337129094737, -15.00000000000000178 ) ) ;
#4224=VERTEX_POINT ( 'NONE', #9789 ) ;
#4225=AXIS2_PLACEMENT_3D ( 'NONE', #23564, #16540, #23144 ) ;
#4229=AXIS2_PLACEMENT_3D ( 'NONE', #20054, #2812, #22216 ) ;
#4233=CIRCLE ( 'NONE', #19841, 2.000000000000000000 ) ;
#4234=EDGE_CURVE ( 'NONE', #19021, #6913, #2178, .T. ) ;
#4238=CARTESIAN_POINT ( 'NONE',  ( 109.9999999999999147, 140.0000000000000000, 90.00000000000002842 ) ) ;
#4240=ORIENTED_EDGE ( 'NONE', *, *, #22065, .F. ) ;
#4252=AXIS2_PLACEMENT_3D ( 'NONE', #8758, #15519, #15233 ) ;
#4253=CARTESIAN_POINT ( 'NONE',  ( -222.2072112174627136, 138.1987073436359026, 14.97424725141359403 ) ) ;
#4254=DIRECTION ( 'NONE',  ( 0.000000000000000000, 0.000000000000000000, 1.000000000000000000 ) ) ;
#4262=CARTESIAN_POINT ( 'NONE',  ( -218.2708698084869638, 86.23473497505111141, -19.67429589792924816 ) ) ;
#4265=FACE_OUTER_BOUND ( 'NONE', #6382, .T. ) ;
#4277=AXIS2_PLACEMENT_3D ( 'NONE', #2108, #4121, #23959 ) ;
#4279=CARTESIAN_POINT ( 'NONE',  ( 93.26488863019004327, 240.2518291191186393, -7.855680688305695547 ) ) ;
#4292=CARTESIAN_POINT ( 'NONE',  ( -107.3221550338875687, 17.24192588826928585, 80.00000000000001421 ) ) ;
#4294=AXIS2_PLACEMENT_3D ( 'NONE', #24629, #6806, #15451 ) ;
#4296=CARTESIAN_POINT ( 'NONE',  ( -175.0000000000000000, -150.0000000000000853, -64.00000000000000000 ) ) ;
#4298=CARTESIAN_POINT ( 'NONE',  ( -119.0030847931093518, 214.2064521616283059, -5.000000000000004441 ) ) ;
#4299=CYLINDRICAL_SURFACE ( 'NONE', #26365, 16.07743405327025243 ) ;
#4301=CARTESIAN_POINT ( 'NONE',  ( -189.8086322075389774, 92.49158130768422836, 15.00000000000000000 ) ) ;
#4302=DIRECTION ( 'NONE',  ( 0.000000000000000000, 1.000000000000000000, 0.000000000000000000 ) ) ;
#4305=CARTESIAN_POINT ( 'NONE',  ( 65.00000000000000000, -120.0000000000000711, 70.00000000000001421 ) ) ;
#4307=EDGE_LOOP ( 'NONE', ( #22135, #22842, #7042, #20194 ) ) ;
#4309=CARTESIAN_POINT ( 'NONE',  ( -167.4985236603498038, 116.4129322153221437, 25.86027712211474494 ) ) ;
#4311=EDGE_LOOP ( 'NONE', ( #15283, #10947, #2895, #12145 ) ) ;
#4315=DIRECTION ( 'NONE',  ( 1.000000000000000000, 0.000000000000000000, 0.000000000000000000 ) ) ;
#4317=ORIENTED_EDGE ( 'NONE', *, *, #6465, .T. ) ;
#4318=CARTESIAN_POINT ( 'NONE',  ( 119.9999999987673220, 136.1131920016294714, -100.0000000000000142 ) ) ;
#4319=EDGE_CURVE ( 'NONE', #14508, #3426, #22993, .T. ) ;
#4320=CARTESIAN_POINT ( 'NONE',  ( 93.99999999999985789, 268.4896896257338312, 84.99999999999995737 ) ) ;
#4321=VERTEX_POINT ( 'NONE', #25284 ) ;
#4322=CARTESIAN_POINT ( 'NONE',  ( -221.9429674677837170, 88.28884742766322802, 17.46146441898723722 ) ) ;
#4326=CIRCLE ( 'NONE', #24074, 6.000000000000005329 ) ;
#4331=ADVANCED_FACE ( 'NONE', ( #14521 ), #21113, .F. ) ;
#4335=ORIENTED_EDGE ( 'NONE', *, *, #16804, .F. ) ;
#4336=DIRECTION ( 'NONE',  ( 0.000000000000000000, 0.000000000000000000, 1.000000000000000000 ) ) ;
#4338=DIRECTION ( 'NONE',  ( -0.000000000000000000, -0.000000000000000000, -1.000000000000000000 ) ) ;
#4339=CARTESIAN_POINT ( 'NONE',  ( -213.5112655984951857, 88.12920823218718169, 20.63189810804927049 ) ) ;
#4344=CARTESIAN_POINT ( 'NONE',  ( -184.0646120581192520, 107.4357226780370667, -31.54942295155680654 ) ) ;
#4347=CONICAL_SURFACE ( 'NONE', #11258, 6.025000000000002132, 0.7853981633974482790 ) ;
#4349=EDGE_CURVE ( 'NONE', #5984, #15146, #24737, .T. ) ;
#4361=AXIS2_PLACEMENT_3D ( 'NONE', #24230, #11163, #26511 ) ;
#4362=CARTESIAN_POINT ( 'NONE',  ( -209.9870472515087840, 61.15599310541787048, -23.95647182577626921 ) ) ;
#4366=VECTOR ( 'NONE', #19997, 1000.000000000000000 ) ;
#4372=DIRECTION ( 'NONE',  ( 1.000000000000000000, 0.000000000000000000, 0.000000000000000000 ) ) ;
#4374=CYLINDRICAL_SURFACE ( 'NONE', #3898, 2.586968381275096984 ) ;
#4376=CARTESIAN_POINT ( 'NONE',  ( -180.0000000000000284, 59.99999999999994316, -100.0000000000000142 ) ) ;
#4379=CARTESIAN_POINT ( 'NONE',  ( -207.5044420441007560, 75.59897387903042443, 45.00000000000000000 ) ) ;
#4385=CIRCLE ( 'NONE', #20452, 30.00000000000002842 ) ;
#4390=( BOUNDED_SURFACE ( )  B_SPLINE_SURFACE ( 3, 2, ( 
 ( #9631, #2118, #17069 ),
 ( #6009, #12916, #28387 ),
 ( #19226, #26107, #28257 ),
 ( #4279, #23967, #10895 ),
 ( #1978, #17213, #6437 ),
 ( #25830, #12639, #1697 ),
 ( #21380, #25972, #12777 ),
 ( #23683, #19650, #10468 ),
 ( #21520, #17347, #27971 ),
 ( #19512, #8315, #10755 ),
 ( #15213, #13065, #6156 ),
 ( #8735, #25688, #14929 ),
 ( #10609, #14784, #3988 ),
 ( #21811, #1559, #14641 ),
 ( #17488, #5864, #23395 ),
 ( #3703, #12494, #6288 ),
 ( #15066, #21238, #23542 ),
 ( #3851, #1834, #19366 ),
 ( #10325, #27829, #28116 ),
 ( #8457, #23825, #4133 ),
 ( #21663, #8167, #8597 ),
 ( #19087, #16931, #15639 ),
 ( #21945, #24243, #26525 ),
 ( #22087, #544, #17921 ),
 ( #9309, #11622, #11178 ),
 ( #4415, #6856, #2827 ),
 ( #4693, #18072, #11475 ),
 ( #15786, #24529, #2254 ),
 ( #15357, #22523, #4839 ),
 ( #20364, #9021, #9457 ) ),
 .UNSPECIFIED., .F., .F., .F. ) 
 B_SPLINE_SURFACE_WITH_KNOTS ( ( 4, 2, 2, 2, 2, 2, 2, 2, 2, 2, 2, 2, 2, 2, 4 ),
 ( 3, 3 ),
 ( 0.000000000000000000, 0.003854887539719038109, 0.007709775079438076217, 0.009637218849297595272, 0.01156466261915711433, 0.01541955015887615243, 0.01927443769859519054, 0.02312932523831422865, 0.03083910031775230487, 0.03469398785747133951, 0.03854887539719038109, 0.04625865047662845730, 0.05396842555606653352, 0.05782331309578557510, 0.06167820063550460974 ),
 ( 0.000000000000000000, 1.000000000000000000 ),
 .UNSPECIFIED. ) 
 GEOMETRIC_REPRESENTATION_ITEM ( )  RATIONAL_B_SPLINE_SURFACE ( (
 ( 1.000000000000000000, 0.7071067811865491270, 1.000000000000000000),
 ( 1.000000000000000000, 0.7108376764369856993, 1.000000000000000000),
 ( 1.000000000000000000, 0.7158505121285758666, 1.000000000000000000),
 ( 1.000000000000000000, 0.7278978148825536731, 1.000000000000000000),
 ( 1.000000000000000000, 0.7349313210304360133, 1.000000000000000000),
 ( 1.000000000000000000, 0.7466216138177209638, 1.000000000000000000),
 ( 1.000000000000000000, 0.7507087799372132997, 1.000000000000000000),
 ( 1.000000000000000000, 0.7592063458283927480, 1.000000000000000000),
 ( 1.000000000000000000, 0.7635836989921321871, 1.000000000000000000),
 ( 1.000000000000000000, 0.7769550404251118758, 1.000000000000000000),
 ( 1.000000000000000000, 0.7862062597111377782, 1.000000000000000000),
 ( 1.000000000000000000, 0.8049739164093935306, 1.000000000000000000),
 ( 1.000000000000000000, 0.8144916847802230464, 1.000000000000000000),
 ( 1.000000000000000000, 0.8334855532645426557, 1.000000000000000000),
 ( 1.000000000000000000, 0.8428380035006605153, 1.000000000000000000),
 ( 1.000000000000000000, 0.8700856926957447612, 1.000000000000000000),
 ( 1.000000000000000000, 0.8872021369645698430, 1.000000000000000000),
 ( 1.000000000000000000, 0.9106340391013421076, 1.000000000000000000),
 ( 1.000000000000000000, 0.9180764524644583480, 1.000000000000000000),
 ( 1.000000000000000000, 0.9321377268945353345, 1.000000000000000000),
 ( 1.000000000000000000, 0.9386792981684866088, 1.000000000000000000),
 ( 1.000000000000000000, 0.9568359836574985566, 1.000000000000000000),
 ( 1.000000000000000000, 0.9669855263606685902, 1.000000000000000000),
 ( 1.000000000000000000, 0.9833405099237995106, 1.000000000000000000),
 ( 1.000000000000000000, 0.9895476861107730393, 1.000000000000000000),
 ( 1.000000000000000000, 0.9958061391666522821, 1.000000000000000000),
 ( 1.000000000000000000, 0.9973811977640341109, 1.000000000000000000),
 ( 1.000000000000000000, 0.9994757700714922422, 1.000000000000000000),
 ( 1.000000000000000000, 1.000000000000000000, 1.000000000000000000),
 ( 1.000000000000000000, 1.000000000000000000, 1.000000000000000000) ) ) 
 REPRESENTATION_ITEM ( '' )  SURFACE ( )  );
#4393=FACE_OUTER_BOUND ( 'NONE', #2591, .T. ) ;
#4394=CARTESIAN_POINT ( 'NONE',  ( 89.77759941121971110, 81.13568025368125802, 100.0000000000000142 ) ) ;
#4395=CARTESIAN_POINT ( 'NONE',  ( 106.7826897485233815, 249.1041097334432948, 25.92390487273943123 ) ) ;
#4399=LINE ( 'NONE', #26236, #714 ) ;
#4400=CARTESIAN_POINT ( 'NONE',  ( -210.7172313291012529, 103.7585653882801182, 15.00000000000000000 ) ) ;
#4407=VERTEX_POINT ( 'NONE', #136 ) ;
#4409=DIRECTION ( 'NONE',  ( -0.000000000000000000, 0.000000000000000000, 1.000000000000000000 ) ) ;
#4412=AXIS2_PLACEMENT_3D ( 'NONE', #6565, #19497, #24098 ) ;
#4415=CARTESIAN_POINT ( 'NONE',  ( 109.8079904624971590, 257.1776683528169656, -40.10892953523403293 ) ) ;
#4416=ORIENTED_EDGE ( 'NONE', *, *, #6558, .T. ) ;
#4418=ORIENTED_EDGE ( 'NONE', *, *, #17562, .T. ) ;
#4423=CIRCLE ( 'NONE', #1679, 7.499999999999992895 ) ;
#4428=FACE_OUTER_BOUND ( 'NONE', #14961, .T. ) ;
#4429=CARTESIAN_POINT ( 'NONE',  ( -215.5934637701523684, 59.01440814108518396, 29.65465734991407132 ) ) ;
#4432=CARTESIAN_POINT ( 'NONE',  ( -68.57415822541635464, 29.64876300893806516, 100.0000000000000000 ) ) ;
#4435=DIRECTION ( 'NONE',  ( 1.000000000000000000, -0.000000000000000000, -0.000000000000000000 ) ) ;
#4438=CARTESIAN_POINT ( 'NONE',  ( -33.80003448231774854, 129.4040373687968497, 16.90087253816493273 ) ) ;
#4440=DIRECTION ( 'NONE',  ( 1.530283246943720875E-16, -1.000000000000000000, 0.000000000000000000 ) ) ;
#4445=CARTESIAN_POINT ( 'NONE',  ( -229.9492672981298824, 89.43170946566928592, -15.28058751945465410 ) ) ;
#4448=EDGE_CURVE ( 'NONE', #20275, #1752, #28332, .T. ) ;
#4450=ORIENTED_EDGE ( 'NONE', *, *, #24237, .F. ) ;
#4454=CARTESIAN_POINT ( 'NONE',  ( 117.1152841538456926, 116.0550883417529491, -100.0000000000000142 ) ) ;
#4457=CARTESIAN_POINT ( 'NONE',  ( -218.7796873555838033, 87.80254006751567886, 18.97549214882609903 ) ) ;
#4459=LINE ( 'NONE', #19982, #1074 ) ;
#4463=FACE_OUTER_BOUND ( 'NONE', #3499, .T. ) ;
#4464=CARTESIAN_POINT ( 'NONE',  ( -225.3736415174480214, 135.7651958811098325, -14.97905406095859959 ) ) ;
#4465=DIRECTION ( 'NONE',  ( 0.000000000000000000, 0.000000000000000000, -1.000000000000000000 ) ) ;
#4466=CARTESIAN_POINT ( 'NONE',  ( -235.6837214056122036, 120.7228219557777180, -13.00000000000000000 ) ) ;
#4469=DIRECTION ( 'NONE',  ( 1.000000000000000000, 0.000000000000000000, -0.000000000000000000 ) ) ;
#4470=EDGE_CURVE ( 'NONE', #20648, #6227, #15514, .T. ) ;
#4472=CARTESIAN_POINT ( 'NONE',  ( 145.9999999999998863, 220.0000000000000284, 99.00000000000001421 ) ) ;
#4478=CARTESIAN_POINT ( 'NONE',  ( -180.2001402660981455, 109.5948180456561261, -30.90938774632539321 ) ) ;
#4480=EDGE_LOOP ( 'NONE', ( #1026, #25485, #16593, #3220, #23899, #183, #955, #22157 ) ) ;
#4481=DIRECTION ( 'NONE',  ( -0.7343588774761952154, 0.6787614006938686995, 0.000000000000000000 ) ) ;
#4482=LINE ( 'NONE', #193, #18066 ) ;
#4486=CARTESIAN_POINT ( 'NONE',  ( -27.06101787524987401, 127.9652732746794044, 17.51969639969995995 ) ) ;
#4489=LINE ( 'NONE', #23763, #25938 ) ;
#4493=CARTESIAN_POINT ( 'NONE',  ( -196.7918453702777128, 80.49308115506423178, 248.5795775865965993 ) ) ;
#4497=CARTESIAN_POINT ( 'NONE',  ( -205.1370039499190625, 144.1304017549904586, -13.00000000000000000 ) ) ;
#4502=ORIENTED_EDGE ( 'NONE', *, *, #9093, .T. ) ;
#4504=CARTESIAN_POINT ( 'NONE',  ( -211.3876077005476759, 59.97725620786452083, 16.20275295307625996 ) ) ;
#4506=ORIENTED_EDGE ( 'NONE', *, *, #27962, .F. ) ;
#4509=CARTESIAN_POINT ( 'NONE',  ( 79.99999999999994316, -70.00000000000002842, 70.00000000000001421 ) ) ;
#4510=DIRECTION ( 'NONE',  ( 0.000000000000000000, 0.000000000000000000, 1.000000000000000000 ) ) ;
#4515=ORIENTED_EDGE ( 'NONE', *, *, #17446, .F. ) ;
#4516=AXIS2_PLACEMENT_3D ( 'NONE', #1651, #10709, #21333 ) ;
#4526=FACE_OUTER_BOUND ( 'NONE', #7222, .T. ) ;
#4527=CARTESIAN_POINT ( 'NONE',  ( 88.44954299047319068, 230.0000000005625225, 16.19779584935177041 ) ) ;
#4532=LINE ( 'NONE', #24093, #4572 ) ;
#4533=AXIS2_PLACEMENT_3D ( 'NONE', #20666, #18523, #20098 ) ;
#4539=CARTESIAN_POINT ( 'NONE',  ( 179.9999999999999147, 330.0000000000000000, -100.0000000000000142 ) ) ;
#4547=ADVANCED_FACE ( 'NONE', ( #16234 ), #13694, .T. ) ;
#4551=ORIENTED_EDGE ( 'NONE', *, *, #18218, .F. ) ;
#4552=VECTOR ( 'NONE', #15618, 1000.000000000000000 ) ;
#4559=AXIS2_PLACEMENT_3D ( 'NONE', #24106, #4409, #11031 ) ;
#4560=EDGE_LOOP ( 'NONE', ( #14387, #3504, #4108, #8676 ) ) ;
#4564=VECTOR ( 'NONE', #13075, 1000.000000000000000 ) ;
#4565=DIRECTION ( 'NONE',  ( 0.000000000000000000, 0.000000000000000000, 1.000000000000000000 ) ) ;
#4568=CARTESIAN_POINT ( 'NONE',  ( -226.8880901706932605, 73.06320664976882995, 17.43415524067561861 ) ) ;
#4570=EDGE_CURVE ( 'NONE', #20676, #27164, #23761, .T. ) ;
#4571=CYLINDRICAL_SURFACE ( 'NONE', #9915, 5.000000000000000888 ) ;
#4572=VECTOR ( 'NONE', #22360, 1000.000000000000000 ) ;
#4574=CARTESIAN_POINT ( 'NONE',  ( 112.4999999999998863, 220.0000000000000284, -105.0000000000000284 ) ) ;
#4576=CARTESIAN_POINT ( 'NONE',  ( 107.3061218092289408, 127.3934823308085242, 87.81249999970602005 ) ) ;
#4578=CARTESIAN_POINT ( 'NONE',  ( -4.279759758627867505, 134.1644510977413915, 13.92782111787041899 ) ) ;
#4579=CARTESIAN_POINT ( 'NONE',  ( -207.9699968406354458, 74.12752936445579621, 42.75546270459319231 ) ) ;
#4584=CARTESIAN_POINT ( 'NONE',  ( -173.3845272153682515, 113.8923293831577013, 27.65784535673404676 ) ) ;
#4585=EDGE_CURVE ( 'NONE', #15391, #14406, #20095, .T. ) ;
#4586=B_SPLINE_CURVE_WITH_KNOTS ( 'NONE', 3,
 ( #27798, #5974, #8564, #23504, #3818, #12604, #25516, #26073, #23360, #24497, #26215, #8839, #20184, #8701, #6542, #21913, #4805, #18035, #26638, #26355, #15324, #6820, #13591, #11438, #22343, #15465, #7115, #225, #17599, #17889, #2651, #13443, #15604, #2217, #11142, #512, #24076, #4379 ),
 .UNSPECIFIED., .F., .F.,
 ( 4, 2, 2, 2, 2, 2, 2, 2, 2, 2, 2, 2, 2, 2, 2, 2, 2, 2, 4 ),
 ( 0.000000000000000000, 0.003119048492555984414, 0.006238096985111968827, 0.007797621231389974261, 0.009357145477667980563, 0.01247619397022393418, 0.01403571821650191620, 0.01559524246277989822, 0.01871429095533593337, 0.02027381520161395528, 0.02183333944789197373, 0.02495238794044801409, 0.03119048492556014684, 0.03742858191067228307, 0.04054763040322835466, 0.04210715464950640086, 0.04366667889578444706, 0.04678572738834055333, 0.04990477588089665961 ),
 .UNSPECIFIED. ) ;
#4588=EDGE_LOOP ( 'NONE', ( #10333, #654 ) ) ;
#4590=ORIENTED_EDGE ( 'NONE', *, *, #22306, .T. ) ;
#4592=CARTESIAN_POINT ( 'NONE',  ( -108.0188924393233947, 135.2207200644698446, 13.71980004753943483 ) ) ;
#4595=LINE ( 'NONE', #13380, #13183 ) ;
#4596=CIRCLE ( 'NONE', #11500, 19.99999999999998934 ) ;
#4598=DIRECTION ( 'NONE',  ( -0.000000000000000000, -0.000000000000000000, -1.000000000000000000 ) ) ;
#4599=EDGE_LOOP ( 'NONE', ( #4952, #27489, #9694, #21317 ) ) ;
#4600=CARTESIAN_POINT ( 'NONE',  ( -208.5124701773697211, 89.65907251580088655, 24.74122501709897293 ) ) ;
#4601=DIRECTION ( 'NONE',  ( 8.673617379884074915E-17, 1.000000000000000000, -0.000000000000000000 ) ) ;
#4603=CARTESIAN_POINT ( 'NONE',  ( 39.99999999999996447, 59.99999999999981526, 100.0000000000000142 ) ) ;
#4607=DIRECTION ( 'NONE',  ( 0.000000000000000000, 0.000000000000000000, -1.000000000000000000 ) ) ;
#4615=DIRECTION ( 'NONE',  ( 1.000000000000000000, 1.850371707708593823E-16, 0.000000000000000000 ) ) ;
#4622=EDGE_LOOP ( 'NONE', ( #20541, #11941, #19367, #21894 ) ) ;
#4627=ORIENTED_EDGE ( 'NONE', *, *, #12476, .F. ) ;
#4638=CARTESIAN_POINT ( 'NONE',  ( -208.4180627997079114, 72.50595385281455663, -40.62079366388483237 ) ) ;
#4642=CARTESIAN_POINT ( 'NONE',  ( 109.9999999999999289, -40.00000000000002842, 100.0000000000000142 ) ) ;
#4643=LINE ( 'NONE', #24484, #11893 ) ;
#4646=DIRECTION ( 'NONE',  ( -0.000000000000000000, 0.000000000000000000, 1.000000000000000000 ) ) ;
#4650=CARTESIAN_POINT ( 'NONE',  ( -217.3069758534620632, 60.48634897156497203, -12.43751791598376499 ) ) ;
#4667=VERTEX_POINT ( 'NONE', #5717 ) ;
#4670=CARTESIAN_POINT ( 'NONE',  ( 92.04920872066333004, 230.5961997032264037, 17.50980340463666707 ) ) ;
#4671=EDGE_CURVE ( 'NONE', #19265, #27055, #7739, .T. ) ;
#4673=DIRECTION ( 'NONE',  ( -1.000000000000000000, 3.700743415417191886E-15, 0.000000000000000000 ) ) ;
#4677=DIRECTION ( 'NONE',  ( -4.625929269271484928E-16, 1.000000000000000000, 0.000000000000000000 ) ) ;
#4678=DIRECTION ( 'NONE',  ( -0.000000000000000000, -0.000000000000000000, 1.000000000000000000 ) ) ;
#4679=FACE_OUTER_BOUND ( 'NONE', #23256, .T. ) ;
#4683=CARTESIAN_POINT ( 'NONE',  ( -221.3650667873343139, -91.18033988749901653, 0.000000000000000000 ) ) ;
#4684=ORIENTED_EDGE ( 'NONE', *, *, #7416, .T. ) ;
#4685=CARTESIAN_POINT ( 'NONE',  ( -160.0000000000000284, 118.4170923319166633, 21.37420696376539198 ) ) ;
#4687=DIRECTION ( 'NONE',  ( 0.000000000000000000, -1.000000000000000000, 0.000000000000000000 ) ) ;
#4688=CARTESIAN_POINT ( 'NONE',  ( -68.57415822541635464, 29.64876300893806516, 95.00000000000000000 ) ) ;
#4693=CARTESIAN_POINT ( 'NONE',  ( 109.8801565119820935, 257.7417414023324795, -41.08725989922736233 ) ) ;
#4694=EDGE_LOOP ( 'NONE', ( #27857, #21716, #27142, #10641, #26323 ) ) ;
#4695=DIRECTION ( 'NONE',  ( 1.000000000000000000, 0.000000000000000000, 0.000000000000000000 ) ) ;
#4698=ORIENTED_EDGE ( 'NONE', *, *, #10927, .T. ) ;
#4703=ORIENTED_EDGE ( 'NONE', *, *, #3904, .T. ) ;
#4704=LINE ( 'NONE', #2406, #13661 ) ;
#4707=EDGE_CURVE ( 'NONE', #15896, #23283, #21458, .T. ) ;
#4712=CARTESIAN_POINT ( 'NONE',  ( -213.4585383333369180, 57.78353604556346568, 35.98283585096940129 ) ) ;
#4715=AXIS2_PLACEMENT_3D ( 'NONE', #6393, #6677, #17590 ) ;
#4717=FACE_OUTER_BOUND ( 'NONE', #28226, .T. ) ;
#4718=AXIS2_PLACEMENT_3D ( 'NONE', #4683, #6991, #20493 ) ;
#4722=CARTESIAN_POINT ( 'NONE',  ( 6.333667032819452203, 140.1905188151071968, 13.00000000068521011 ) ) ;
#4728=ORIENTED_EDGE ( 'NONE', *, *, #1442, .T. ) ;
#4729=CARTESIAN_POINT ( 'NONE',  ( 125.3433571860711453, 242.0587615242396566, 84.99999999999995737 ) ) ;
#4731=CARTESIAN_POINT ( 'NONE',  ( -207.8550219111573369, 89.23948686170545841, -26.88820707009881161 ) ) ;
#4732=ORIENTED_EDGE ( 'NONE', *, *, #1128, .T. ) ;
#4737=VECTOR ( 'NONE', #6075, 1000.000000000000000 ) ;
#4738=DIRECTION ( 'NONE',  ( 0.000000000000000000, 0.000000000000000000, 1.000000000000000000 ) ) ;
#4746=ORIENTED_EDGE ( 'NONE', *, *, #27218, .F. ) ;
#4749=ADVANCED_FACE ( 'NONE', ( #18934 ), #26051, .T. ) ;
#4752=CARTESIAN_POINT ( 'NONE',  ( -215.3329573321002783, 58.91837420257471081, -30.17944279518760098 ) ) ;
#4756=DIRECTION ( 'NONE',  ( 1.000000000000000000, -0.000000000000000000, -0.000000000000000000 ) ) ;
#4760=ORIENTED_EDGE ( 'NONE', *, *, #16462, .F. ) ;
#4761=EDGE_CURVE ( 'NONE', #27481, #21665, #17341, .T. ) ;
#4762=CARTESIAN_POINT ( 'NONE',  ( 0.000000000000000000, -18.01420295945611727, 100.0000000000000000 ) ) ;
#4770=PLANE ( 'NONE',  #11298 ) ;
#4774=DIRECTION ( 'NONE',  ( 1.000000000000000000, 0.000000000000000000, 0.000000000000000000 ) ) ;
#4775=ORIENTED_EDGE ( 'NONE', *, *, #8346, .T. ) ;
#4778=CARTESIAN_POINT ( 'NONE',  ( 5.539884921987776600, 137.3884131596613258, 15.09220095556929664 ) ) ;
#4781=DIRECTION ( 'NONE',  ( 1.000000000000000000, -0.000000000000000000, -0.000000000000000000 ) ) ;
#4783=CARTESIAN_POINT ( 'NONE',  ( 8.117852850209605009, 141.5785587194356197, -13.00000000000000000 ) ) ;
#4785=CARTESIAN_POINT ( 'NONE',  ( -207.9673235353189682, 74.11717653937235184, -42.76310609277111041 ) ) ;
#4786=CARTESIAN_POINT ( 'NONE',  ( -187.8924994060663494, 156.4650759647683742, 12.99999999999999822 ) ) ;
#4791=CYLINDRICAL_SURFACE ( 'NONE', #10273, 32.49120955644046660 ) ;
#4792=ORIENTED_EDGE ( 'NONE', *, *, #27028, .T. ) ;
#4797=EDGE_CURVE ( 'NONE', #21744, #18881, #25537, .T. ) ;
#4799=CARTESIAN_POINT ( 'NONE',  ( -215.0412094859542833, 60.20193349634170232, -13.76727271988285750 ) ) ;
#4805=CARTESIAN_POINT ( 'NONE',  ( -223.8049923706243476, 71.89136757138916778, 19.05429412414824242 ) ) ;
#4808=VERTEX_POINT ( 'NONE', #16920 ) ;
#4813=AXIS2_PLACEMENT_3D ( 'NONE', #2954, #5253, #14039 ) ;
#4814=VERTEX_POINT ( 'NONE', #17478 ) ;
#4815=ORIENTED_EDGE ( 'NONE', *, *, #12645, .T. ) ;
#4817=CARTESIAN_POINT ( 'NONE',  ( 93.75109487930637897, 231.1752187890906214, 18.33298295918253018 ) ) ;
#4820=CARTESIAN_POINT ( 'NONE',  ( -227.3657730843237061, 133.9833936510271997, -14.99191580167116911 ) ) ;
#4822=CARTESIAN_POINT ( 'NONE',  ( -125.2895325436292069, 200.2180533211636657, 12.99999999999999822 ) ) ;
#4824=FACE_OUTER_BOUND ( 'NONE', #584, .T. ) ;
#4828=CARTESIAN_POINT ( 'NONE',  ( -214.3828916364065833, 175.2783111443768576, -13.00000000000000000 ) ) ;
#4839=CARTESIAN_POINT ( 'NONE',  ( 109.9999999999998863, 259.1520133598112352, -44.26562200958714755 ) ) ;
#4841=DIRECTION ( 'NONE',  ( -1.000000000000000000, 0.000000000000000000, 0.000000000000000000 ) ) ;
#4842=AXIS2_PLACEMENT_3D ( 'NONE', #26288, #8768, #15530 ) ;
#4845=ORIENTED_EDGE ( 'NONE', *, *, #11047, .F. ) ;
#4846=EDGE_LOOP ( 'NONE', ( #27580, #494, #13805, #25717 ) ) ;
#4847=DIRECTION ( 'NONE',  ( 1.850371707708594316E-16, -1.000000000000000000, -0.000000000000000000 ) ) ;
#4855=CARTESIAN_POINT ( 'NONE',  ( -208.5306448315634213, 60.03373823553869926, 18.45924612780262208 ) ) ;
#4860=CARTESIAN_POINT ( 'NONE',  ( -223.7378885753377347, 88.77739991535318609, -14.68536764801921279 ) ) ;
#4862=B_SPLINE_CURVE_WITH_KNOTS ( 'NONE', 3,
 ( #24927, #4948, #658, #13740, #18324, #14159, #27075, #5243, #14029, #22776, #9701, #3076, #18462, #27212, #7552, #16318, #25069, #5380, #2504, #10262, #27347, #12004, #10124, #14439, #20748, #14298, #16730, #1492, #18736, #12569, #9982, #5803, #1354, #19020 ),
 .UNSPECIFIED., .F., .F.,
 ( 4, 2, 2, 2, 2, 2, 2, 2, 2, 2, 2, 2, 2, 2, 2, 2, 4 ),
 ( 0.000000000000000000, 0.003147291746946911419, 0.006294583493893822837, 0.007868229367367264235, 0.009441875240840705633, 0.01258916698778760924, 0.01573645873473451112, 0.01888375048168141473, 0.02517833397557515604, 0.02832562572252201108, 0.03147291746946885571, 0.03776750096336255885, 0.04406208445725624118, 0.04720937620420308234, 0.04878302207767650639, 0.04956984501441326352, 0.05035666795115002065 ),
 .UNSPECIFIED. ) ;
#4865=CARTESIAN_POINT ( 'NONE',  ( -143.6428522700808230, 20.24192588826928585, 83.00000000000001421 ) ) ;
#4869=DIRECTION ( 'NONE',  ( 1.000000000000000000, -0.000000000000000000, -0.000000000000000000 ) ) ;
#4876=EDGE_CURVE ( 'NONE', #24936, #223, #17337, .T. ) ;
#4877=ORIENTED_EDGE ( 'NONE', *, *, #6822, .F. ) ;
#4881=VERTEX_POINT ( 'NONE', #26096 ) ;
#4883=CARTESIAN_POINT ( 'NONE',  ( -112.7208498180836358, 133.0274648423633437, 15.80898321009636298 ) ) ;
#4892=DIRECTION ( 'NONE',  ( -0.000000000000000000, -0.000000000000000000, 1.000000000000000000 ) ) ;
#4894=CARTESIAN_POINT ( 'NONE',  ( -213.7829002709373754, 55.69945581370277665, -42.78690303009008034 ) ) ;
#4896=ADVANCED_FACE ( 'NONE', ( #6425 ), #10029, .T. ) ;
#4897=ORIENTED_EDGE ( 'NONE', *, *, #8905, .T. ) ;
#4899=CARTESIAN_POINT ( 'NONE',  ( -216.6483861793058452, 139.2130420792684902, -15.04814241299435018 ) ) ;
#4900=CARTESIAN_POINT ( 'NONE',  ( 134.9999999999998579, 220.0000000000000284, 100.0000000000000142 ) ) ;
#4905=CARTESIAN_POINT ( 'NONE',  ( -243.4193540313498545, 74.61988491602063789, 4.999999999761307379 ) ) ;
#4907=ORIENTED_EDGE ( 'NONE', *, *, #3753, .F. ) ;
#4909=CARTESIAN_POINT ( 'NONE',  ( 88.58553289623721128, 111.2425746091579413, 71.46484375014649970 ) ) ;
#4910=FACE_OUTER_BOUND ( 'NONE', #12193, .T. ) ;
#4914=CYLINDRICAL_SURFACE ( 'NONE', #12713, 5.000000000000004441 ) ;
#4916=ORIENTED_EDGE ( 'NONE', *, *, #17562, .F. ) ;
#4919=ORIENTED_EDGE ( 'NONE', *, *, #9300, .T. ) ;
#4920=CARTESIAN_POINT ( 'NONE',  ( 9.345921402568853509, 139.9999999999999716, -13.00000000000000000 ) ) ;
#4923=CARTESIAN_POINT ( 'NONE',  ( -4.329335832958885355, 134.1424492706239846, -13.93339712843492606 ) ) ;
#4926=AXIS2_PLACEMENT_3D ( 'NONE', #3480, #21146, #3614 ) ;
#4927=ADVANCED_FACE ( 'NONE', ( #12765 ), #9569, .T. ) ;
#4930=CARTESIAN_POINT ( 'NONE',  ( -63.57415822541634043, -18.01420295945611727, 100.0000000000000000 ) ) ;
#4936=ORIENTED_EDGE ( 'NONE', *, *, #10894, .F. ) ;
#4944=EDGE_CURVE ( 'NONE', #25070, #5248, #7289, .T. ) ;
#4945=FACE_OUTER_BOUND ( 'NONE', #18526, .T. ) ;
#4947=ADVANCED_FACE ( 'NONE', ( #8448 ), #25594, .F. ) ;
#4948=CARTESIAN_POINT ( 'NONE',  ( 90.99996944231388341, 240.0000000000000568, 6.657453037605657542 ) ) ;
#4949=ORIENTED_EDGE ( 'NONE', *, *, #7416, .F. ) ;
#4952=ORIENTED_EDGE ( 'NONE', *, *, #7787, .F. ) ;
#4953=AXIS2_PLACEMENT_3D ( 'NONE', #3553, #18653, #10036 ) ;
#4955=ORIENTED_EDGE ( 'NONE', *, *, #16813, .F. ) ;
#4958=CARTESIAN_POINT ( 'NONE',  ( 90.45806322831077750, 239.6644751351248317, 16.82109631826968865 ) ) ;
#4960=CARTESIAN_POINT ( 'NONE',  ( -219.9082363642617111, 137.1815813412194700, 12.98324324876687186 ) ) ;
#4961=CARTESIAN_POINT ( 'NONE',  ( 65.00000000000000000, -120.0000000000000711, 70.00000000000001421 ) ) ;
#4966=LINE ( 'NONE', #5539, #7647 ) ;
#4967=FACE_OUTER_BOUND ( 'NONE', #22589, .T. ) ;
#4971=ORIENTED_EDGE ( 'NONE', *, *, #8571, .T. ) ;
#4973=CIRCLE ( 'NONE', #19186, 5.999999999999991118 ) ;
#4975=CARTESIAN_POINT ( 'NONE',  ( 79.99999999999994316, -100.0000000000000284, 100.0000000000000142 ) ) ;
#4977=CARTESIAN_POINT ( 'NONE',  ( -221.3650667873343139, -91.18033988749901653, -14.94182580522077330 ) ) ;
#4978=ORIENTED_EDGE ( 'NONE', *, *, #16413, .T. ) ;
#4985=AXIS2_PLACEMENT_3D ( 'NONE', #21400, #139, #10630 ) ;
#4989=CYLINDRICAL_SURFACE ( 'NONE', #7230, 53.86582179324592090 ) ;
#4990=DIRECTION ( 'NONE',  ( 0.000000000000000000, 0.000000000000000000, -1.000000000000000000 ) ) ;
#4992=CIRCLE ( 'NONE', #28371, 16.07743405327025243 ) ;
#4993=CIRCLE ( 'NONE', #26965, 1.000000000000000888 ) ;
#4994=CARTESIAN_POINT ( 'NONE',  ( -43.02437977270767533, 129.7200458115292747, -16.81627168235289105 ) ) ;
#4995=EDGE_CURVE ( 'NONE', #26118, #11930, #16200, .T. ) ;
#4999=CARTESIAN_POINT ( 'NONE',  ( -215.6254804987316334, 60.26473849368087343, 13.41209097274074047 ) ) ;
#5001=DIRECTION ( 'NONE',  ( 0.000000000000000000, 0.000000000000000000, 1.000000000000000000 ) ) ;
#5002=CARTESIAN_POINT ( 'NONE',  ( 79.99999999999991473, 80.00000000000001421, -100.0000000000000142 ) ) ;
#5003=CARTESIAN_POINT ( 'NONE',  ( -223.0561610845317375, 88.57719356741800709, -14.95839461110579016 ) ) ;
#5004=EDGE_CURVE ( 'NONE', #3825, #10017, #11465, .T. ) ;
#5005=LINE ( 'NONE', #22399, #11979 ) ;
#5007=CARTESIAN_POINT ( 'NONE',  ( 82.68942924499303615, 110.0997128786253683, 70.07812500014873081 ) ) ;
#5009=CARTESIAN_POINT ( 'NONE',  ( -17.77354996712479007, 128.7458775741096133, 17.18687607546115004 ) ) ;
#5011=VECTOR ( 'NONE', #5846, 1000.000000000000000 ) ;
#5014=EDGE_LOOP ( 'NONE', ( #27583, #27170, #6085, #12182 ) ) ;
#5016=CARTESIAN_POINT ( 'NONE',  ( -215.9971974014444811, 86.39790881275628465, -21.03121872006250825 ) ) ;
#5019=ORIENTED_EDGE ( 'NONE', *, *, #12839, .T. ) ;
#5021=CIRCLE ( 'NONE', #27487, 1.999999999999998224 ) ;
#5029=AXIS2_PLACEMENT_3D ( 'NONE', #3004, #26708, #22408 ) ;
#5035=EDGE_CURVE ( 'NONE', #20039, #14569, #4973, .T. ) ;
#5039=CARTESIAN_POINT ( 'NONE',  ( -124.9781469243919076, 222.2250949724356985, -5.000000000000004441 ) ) ;
#5040=CARTESIAN_POINT ( 'NONE',  ( -207.8278798888169945, 75.36218601466582356, -41.22349376586717540 ) ) ;
#5046=LINE ( 'NONE', #614, #6408 ) ;
#5048=LINE ( 'NONE', #19855, #10803 ) ;
#5049=ORIENTED_EDGE ( 'NONE', *, *, #6093, .F. ) ;
#5052=VECTOR ( 'NONE', #19381, 1000.000000000000000 ) ;
#5055=CARTESIAN_POINT ( 'NONE',  ( -175.0000000000000000, -120.0000000000001705, 70.00000000000001421 ) ) ;
#5056=ORIENTED_EDGE ( 'NONE', *, *, #14671, .F. ) ;
#5059=DIRECTION ( 'NONE',  ( -1.000000000000000000, 0.000000000000000000, 0.000000000000000000 ) ) ;
#5061=FACE_OUTER_BOUND ( 'NONE', #4560, .T. ) ;
#5062=CARTESIAN_POINT ( 'NONE',  ( -216.6483861793289805, 139.2130420793173471, 15.04814241300593913 ) ) ;
#5063=VERTEX_POINT ( 'NONE', #11316 ) ;
#5067=ADVANCED_FACE ( 'NONE', ( #13616 ), #24236, .T. ) ;
#5069=EDGE_CURVE ( 'NONE', #10866, #19795, #27095, .T. ) ;
#5072=CARTESIAN_POINT ( 'NONE',  ( 6.334507319946773407, 140.1911725318066715, -13.00000000064436634 ) ) ;
#5080=DIRECTION ( 'NONE',  ( -1.000000000000000000, 0.000000000000000000, 0.000000000000000000 ) ) ;
#5082=CARTESIAN_POINT ( 'NONE',  ( -200.0000000000000284, -62.36067977499792647, 25.00000000000000000 ) ) ;
#5083=ORIENTED_EDGE ( 'NONE', *, *, #22187, .F. ) ;
#5084=DIRECTION ( 'NONE',  ( 1.000000000000000000, 0.000000000000000000, -0.000000000000000000 ) ) ;
#5086=CARTESIAN_POINT ( 'NONE',  ( 79.99999999999992895, 240.0000000000000284, 5.000000000000002665 ) ) ;
#5091=DIRECTION ( 'NONE',  ( -1.000000000000000000, 0.000000000000000000, 0.000000000000000000 ) ) ;
#5093=CIRCLE ( 'NONE', #20678, 6.025000000000002132 ) ;
#5094=CARTESIAN_POINT ( 'NONE',  ( -62.69330818947670281, 133.3645688629142967, 15.73244652714148373 ) ) ;
#5098=EDGE_CURVE ( 'NONE', #2906, #24273, #20206, .T. ) ;
#5099=VERTEX_POINT ( 'NONE', #7426 ) ;
#5102=ADVANCED_FACE ( 'NONE', ( #15627 ), #7284, .T. ) ;
#5108=DIRECTION ( 'NONE',  ( 1.000000000000000000, 0.000000000000000000, 0.000000000000000000 ) ) ;
#5114=DIRECTION ( 'NONE',  ( -0.000000000000000000, -0.000000000000000000, 1.000000000000000000 ) ) ;
#5117=DIRECTION ( 'NONE',  ( -0.000000000000000000, -0.000000000000000000, 1.000000000000000000 ) ) ;
#5118=LINE ( 'NONE', #11166, #6125 ) ;
#5121=CYLINDRICAL_SURFACE ( 'NONE', #22970, 30.00000000000000000 ) ;
#5126=ORIENTED_EDGE ( 'NONE', *, *, #11746, .T. ) ;
#5128=EDGE_CURVE ( 'NONE', #1940, #12493, #21033, .T. ) ;
#5131=CARTESIAN_POINT ( 'NONE',  ( -141.6428522700808230, 69.54464929955099706, 83.00000000000001421 ) ) ;
#5137=ORIENTED_EDGE ( 'NONE', *, *, #24717, .T. ) ;
#5138=CARTESIAN_POINT ( 'NONE',  ( -138.8850951481510378, 128.5925778606047061, 15.90076932754394612 ) ) ;
#5140=CARTESIAN_POINT ( 'NONE',  ( -110.3221550338875687, 68.51688903468615877, 83.00000000000001421 ) ) ;
#5143=CARTESIAN_POINT ( 'NONE',  ( -107.9388568470210856, 135.2304614929108482, -15.33442335600818396 ) ) ;
#5147=CARTESIAN_POINT ( 'NONE',  ( -207.7463451706791773, 75.42136631982602069, 41.72512927420302020 ) ) ;
#5151=CARTESIAN_POINT ( 'NONE',  ( 79.99999999999995737, 109.8066173636171499, -73.92694226569399518 ) ) ;
#5155=CARTESIAN_POINT ( 'NONE',  ( 109.9999999999999147, 137.0808454111986237, 89.99999999939370809 ) ) ;
#5163=EDGE_LOOP ( 'NONE', ( #20366, #23723, #15792 ) ) ;
#5165=CARTESIAN_POINT ( 'NONE',  ( -220.6963704969327011, 86.29915981945389092, -18.37871326271141115 ) ) ;
#5167=LINE ( 'NONE', #19436, #20295 ) ;
#5168=ORIENTED_EDGE ( 'NONE', *, *, #7787, .T. ) ;
#5172=CARTESIAN_POINT ( 'NONE',  ( -122.5470052484187704, 131.3754805985278438, 16.25370679815316066 ) ) ;
#5180=DIRECTION ( 'NONE',  ( 0.000000000000000000, 0.000000000000000000, -1.000000000000000000 ) ) ;
#5186=CARTESIAN_POINT ( 'NONE',  ( -209.7310389751728508, 59.98715598645322444, -17.47553936829965338 ) ) ;
#5194=CARTESIAN_POINT ( 'NONE',  ( -235.5733620266476578, 80.43390826602548316, 15.03591609561660469 ) ) ;
#5200=ORIENTED_EDGE ( 'NONE', *, *, #22259, .T. ) ;
#5201=EDGE_CURVE ( 'NONE', #10815, #14295, #10283, .T. ) ;
#5205=DIRECTION ( 'NONE',  ( 1.000000000000000000, 0.000000000000000000, 0.000000000000000000 ) ) ;
#5213=VECTOR ( 'NONE', #4211, 1000.000000000000000 ) ;
#5217=CARTESIAN_POINT ( 'NONE',  ( -25.41071799330663694, 129.2224460950298237, -15.66088409790421920 ) ) ;
#5218=VECTOR ( 'NONE', #7948, 1000.000000000000000 ) ;
#5222=ORIENTED_EDGE ( 'NONE', *, *, #6943, .F. ) ;
#5224=CYLINDRICAL_SURFACE ( 'NONE', #21940, 5.999999999999991118 ) ;
#5225=DIRECTION ( 'NONE',  ( 0.000000000000000000, 0.000000000000000000, -1.000000000000000000 ) ) ;
#5227=FACE_OUTER_BOUND ( 'NONE', #23456, .T. ) ;
#5229=CARTESIAN_POINT ( 'NONE',  ( -231.1953787138146765, 65.04295872140690449, 6.836033801457080727 ) ) ;
#5231=DIRECTION ( 'NONE',  ( 1.000000000000000000, 0.000000000000000000, 0.000000000000000000 ) ) ;
#5232=CARTESIAN_POINT ( 'NONE',  ( -220.3653290071072206, 61.04242272473436515, -10.83006322850141778 ) ) ;
#5235=LINE ( 'NONE', #653, #2818 ) ;
#5236=CARTESIAN_POINT ( 'NONE',  ( -146.6428522700808230, 22.24192588826928585, 80.00000000000001421 ) ) ;
#5238=EDGE_LOOP ( 'NONE', ( #1910, #26945, #17264 ) ) ;
#5243=CARTESIAN_POINT ( 'NONE',  ( 97.02590988242761227, 241.2701841432802041, 10.66915916737285031 ) ) ;
#5245=VECTOR ( 'NONE', #22438, 1000.000000000000000 ) ;
#5246=ORIENTED_EDGE ( 'NONE', *, *, #20910, .T. ) ;
#5248=VERTEX_POINT ( 'NONE', #27232 ) ;
#5249=ORIENTED_EDGE ( 'NONE', *, *, #84, .T. ) ;
#5250=ORIENTED_EDGE ( 'NONE', *, *, #17544, .F. ) ;
#5251=CARTESIAN_POINT ( 'NONE',  ( 107.7175597583454021, 250.4128021203281946, 33.27520275799354010 ) ) ;
#5252=VECTOR ( 'NONE', #1001, 1000.000000000000000 ) ;
#5253=DIRECTION ( 'NONE',  ( 0.000000000000000000, 0.000000000000000000, 1.000000000000000000 ) ) ;
#5254=CARTESIAN_POINT ( 'NONE',  ( 79.99999999999994316, -70.00000000000002842, 100.0000000000000142 ) ) ;
#5256=CARTESIAN_POINT ( 'NONE',  ( 101.7779539750033280, 119.2876405404464890, -82.50000000032424907 ) ) ;
#5259=DIRECTION ( 'NONE',  ( 0.8018642810807398158, 0.5975062131282554700, -0.000000000000000000 ) ) ;
#5264=CARTESIAN_POINT ( 'NONE',  ( 115.6411010564591777, 208.5333949359988139, -99.00000000000001421 ) ) ;
#5268=EDGE_CURVE ( 'NONE', #5960, #11012, #9607, .T. ) ;
#5271=LINE ( 'NONE', #14056, #10621 ) ;
#5277=VECTOR ( 'NONE', #21179, 1000.000000000000000 ) ;
#5278=CIRCLE ( 'NONE', #3889, 4.355764593064429313 ) ;
#5284=CARTESIAN_POINT ( 'NONE',  ( -75.07674457730871609, 136.1111122117180798, 13.54517443609203653 ) ) ;
#5286=CARTESIAN_POINT ( 'NONE',  ( 109.9999999999999432, 2.035408878479452500E-14, 100.0000000000000142 ) ) ;
#5287=CARTESIAN_POINT ( 'NONE',  ( -42.65532241761712839, 131.0044336801081784, -16.34779397420837910 ) ) ;
#5288=CARTESIAN_POINT ( 'NONE',  ( -18.10916961908506551, 129.9686900844010893, 15.33252739753482885 ) ) ;
#5289=CARTESIAN_POINT ( 'NONE',  ( -207.5064340660269693, 75.59749780642115979, 45.29313139209890693 ) ) ;
#5290=CARTESIAN_POINT ( 'NONE',  ( 79.99999999999994316, -100.0000000000000284, 25.00000000000000711 ) ) ;
#5291=CARTESIAN_POINT ( 'NONE',  ( -59.48697296830715686, 2.336311854928213219E-15, 100.0000000000000000 ) ) ;
#5292=DIRECTION ( 'NONE',  ( 1.000000000000000000, 0.000000000000000000, 0.000000000000000000 ) ) ;
#5294=CARTESIAN_POINT ( 'NONE',  ( -211.7690755206428719, 88.48850965457344842, -21.98930932911726899 ) ) ;
#5299=EDGE_CURVE ( 'NONE', #23283, #9810, #12731, .T. ) ;
#5300=EDGE_CURVE ( 'NONE', #7257, #366, #8193, .T. ) ;
#5302=CARTESIAN_POINT ( 'NONE',  ( -192.4056874188291602, 101.4351547665440023, 32.80394979098671371 ) ) ;
#5303=DIRECTION ( 'NONE',  ( 0.000000000000000000, 0.000000000000000000, 1.000000000000000000 ) ) ;
#5310=ADVANCED_FACE ( 'NONE', ( #21764 ), #10969, .F. ) ;
#5318=CARTESIAN_POINT ( 'NONE',  ( -17.24491960465745777, -18.01420295945611727, 80.00000000000001421 ) ) ;
#5319=DIRECTION ( 'NONE',  ( -0.000000000000000000, -0.000000000000000000, -1.000000000000000000 ) ) ;
#5322=CARTESIAN_POINT ( 'NONE',  ( 93.83233610022676885, 231.2056637020306198, -18.37429547533238861 ) ) ;
#5327=CARTESIAN_POINT ( 'NONE',  ( -221.9864287755668784, 60.98533040124252835, -21.67821222923991442 ) ) ;
#5328=CARTESIAN_POINT ( 'NONE',  ( 109.9999999999999005, 230.0000000000000284, -5.000000000000004441 ) ) ;
#5332=ORIENTED_EDGE ( 'NONE', *, *, #12122, .F. ) ;
#5335=CARTESIAN_POINT ( 'NONE',  ( -239.6893155506737401, 70.91029463950323475, 5.253362301622646946 ) ) ;
#5342=EDGE_CURVE ( 'NONE', #15188, #23617, #9124, .T. ) ;
#5343=CARTESIAN_POINT ( 'NONE',  ( 105.2480867105129505, 123.6573351778161793, 100.0000000000216573 ) ) ;
#5346=VERTEX_POINT ( 'NONE', #8409 ) ;
#5356=CARTESIAN_POINT ( 'NONE',  ( 4.595825946142663376, 138.9899071332870335, -14.95390936462971254 ) ) ;
#5357=DIRECTION ( 'NONE',  ( 0.000000000000000000, 0.000000000000000000, 1.000000000000000000 ) ) ;
#5364=EDGE_CURVE ( 'NONE', #12131, #4224, #18322, .T. ) ;
#5367=ORIENTED_EDGE ( 'NONE', *, *, #7288, .F. ) ;
#5368=DIRECTION ( 'NONE',  ( -1.000000000000000000, -2.602085213965211135E-16, 0.000000000000000000 ) ) ;
#5370=DIRECTION ( 'NONE',  ( 0.000000000000000000, 0.000000000000000000, -1.000000000000000000 ) ) ;
#5371=PLANE ( 'NONE',  #10113 ) ;
#5374=DIRECTION ( 'NONE',  ( 0.000000000000000000, 0.000000000000000000, 1.000000000000000000 ) ) ;
#5375=CARTESIAN_POINT ( 'NONE',  ( -68.57415822541635464, 24.64876300893806160, 95.00000000000000000 ) ) ;
#5379=CARTESIAN_POINT ( 'NONE',  ( -77.65366760726760731, 134.6132604961730124, 15.48745542953684939 ) ) ;
#5380=CARTESIAN_POINT ( 'NONE',  ( 106.1557582624860601, 248.1951032683517724, 24.28480840886491876 ) ) ;
#5384=VERTEX_POINT ( 'NONE', #26062 ) ;
#5391=CIRCLE ( 'NONE', #13678, 30.00000000000000000 ) ;
#5393=VECTOR ( 'NONE', #15042, 1000.000000000000000 ) ;
#5395=CARTESIAN_POINT ( 'NONE',  ( 93.07270601803662657, 112.9533406971499971, -74.06249999970600584 ) ) ;
#5397=FACE_OUTER_BOUND ( 'NONE', #2126, .T. ) ;
#5398=EDGE_CURVE ( 'NONE', #15531, #27002, #23493, .T. ) ;
#5399=DIRECTION ( 'NONE',  ( 0.6782242722910298838, 0.7348549764921669114, 0.000000000000000000 ) ) ;
#5402=DIRECTION ( 'NONE',  ( 0.000000000000000000, 0.000000000000000000, 1.000000000000000000 ) ) ;
#5403=ORIENTED_EDGE ( 'NONE', *, *, #25753, .F. ) ;
#5410=EDGE_LOOP ( 'NONE', ( #6509, #1412, #22952, #16546 ) ) ;
#5417=CARTESIAN_POINT ( 'NONE',  ( -42.53273978471831640, 130.9733465240572627, 14.93735646117640847 ) ) ;
#5421=ADVANCED_FACE ( 'NONE', ( #782 ), #26474, .T. ) ;
#5422=AXIS2_PLACEMENT_3D ( 'NONE', #5131, #27108, #4841 ) ;
#5425=EDGE_CURVE ( 'NONE', #19092, #11112, #24198, .T. ) ;
#5427=CARTESIAN_POINT ( 'NONE',  ( -97.84640529597095338, 136.0962391708293353, -13.54842801288088161 ) ) ;
#5429=CARTESIAN_POINT ( 'NONE',  ( 65.00000000000000000, -150.0000000000000568, 64.00000000000002842 ) ) ;
#5431=CARTESIAN_POINT ( 'NONE',  ( -217.2892621185082760, 109.4029876883478352, 12.99999999999999822 ) ) ;
#5434=CYLINDRICAL_SURFACE ( 'NONE', #1081, 24.07986109634097005 ) ;
#5438=CARTESIAN_POINT ( 'NONE',  ( -189.5231184314567940, 157.6231267382816554, -15.00000000000000000 ) ) ;
#5445=ORIENTED_EDGE ( 'NONE', *, *, #142, .T. ) ;
#5447=AXIS2_PLACEMENT_3D ( 'NONE', #604, #20413, #9367 ) ;
#5456=CARTESIAN_POINT ( 'NONE',  ( 96.79691392614289214, 232.6553747178996332, -20.12435212500413684 ) ) ;
#5458=AXIS2_PLACEMENT_3D ( 'NONE', #19431, #17271, #4193 ) ;
#5459=VECTOR ( 'NONE', #15975, 1000.000000000000000 ) ;
#5462=CARTESIAN_POINT ( 'NONE',  ( -215.1670473708328473, 71.77859382844975755, -26.43926314730827443 ) ) ;
#5463=AXIS2_PLACEMENT_3D ( 'NONE', #21837, #10631, #2001 ) ;
#5464=EDGE_CURVE ( 'NONE', #16435, #4097, #2236, .T. ) ;
#5469=ORIENTED_EDGE ( 'NONE', *, *, #8870, .F. ) ;
#5471=CIRCLE ( 'NONE', #9610, 6.025000000000002132 ) ;
#5472=CARTESIAN_POINT ( 'NONE',  ( -230.6117145417363190, 64.61843588005640981, 16.59905221104221695 ) ) ;
#5478=CARTESIAN_POINT ( 'NONE',  ( 109.9999999999999147, 137.0808454111986237, 89.99999999939370809 ) ) ;
#5479=VECTOR ( 'NONE', #15850, 1000.000000000000000 ) ;
#5481=VERTEX_POINT ( 'NONE', #19884 ) ;
#5482=AXIS2_PLACEMENT_3D ( 'NONE', #18904, #12316, #21058 ) ;
#5485=CIRCLE ( 'NONE', #16531, 10.00000000000000888 ) ;
#5486=EDGE_CURVE ( 'NONE', #7588, #27001, #20169, .T. ) ;
#5488=CARTESIAN_POINT ( 'NONE',  ( -210.7172313291012529, 103.7585653882801182, 15.00000000000000000 ) ) ;
#5491=ORIENTED_EDGE ( 'NONE', *, *, #10051, .F. ) ;
#5493=AXIS2_PLACEMENT_3D ( 'NONE', #15225, #26399, #15651 ) ;
#5497=CARTESIAN_POINT ( 'NONE',  ( -175.0000000000000000, -120.0000000000001847, -64.00000000000000000 ) ) ;
#5498=EDGE_CURVE ( 'NONE', #15391, #15494, #4643, .T. ) ;
#5500=CARTESIAN_POINT ( 'NONE',  ( -279.3160071107327553, -91.18033988749907337, 0.000000000000000000 ) ) ;
#5501=ORIENTED_EDGE ( 'NONE', *, *, #27229, .T. ) ;
#5506=DIRECTION ( 'NONE',  ( 1.000000000000000000, -0.000000000000000000, -0.000000000000000000 ) ) ;
#5509=AXIS2_PLACEMENT_3D ( 'NONE', #14430, #9692, #9832 ) ;
#5512=CARTESIAN_POINT ( 'NONE',  ( -175.0000000000000000, -120.0250000000001762, 70.00000000000001421 ) ) ;
#5516=( LENGTH_UNIT ( ) NAMED_UNIT ( * ) SI_UNIT ( .MILLI., .METRE. ) );
#5517=DIRECTION ( 'NONE',  ( -0.000000000000000000, -0.000000000000000000, 1.000000000000000000 ) ) ;
#5520=CARTESIAN_POINT ( 'NONE',  ( -180.0000000000000284, -2.775557561562891982E-14, 70.00000000000001421 ) ) ;
#5524=ORIENTED_EDGE ( 'NONE', *, *, #8976, .F. ) ;
#5528=AXIS2_PLACEMENT_3D ( 'NONE', #17015, #3801, #7834 ) ;
#5529=ADVANCED_FACE ( 'NONE', ( #13869 ), #12239, .F. ) ;
#5530=EDGE_LOOP ( 'NONE', ( #11034, #7616, #27944, #16929 ) ) ;
#5532=CARTESIAN_POINT ( 'NONE',  ( 109.9999999999999005, 260.0000000000000000, 45.00000000000000000 ) ) ;
#5533=AXIS2_PLACEMENT_3D ( 'NONE', #4685, #393, #253 ) ;
#5537=CARTESIAN_POINT ( 'NONE',  ( -17.24491960465746132, -23.01420295945612082, 95.00000000000000000 ) ) ;
#5539=CARTESIAN_POINT ( 'NONE',  ( 157.4999999999998579, 220.0000000000000284, -105.0000000000000284 ) ) ;
#5545=CARTESIAN_POINT ( 'NONE',  ( -6.707964895605361022, 133.1658889964437549, 15.75304700660547574 ) ) ;
#5546=CIRCLE ( 'NONE', #18848, 2.000000000000003109 ) ;
#5548=CARTESIAN_POINT ( 'NONE',  ( 29.38151960293523501, 82.99431933797082195, 99.87622392724593112 ) ) ;
#5551=VERTEX_POINT ( 'NONE', #12797 ) ;
#5557=ADVANCED_FACE ( 'NONE', ( #10491 ), #18966, .T. ) ;
#5562=ORIENTED_EDGE ( 'NONE', *, *, #1145, .F. ) ;
#5570=CARTESIAN_POINT ( 'NONE',  ( -194.4086842179900714, 63.14614340836796913, 41.97977085781615614 ) ) ;
#5573=ADVANCED_FACE ( 'NONE', ( #21259 ), #27710, .T. ) ;
#5574=DIRECTION ( 'NONE',  ( 0.000000000000000000, 0.000000000000000000, -1.000000000000000000 ) ) ;
#5577=DIRECTION ( 'NONE',  ( 0.000000000000000000, 0.000000000000000000, 1.000000000000000000 ) ) ;
#5578=FACE_OUTER_BOUND ( 'NONE', #11855, .T. ) ;
#5579=ORIENTED_EDGE ( 'NONE', *, *, #3883, .T. ) ;
#5582=DIRECTION ( 'NONE',  ( 1.000000000000000000, 0.000000000000000000, 0.000000000000000000 ) ) ;
#5584=EDGE_LOOP ( 'NONE', ( #2684, #22836 ) ) ;
#5586=AXIS2_PLACEMENT_3D ( 'NONE', #22763, #27198, #9407 ) ;
#5598=DIRECTION ( 'NONE',  ( 0.000000000000000000, 0.000000000000000000, 1.000000000000000000 ) ) ;
#5599=CARTESIAN_POINT ( 'NONE',  ( 79.99999999999992895, 230.0000000000000284, 45.00000000000000000 ) ) ;
#5600=CARTESIAN_POINT ( 'NONE',  ( 109.2201764734642495, 251.9989660840318209, -38.05726333473669598 ) ) ;
#5605=AXIS2_PLACEMENT_3D ( 'NONE', #19916, #13757, #11161 ) ;
#5607=DIRECTION ( 'NONE',  ( 1.000000000000000000, 0.000000000000000000, 0.000000000000000000 ) ) ;
#5608=CARTESIAN_POINT ( 'NONE',  ( -214.2335385402416534, 55.09354448559546569, -44.71599978583095236 ) ) ;
#5609=VECTOR ( 'NONE', #11796, 1000.000000000000000 ) ;
#5613=ORIENTED_EDGE ( 'NONE', *, *, #10894, .T. ) ;
#5616=DIRECTION ( 'NONE',  ( 0.000000000000000000, 0.000000000000000000, 1.000000000000000000 ) ) ;
#5625=EDGE_CURVE ( 'NONE', #20966, #24930, #6366, .T. ) ;
#5631=EDGE_CURVE ( 'NONE', #16686, #20219, #12358, .T. ) ;
#5632=CARTESIAN_POINT ( 'NONE',  ( 98.66162091205576701, 233.9456586972327727, 21.50625937152093670 ) ) ;
#5641=CARTESIAN_POINT ( 'NONE',  ( 22.58950924271104910, 154.2349915562422780, 15.00000000000000000 ) ) ;
#5643=VECTOR ( 'NONE', #12121, 1000.000000000000000 ) ;
#5645=CARTESIAN_POINT ( 'NONE',  ( -178.5907483116646119, 110.5436109027794203, -30.33689931536702389 ) ) ;
#5648=DIRECTION ( 'NONE',  ( 1.000000000000000000, 0.000000000000000000, 0.000000000000000000 ) ) ;
#5651=AXIS2_PLACEMENT_3D ( 'NONE', #986, #3270, #10317 ) ;
#5654=LINE ( 'NONE', #25471, #16046 ) ;
#5656=ADVANCED_FACE ( 'NONE', ( #27851, #14012 ), #8188, .F. ) ;
#5658=DIRECTION ( 'NONE',  ( 0.000000000000000000, 0.000000000000000000, -1.000000000000000000 ) ) ;
#5661=CARTESIAN_POINT ( 'NONE',  ( -107.3221550338875687, 69.54464929955099706, 83.00000000000001421 ) ) ;
#5673=EDGE_CURVE ( 'NONE', #1493, #11930, #4992, .T. ) ;
#5677=CARTESIAN_POINT ( 'NONE',  ( 109.2808348379980856, 254.3902513976626949, 38.18180188068609482 ) ) ;
#5678=LINE ( 'NONE', #18886, #14010 ) ;
#5679=DIRECTION ( 'NONE',  ( 0.000000000000000000, 0.000000000000000000, 1.000000000000000000 ) ) ;
#5680=ADVANCED_FACE ( 'NONE', ( #13225 ), #26135, .F. ) ;
#5681=CARTESIAN_POINT ( 'NONE',  ( 116.2340178909016970, 207.5736003696172816, -99.27034901580077531 ) ) ;
#5684=EDGE_CURVE ( 'NONE', #24273, #19795, #27040, .T. ) ;
#5690=AXIS2_PLACEMENT_3D ( 'NONE', #13715, #7238, #634 ) ;
#5692=CARTESIAN_POINT ( 'NONE',  ( 107.1321927721269134, 249.6641751418899844, -26.92697050482404819 ) ) ;
#5693=CARTESIAN_POINT ( 'NONE',  ( 22.72047449844828293, 87.17468966359002991, 99.13026680618094133 ) ) ;
#5695=DIRECTION ( 'NONE',  ( 0.000000000000000000, 0.000000000000000000, -1.000000000000000000 ) ) ;
#5698=ORIENTED_EDGE ( 'NONE', *, *, #6331, .F. ) ;
#5700=ORIENTED_EDGE ( 'NONE', *, *, #2534, .T. ) ;
#5703=ORIENTED_EDGE ( 'NONE', *, *, #11863, .F. ) ;
#5704=CARTESIAN_POINT ( 'NONE',  ( -92.89132778029807014, 136.4114671995147603, 15.16824819155097259 ) ) ;
#5710=CARTESIAN_POINT ( 'NONE',  ( 39.99999999999995026, -19.99999999999983302, 80.00000000000001421 ) ) ;
#5711=CARTESIAN_POINT ( 'NONE',  ( 6.071532165918828775E-15, -70.00000000000002842, 100.0000000000000142 ) ) ;
#5713=DIRECTION ( 'NONE',  ( 1.000000000000000000, 0.000000000000000000, 0.000000000000000000 ) ) ;
#5717=CARTESIAN_POINT ( 'NONE',  ( -12.24491960465745599, 75.97823757117562593, 80.00000000000001421 ) ) ;
#5722=CARTESIAN_POINT ( 'NONE',  ( 85.37729192593057803, 80.27798593821322015, -100.0000000000000142 ) ) ;
#5726=CARTESIAN_POINT ( 'NONE',  ( -76.25760768171835480, 221.6666220619077876, 12.99999999999999822 ) ) ;
#5727=ORIENTED_EDGE ( 'NONE', *, *, #12293, .F. ) ;
#5732=ORIENTED_EDGE ( 'NONE', *, *, #18471, .T. ) ;
#5735=EDGE_CURVE ( 'NONE', #14118, #8411, #282, .T. ) ;
#5736=FACE_OUTER_BOUND ( 'NONE', #17102, .T. ) ;
#5743=AXIS2_PLACEMENT_3D ( 'NONE', #10640, #25857, #6316 ) ;
#5746=CARTESIAN_POINT ( 'NONE',  ( -207.5064340660269693, 75.59749780642115979, -45.29313139209890693 ) ) ;
#5750=EDGE_CURVE ( 'NONE', #2012, #24201, #25664, .T. ) ;
#5752=DIRECTION ( 'NONE',  ( 0.000000000000000000, 0.000000000000000000, 1.000000000000000000 ) ) ;
#5755=CARTESIAN_POINT ( 'NONE',  ( -189.5697394631524730, 103.4865528990713841, 32.83955206258175252 ) ) ;
#5758=AXIS2_PLACEMENT_3D ( 'NONE', #27188, #4781, #13566 ) ;
#5760=AXIS2_PLACEMENT_3D ( 'NONE', #27501, #7978, #21042 ) ;
#5762=VERTEX_POINT ( 'NONE', #8906 ) ;
#5763=CARTESIAN_POINT ( 'NONE',  ( 98.15430812625453427, 116.0637945822804795, 100.0000000000432863 ) ) ;
#5764=DIRECTION ( 'NONE',  ( 1.000000000000000000, 0.000000000000000000, 0.000000000000000000 ) ) ;
#5770=CYLINDRICAL_SURFACE ( 'NONE', #18769, 43.76444293738735070 ) ;
#5772=CARTESIAN_POINT ( 'NONE',  ( 114.5273445118512967, 107.2595481030940476, 100.0000000000000142 ) ) ;
#5773=EDGE_LOOP ( 'NONE', ( #3382, #11862, #24319, #7244 ) ) ;
#5788=DIRECTION ( 'NONE',  ( -1.000000000000000000, 0.000000000000000000, 0.000000000000000000 ) ) ;
#5795=CARTESIAN_POINT ( 'NONE',  ( 79.99999999999992895, 230.0000000000000284, 45.00000000000000000 ) ) ;
#5800=CARTESIAN_POINT ( 'NONE',  ( -76.25760768171835480, 219.6666220619077876, 12.99999999999999822 ) ) ;
#5803=CARTESIAN_POINT ( 'NONE',  ( 109.9986890988327559, 259.7355369120359683, 44.54193649829915813 ) ) ;
#5805=AXIS2_PLACEMENT_3D ( 'NONE', #25205, #12433, #16734 ) ;
#5811=LINE ( 'NONE', #4072, #7501 ) ;
#5813=DIRECTION ( 'NONE',  ( -1.000000000000000000, -1.321694076934710155E-16, 0.000000000000000000 ) ) ;
#5814=CARTESIAN_POINT ( 'NONE',  ( -146.6428522700808230, 22.24192588826928585, 83.00000000000001421 ) ) ;
#5815=CARTESIAN_POINT ( 'NONE',  ( 117.2367070128591422, 206.1781180960884683, -99.61792820886472555 ) ) ;
#5817=CARTESIAN_POINT ( 'NONE',  ( -223.4642351922133230, 61.48957812539607914, -20.50364820523719089 ) ) ;
#5823=ORIENTED_EDGE ( 'NONE', *, *, #8346, .F. ) ;
#5824=DIRECTION ( 'NONE',  ( -1.000000000000000000, 0.000000000000000000, 0.000000000000000000 ) ) ;
#5829=CARTESIAN_POINT ( 'NONE',  ( 30.93948709196389402, 81.58894172419465463, 100.0000000000000426 ) ) ;
#5833=VERTEX_POINT ( 'NONE', #13949 ) ;
#5839=ORIENTED_EDGE ( 'NONE', *, *, #19351, .T. ) ;
#5843=ORIENTED_EDGE ( 'NONE', *, *, #5625, .T. ) ;
#5844=CARTESIAN_POINT ( 'NONE',  ( -210.7172313291012529, 103.7585653882801182, -5.000000000000004441 ) ) ;
#5846=DIRECTION ( 'NONE',  ( -0.8018642810807398158, -0.5975062131282554700, 0.000000000000000000 ) ) ;
#5850=DIRECTION ( 'NONE',  ( 1.000000000000000000, 0.000000000000000000, 0.000000000000000000 ) ) ;
#5853=CARTESIAN_POINT ( 'NONE',  ( -229.3359862820369699, 89.05815699785955530, 15.38749228882161368 ) ) ;
#5855=CARTESIAN_POINT ( 'NONE',  ( -175.8417606860892874, 246.9430296707336652, -13.00000000000000000 ) ) ;
#5857=VERTEX_POINT ( 'NONE', #430 ) ;
#5862=EDGE_LOOP ( 'NONE', ( #25128, #18581, #23038, #16492 ) ) ;
#5864=CARTESIAN_POINT ( 'NONE',  ( 98.85598102458322955, 241.6222630368573050, -21.45481330788184238 ) ) ;
#5865=ORIENTED_EDGE ( 'NONE', *, *, #17352, .T. ) ;
#5868=ORIENTED_EDGE ( 'NONE', *, *, #24018, .T. ) ;
#5871=ORIENTED_EDGE ( 'NONE', *, *, #20568, .T. ) ;
#5874=ADVANCED_FACE ( 'NONE', ( #11790 ), #24985, .F. ) ;
#5878=EDGE_CURVE ( 'NONE', #10474, #20004, #13755, .T. ) ;
#5879=CARTESIAN_POINT ( 'NONE',  ( 109.8784163943440859, 256.7827724119275103, -42.21295053313544088 ) ) ;
#5880=CARTESIAN_POINT ( 'NONE',  ( -6.888137583864597957, 131.5152179544879800, -16.22191523157399473 ) ) ;
#5883=CARTESIAN_POINT ( 'NONE',  ( -208.9840953169581894, 74.56930307094893351, -36.91869771329891847 ) ) ;
#5886=DIRECTION ( 'NONE',  ( 0.000000000000000000, 1.000000000000000000, 0.000000000000000000 ) ) ;
#5887=EDGE_CURVE ( 'NONE', #11179, #3789, #9193, .T. ) ;
#5893=CIRCLE ( 'NONE', #7736, 5.000000000000004441 ) ;
#5898=CONICAL_SURFACE ( 'NONE', #7310, 14.64217782292691261, 0.08885387018394190484 ) ;
#5905=ADVANCED_FACE ( 'NONE', ( #15814 ), #24558, .F. ) ;
#5906=CARTESIAN_POINT ( 'NONE',  ( 108.4328498615424508, 248.8771578154930069, 35.32563474708244655 ) ) ;
#5907=CIRCLE ( 'NONE', #7766, 50.00000000000000000 ) ;
#5909=CARTESIAN_POINT ( 'NONE',  ( -183.2710533429381883, 107.9500601985746897, -30.83634108471951762 ) ) ;
#5915=DIRECTION ( 'NONE',  ( -1.000000000000000000, 0.000000000000000000, 0.000000000000000000 ) ) ;
#5916=DIRECTION ( 'NONE',  ( 0.5804519453834706688, -0.8142945039115421224, 0.000000000000000000 ) ) ;
#5917=CARTESIAN_POINT ( 'NONE',  ( 134.9999999999998579, 220.0000000000000284, 99.00000000000001421 ) ) ;
#5918=CARTESIAN_POINT ( 'NONE',  ( -180.0000000000000284, -40.00000000000004974, -70.00000000000001421 ) ) ;
#5922=CARTESIAN_POINT ( 'NONE',  ( -196.6548244826268785, 98.17949491351788538, -32.15600783193318080 ) ) ;
#5932=CARTESIAN_POINT ( 'NONE',  ( -28.05246235954390244, 188.0718642840173516, -15.00000000000000000 ) ) ;
#5934=CARTESIAN_POINT ( 'NONE',  ( -208.4828279284123482, 89.67248562427096203, 24.76657354760775220 ) ) ;
#5940=DIRECTION ( 'NONE',  ( 1.000000000000000000, 0.000000000000000000, 0.000000000000000000 ) ) ;
#5942=ORIENTED_EDGE ( 'NONE', *, *, #21515, .F. ) ;
#5945=EDGE_CURVE ( 'NONE', #22383, #11368, #6774, .T. ) ;
#5948=ADVANCED_FACE ( 'NONE', ( #20813 ), #17062, .T. ) ;
#5953=DIRECTION ( 'NONE',  ( -2.312964634635743450E-16, 1.000000000000000000, 0.000000000000000000 ) ) ;
#5954=CARTESIAN_POINT ( 'NONE',  ( -175.0000000000000000, -150.0000000000000853, 64.00000000000002842 ) ) ;
#5959=CARTESIAN_POINT ( 'NONE',  ( 119.9999999999999147, 236.7705098312484893, -100.0000000000000284 ) ) ;
#5960=VERTEX_POINT ( 'NONE', #16511 ) ;
#5967=DIRECTION ( 'NONE',  ( -0.000000000000000000, -0.000000000000000000, 1.000000000000000000 ) ) ;
#5973=AXIS2_PLACEMENT_3D ( 'NONE', #10413, #14450, #8259 ) ;
#5974=CARTESIAN_POINT ( 'NONE',  ( -236.2689932932674424, 81.43917303656978390, 15.00000000000000355 ) ) ;
#5978=ORIENTED_EDGE ( 'NONE', *, *, #11674, .T. ) ;
#5979=CARTESIAN_POINT ( 'NONE',  ( -92.90453691731501351, 136.4113017735256221, 13.49169152925984427 ) ) ;
#5984=VERTEX_POINT ( 'NONE', #19080 ) ;
#5985=DIRECTION ( 'NONE',  ( 1.000000000000000000, 0.000000000000000000, 0.000000000000000000 ) ) ;
#5989=DIRECTION ( 'NONE',  ( -1.000000000000000000, -8.673617379884036705E-17, 0.000000000000000000 ) ) ;
#5992=CARTESIAN_POINT ( 'NONE',  ( 21.78408758738015294, -47.59365313163254285, 99.02387345699440857 ) ) ;
#5993=CARTESIAN_POINT ( 'NONE',  ( -220.9594934662428614, 86.32379293724815739, -18.24975661118741499 ) ) ;
#5994=CIRCLE ( 'NONE', #28, 4.999999999999997335 ) ;
#5999=PLANE ( 'NONE',  #10249 ) ;
#6000=ORIENTED_EDGE ( 'NONE', *, *, #19170, .F. ) ;
#6004=CARTESIAN_POINT ( 'NONE',  ( 119.9999999999999147, 236.7705098312484893, 100.0000000000000142 ) ) ;
#6006=EDGE_LOOP ( 'NONE', ( #17833, #13166, #16765, #17256 ) ) ;
#6008=EDGE_CURVE ( 'NONE', #25446, #4407, #24276, .T. ) ;
#6009=CARTESIAN_POINT ( 'NONE',  ( 90.84405255075068908, 240.0000000000000568, -6.597066685413930820 ) ) ;
#6010=ORIENTED_EDGE ( 'NONE', *, *, #19276, .T. ) ;
#6011=ORIENTED_EDGE ( 'NONE', *, *, #9459, .F. ) ;
#6012=ORIENTED_EDGE ( 'NONE', *, *, #16045, .T. ) ;
#6013=AXIS2_PLACEMENT_3D ( 'NONE', #16982, #567, #12829 ) ;
#6021=DIRECTION ( 'NONE',  ( 0.000000000000000000, 0.000000000000000000, -1.000000000000000000 ) ) ;
#6022=DIRECTION ( 'NONE',  ( 0.000000000000000000, -1.000000000000000000, -2.498359269027536814E-16 ) ) ;
#6023=LINE ( 'NONE', #18542, #23409 ) ;
#6026=DIRECTION ( 'NONE',  ( 1.000000000000000000, -1.902611372570518757E-15, 0.000000000000000000 ) ) ;
#6032=CARTESIAN_POINT ( 'NONE',  ( -233.2943309833541718, 92.06151970357194614, 15.00000000000000000 ) ) ;
#6034=ORIENTED_EDGE ( 'NONE', *, *, #8976, .T. ) ;
#6036=CARTESIAN_POINT ( 'NONE',  ( 116.2405502098322501, 232.4361285658575014, -99.27293966533116532 ) ) ;
#6038=AXIS2_PLACEMENT_3D ( 'NONE', #1100, #13770, #2824 ) ;
#6042=EDGE_CURVE ( 'NONE', #26112, #20676, #12212, .T. ) ;
#6043=ORIENTED_EDGE ( 'NONE', *, *, #20240, .F. ) ;
#6048=ORIENTED_EDGE ( 'NONE', *, *, #10170, .T. ) ;
#6051=CARTESIAN_POINT ( 'NONE',  ( 105.9596802632211450, 242.8245672004252924, 29.94426634347210125 ) ) ;
#6052=CARTESIAN_POINT ( 'NONE',  ( -191.3965535058103171, 102.3881842207307358, -32.04908598840737000 ) ) ;
#6058=LINE ( 'NONE', #1463, #6571 ) ;
#6062=CARTESIAN_POINT ( 'NONE',  ( -186.8209274618468498, 105.3754588275796209, -32.54694188853392234 ) ) ;
#6065=( BOUNDED_SURFACE ( )  B_SPLINE_SURFACE ( 3, 2, ( 
 ( #16012, #489, #4783 ),
 ( #910, #25046, #5072 ),
 ( #9250, #5356, #14137 ),
 ( #26914, #9679, #635 ),
 ( #18439, #13862, #20449 ),
 ( #26773, #2480, #4923 ),
 ( #27190, #20302, #9401 ),
 ( #16152, #7529, #773 ),
 ( #26615, #6940, #20014 ),
 ( #18012, #11268, #7092 ),
 ( #16292, #7239, #24765 ),
 ( #15873, #22751, #24904 ),
 ( #15726, #24619, #347 ),
 ( #27050, #22611, #3056 ),
 ( #22465, #13716, #2773 ),
 ( #18158, #2921, #11705 ),
 ( #9540, #13569, #5217 ),
 ( #18300, #14004, #9105 ),
 ( #7384, #17863, #11842 ),
 ( #22320, #11416, #2627 ),
 ( #20587, #20161, #16844 ),
 ( #27321, #11982, #19133 ),
 ( #26128, #27458, #8078 ),
 ( #27599, #7937, #25178 ) ),
 .UNSPECIFIED., .F., .F., .F. ) 
 B_SPLINE_SURFACE_WITH_KNOTS ( ( 4, 2, 2, 2, 2, 2, 2, 2, 2, 2, 2, 4 ),
 ( 3, 3 ),
 ( -3.469446951953614189E-18, 0.006932175204370943401, 0.01386435040874189027, 0.01733043801092736327, 0.02079652561311283801, 0.02772870081748378401, 0.03466087602185473349, 0.03639391982294747085, 0.03812696362404020822, 0.04159305122622568296, 0.04852522643059663243, 0.05545740163496757497 ),
 ( 0.000000000000000000, 1.000000000000000000 ),
 .UNSPECIFIED. ) 
 GEOMETRIC_REPRESENTATION_ITEM ( )  RATIONAL_B_SPLINE_SURFACE ( (
 ( 1.000000000000000000, 0.7071067811865475727, 1.000000000000000000),
 ( 1.000000000000000000, 0.7196205501095098711, 1.000000000000000000),
 ( 1.000000000000000000, 0.7318467739635132752, 1.000000000000000000),
 ( 1.000000000000000000, 0.7550137444392899244, 1.000000000000000000),
 ( 1.000000000000000000, 0.7659551710817132930, 1.000000000000000000),
 ( 1.000000000000000000, 0.7809925864113128613, 1.000000000000000000),
 ( 1.000000000000000000, 0.7857889008458237567, 1.000000000000000000),
 ( 1.000000000000000000, 0.7947914178569325250, 1.000000000000000000),
 ( 1.000000000000000000, 0.7989996273462374177, 1.000000000000000000),
 ( 1.000000000000000000, 0.8107003658405596003, 1.000000000000000000),
 ( 1.000000000000000000, 0.8172691060501307003, 1.000000000000000000),
 ( 1.000000000000000000, 0.8277221977076023585, 1.000000000000000000),
 ( 1.000000000000000000, 0.8316078875901102840, 1.000000000000000000),
 ( 1.000000000000000000, 0.8346398751107367842, 1.000000000000000000),
 ( 1.000000000000000000, 0.8351546698963130400, 1.000000000000000000),
 ( 1.000000000000000000, 0.8359930079802355696, 1.000000000000000000),
 ( 1.000000000000000000, 0.8363177555487408821, 1.000000000000000000),
 ( 1.000000000000000000, 0.8370113090867827843, 1.000000000000000000),
 ( 1.000000000000000000, 0.8370994751787733668, 1.000000000000000000),
 ( 1.000000000000000000, 0.8362601742890978240, 1.000000000000000000),
 ( 1.000000000000000000, 0.8342295125018783786, 1.000000000000000000),
 ( 1.000000000000000000, 0.8273091872078748299, 1.000000000000000000),
 ( 1.000000000000000000, 0.8224188864783793518, 1.000000000000000000),
 ( 1.000000000000000000, 0.8161343730438194166, 1.000000000000000000) ) ) 
 REPRESENTATION_ITEM ( '' )  SURFACE ( )  );
#6066=LINE ( 'NONE', #6208, #1409 ) ;
#6072=CARTESIAN_POINT ( 'NONE',  ( 115.9275995189148318, 231.9502961609913143, 99.13875753836930471 ) ) ;
#6075=DIRECTION ( 'NONE',  ( 1.000000000000000000, -0.000000000000000000, 0.000000000000000000 ) ) ;
#6079=FACE_OUTER_BOUND ( 'NONE', #25799, .T. ) ;
#6085=ORIENTED_EDGE ( 'NONE', *, *, #1641, .T. ) ;
#6086=EDGE_LOOP ( 'NONE', ( #7061, #7339, #23901, #24077 ) ) ;
#6088=VERTEX_POINT ( 'NONE', #16650 ) ;
#6093=EDGE_CURVE ( 'NONE', #18691, #9161, #18782, .T. ) ;
#6096=DIRECTION ( 'NONE',  ( 1.000000000000000000, 8.673617379884036705E-17, 0.000000000000000000 ) ) ;
#6100=DIRECTION ( 'NONE',  ( 1.000000000000000000, 1.850371707708592344E-16, 0.000000000000000000 ) ) ;
#6101=CARTESIAN_POINT ( 'NONE',  ( -239.6893155506592166, 70.91029463948937916, -5.253362301615601027 ) ) ;
#6104=EDGE_CURVE ( 'NONE', #17036, #6791, #16051, .T. ) ;
#6105=CARTESIAN_POINT ( 'NONE',  ( -227.8378063125350650, 130.6400894613935293, 12.99999999999999822 ) ) ;
#6106=DIRECTION ( 'NONE',  ( -1.000000000000000000, 0.000000000000000000, 0.000000000000000000 ) ) ;
#6107=CARTESIAN_POINT ( 'NONE',  ( -24.33210486176665910, 0.000000000000000000, 100.0000000000000000 ) ) ;
#6108=ORIENTED_EDGE ( 'NONE', *, *, #13682, .T. ) ;
#6110=CARTESIAN_POINT ( 'NONE',  ( 0.000000000000000000, 75.97823757117562593, 100.0000000000000000 ) ) ;
#6112=EDGE_CURVE ( 'NONE', #17545, #7637, #21076, .T. ) ;
#6113=CARTESIAN_POINT ( 'NONE',  ( 39.99999999999995026, -19.99999999999983302, 110.0000000000000284 ) ) ;
#6125=VECTOR ( 'NONE', #9297, 1000.000000000000000 ) ;
#6127=CARTESIAN_POINT ( 'NONE',  ( -85.28599540134722190, 134.8026027455211988, 15.45364094122273002 ) ) ;
#6131=CARTESIAN_POINT ( 'NONE',  ( -90.06590765905433216, 134.7839249153333583, -15.45693337243942267 ) ) ;
#6133=CARTESIAN_POINT ( 'NONE',  ( -127.8679930504526538, 131.6610752695499400, -14.66658078038128998 ) ) ;
#6139=CARTESIAN_POINT ( 'NONE',  ( -222.9992919783725824, 86.62858596284870316, -17.32510164567526800 ) ) ;
#6141=DIRECTION ( 'NONE',  ( 1.000000000000000000, 0.000000000000000000, 0.000000000000000000 ) ) ;
#6143=CARTESIAN_POINT ( 'NONE',  ( -209.3833921019910349, 88.44299030055611865, 25.74621063874961280 ) ) ;
#6146=DIRECTION ( 'NONE',  ( 1.000000000000000000, 0.000000000000000000, 0.000000000000000000 ) ) ;
#6149=EDGE_CURVE ( 'NONE', #28035, #15436, #10363, .T. ) ;
#6151=CARTESIAN_POINT ( 'NONE',  ( -143.6428522700808230, 71.54464929955099706, 83.00000000000001421 ) ) ;
#6156=CARTESIAN_POINT ( 'NONE',  ( 96.93828241644565935, 232.7455409703808016, -20.22303902613517579 ) ) ;
#6161=ORIENTED_EDGE ( 'NONE', *, *, #5673, .T. ) ;
#6165=CARTESIAN_POINT ( 'NONE',  ( 179.9999999999999147, 330.0000000000000000, 84.99999999999995737 ) ) ;
#6166=DIRECTION ( 'NONE',  ( 1.000000000000000000, -0.000000000000000000, -0.000000000000000000 ) ) ;
#6167=DIRECTION ( 'NONE',  ( 1.000000000000000000, -0.000000000000000000, -0.000000000000000000 ) ) ;
#6169=ADVANCED_FACE ( 'NONE', ( #8452 ), #13317, .T. ) ;
#6172=CARTESIAN_POINT ( 'NONE',  ( -225.9870166515752601, 72.66138222772276833, -17.86717049014344383 ) ) ;
#6174=CARTESIAN_POINT ( 'NONE',  ( -40.35410369946821163, 130.4208408520967168, 15.14572397854045249 ) ) ;
#6177=PLANE ( 'NONE',  #6974 ) ;
#6178=CIRCLE ( 'NONE', #15365, 9.999999999999996447 ) ;
#6180=CARTESIAN_POINT ( 'NONE',  ( -178.0751036719780132, 111.1757337266472518, 28.96268686395388059 ) ) ;
#6183=DIRECTION ( 'NONE',  ( 0.000000000000000000, 0.000000000000000000, 1.000000000000000000 ) ) ;
#6188=CARTESIAN_POINT ( 'NONE',  ( 79.99999999999991473, 110.0000000000000142, 100.0000000000000142 ) ) ;
#6189=CARTESIAN_POINT ( 'NONE',  ( 79.99999999999995737, 59.99999999999998579, 15.00000000000000000 ) ) ;
#6190=ORIENTED_EDGE ( 'NONE', *, *, #14879, .F. ) ;
#6192=ORIENTED_EDGE ( 'NONE', *, *, #5498, .F. ) ;
#6193=EDGE_CURVE ( 'NONE', #7297, #2370, #6430, .T. ) ;
#6194=CARTESIAN_POINT ( 'NONE',  ( 96.92716526686170653, 115.1868982021059935, -100.0000000000216716 ) ) ;
#6196=CARTESIAN_POINT ( 'NONE',  ( 99.70645294041088391, 234.7926843489850057, 22.37568098243790971 ) ) ;
#6198=ORIENTED_EDGE ( 'NONE', *, *, #5299, .F. ) ;
#6199=CARTESIAN_POINT ( 'NONE',  ( -207.3017215893796106, 90.23546665973240977, 26.80608177402522685 ) ) ;
#6201=CYLINDRICAL_SURFACE ( 'NONE', #18970, 5.999999999999991118 ) ;
#6202=FACE_OUTER_BOUND ( 'NONE', #215, .T. ) ;
#6206=FACE_OUTER_BOUND ( 'NONE', #7500, .T. ) ;
#6208=CARTESIAN_POINT ( 'NONE',  ( -412.2374841615667833, -120.0000000000002558, 100.0000000000000142 ) ) ;
#6213=CARTESIAN_POINT ( 'NONE',  ( 119.9999999999999147, 236.7705098312484893, 100.0000000000000142 ) ) ;
#6223=CARTESIAN_POINT ( 'NONE',  ( -185.4353359813156601, 106.5295224582049372, -31.86382914232619257 ) ) ;
#6225=VERTEX_POINT ( 'NONE', #9451 ) ;
#6227=VERTEX_POINT ( 'NONE', #11321 ) ;
#6228=VECTOR ( 'NONE', #24130, 1000.000000000000000 ) ;
#6231=VECTOR ( 'NONE', #2757, 1000.000000000000000 ) ;
#6237=SPHERICAL_SURFACE ( 'NONE', #20822, 30.00000000000000000 ) ;
#6240=DIRECTION ( 'NONE',  ( 1.000000000000000000, 0.000000000000000000, 0.000000000000000000 ) ) ;
#6241=FACE_OUTER_BOUND ( 'NONE', #2915, .T. ) ;
#6242=CARTESIAN_POINT ( 'NONE',  ( -233.5270925705994500, 66.28764270639172196, -15.64035431904813045 ) ) ;
#6243=EDGE_LOOP ( 'NONE', ( #22004, #1803, #17882, #28030 ) ) ;
#6246=DIRECTION ( 'NONE',  ( -0.000000000000000000, -0.000000000000000000, 1.000000000000000000 ) ) ;
#6252=CARTESIAN_POINT ( 'NONE',  ( -12.24491960465745599, 75.97823757117562593, 95.00000000000000000 ) ) ;
#6260=EDGE_LOOP ( 'NONE', ( #25691, #3432, #13702, #25861 ) ) ;
#6263=CARTESIAN_POINT ( 'NONE',  ( -81.50071837300136224, 134.7411680033590358, 15.46448801347469981 ) ) ;
#6265=EDGE_CURVE ( 'NONE', #7514, #6925, #27500, .T. ) ;
#6266=ORIENTED_EDGE ( 'NONE', *, *, #17104, .F. ) ;
#6267=CARTESIAN_POINT ( 'NONE',  ( 109.9999999999999147, 140.0000000000000000, -45.00000000000000000 ) ) ;
#6270=EDGE_CURVE ( 'NONE', #7659, #12559, #25686, .T. ) ;
#6272=CARTESIAN_POINT ( 'NONE',  ( -108.0095164744623730, 135.2230479792049493, -13.71926593627200397 ) ) ;
#6273=CARTESIAN_POINT ( 'NONE',  ( -141.6428522700808230, 74.54464929955099706, 83.00000000000001421 ) ) ;
#6277=CARTESIAN_POINT ( 'NONE',  ( -229.7952689998928690, 91.77895247750312535, -15.17557543154750910 ) ) ;
#6287=ORIENTED_EDGE ( 'NONE', *, *, #11206, .T. ) ;
#6288=CARTESIAN_POINT ( 'NONE',  ( 102.7763551498842816, 237.8836077948904517, -25.40199625708464382 ) ) ;
#6296=ORIENTED_EDGE ( 'NONE', *, *, #7625, .F. ) ;
#6297=ORIENTED_EDGE ( 'NONE', *, *, #12021, .F. ) ;
#6301=DIRECTION ( 'NONE',  ( 1.000000000000000000, 4.163336342344337027E-16, -0.000000000000000000 ) ) ;
#6303=CARTESIAN_POINT ( 'NONE',  ( -180.0000000000000284, -2.775557561562891982E-14, -70.00000000000001421 ) ) ;
#6304=CIRCLE ( 'NONE', #26029, 22.49999999999997868 ) ;
#6306=DIRECTION ( 'NONE',  ( 0.000000000000000000, 0.000000000000000000, -1.000000000000000000 ) ) ;
#6309=CARTESIAN_POINT ( 'NONE',  ( -236.2685473594162602, 81.43844187475562535, -14.99999999999999822 ) ) ;
#6310=CARTESIAN_POINT ( 'NONE',  ( -24.72692578937659036, 129.2488030442671914, 16.96197069768293986 ) ) ;
#6311=CARTESIAN_POINT ( 'NONE',  ( -209.9968669296227972, 60.57716416197344245, 21.99717788492469595 ) ) ;
#6315=CARTESIAN_POINT ( 'NONE',  ( -168.2126854711127635, 116.6621084685910574, 24.58429559685009380 ) ) ;
#6316=DIRECTION ( 'NONE',  ( 1.000000000000000000, -1.832271836300406591E-15, 0.000000000000000000 ) ) ;
#6321=ORIENTED_EDGE ( 'NONE', *, *, #14801, .F. ) ;
#6325=LINE ( 'NONE', #6189, #9010 ) ;
#6328=ORIENTED_EDGE ( 'NONE', *, *, #26630, .T. ) ;
#6329=CARTESIAN_POINT ( 'NONE',  ( 101.7779539752773275, 119.2876405402304982, -100.0000000000216716 ) ) ;
#6330=CARTESIAN_POINT ( 'NONE',  ( 89.55286837137404632, 230.0961515142736573, 16.54242047486848932 ) ) ;
#6331=EDGE_CURVE ( 'NONE', #5762, #14227, #24778, .T. ) ;
#6334=CARTESIAN_POINT ( 'NONE',  ( -226.8383669992199430, 90.02672605029661668, 13.69137186706111997 ) ) ;
#6338=CIRCLE ( 'NONE', #26066, 4.355764593064429313 ) ;
#6339=DIRECTION ( 'NONE',  ( -0.2458199939946738577, -0.9693154958796741383, 0.000000000000000000 ) ) ;
#6347=DIRECTION ( 'NONE',  ( 1.000000000000000000, -0.000000000000000000, -0.000000000000000000 ) ) ;
#6350=EDGE_CURVE ( 'NONE', #20577, #1393, #922, .T. ) ;
#6353=DIRECTION ( 'NONE',  ( 1.000000000000000000, 0.000000000000000000, 0.000000000000000000 ) ) ;
#6354=CARTESIAN_POINT ( 'NONE',  ( -229.6313009160351442, 91.61680614984454962, 13.11372941846348361 ) ) ;
#6361=CARTESIAN_POINT ( 'NONE',  ( -175.2889320536586979, 112.8162159305347814, -27.79264103675363629 ) ) ;
#6363=ORIENTED_EDGE ( 'NONE', *, *, #4122, .T. ) ;
#6364=CARTESIAN_POINT ( 'NONE',  ( -112.7754610104328634, 70.85428810103185526, 82.84745292188917176 ) ) ;
#6365=ORIENTED_EDGE ( 'NONE', *, *, #17792, .F. ) ;
#6366=CIRCLE ( 'NONE', #24734, 22.49999999999997868 ) ;
#6369=VECTOR ( 'NONE', #25558, 1000.000000000000000 ) ;
#6371=ORIENTED_EDGE ( 'NONE', *, *, #16437, .T. ) ;
#6381=CARTESIAN_POINT ( 'NONE',  ( -224.2911920753269897, 72.03214051461351630, -18.76861173148824591 ) ) ;
#6382=EDGE_LOOP ( 'NONE', ( #26483, #21417, #14008, #23224 ) ) ;
#6383=VECTOR ( 'NONE', #5368, 1000.000000000000000 ) ;
#6385=CIRCLE ( 'NONE', #896, 19.99999999999998934 ) ;
#6390=EDGE_CURVE ( 'NONE', #17712, #14597, #19263, .T. ) ;
#6392=AXIS2_PLACEMENT_3D ( 'NONE', #25404, #21658, #13059 ) ;
#6393=CARTESIAN_POINT ( 'NONE',  ( 33.10302365956999182, 221.6666220619077876, 12.99999999999999822 ) ) ;
#6395=DIRECTION ( 'NONE',  ( -0.9654425086906593956, 0.2448377981135679560, -0.08930405941493296806 ) ) ;
#6401=SPHERICAL_SURFACE ( 'NONE', #22626, 5.000000000000000000 ) ;
#6405=EDGE_CURVE ( 'NONE', #12131, #17425, #1369, .T. ) ;
#6406=ORIENTED_EDGE ( 'NONE', *, *, #28394, .F. ) ;
#6407=CARTESIAN_POINT ( 'NONE',  ( -76.25760768171835480, 219.6666220619077876, -13.00000000000000000 ) ) ;
#6408=VECTOR ( 'NONE', #27165, 1000.000000000000114 ) ;
#6410=( BOUNDED_SURFACE ( )  B_SPLINE_SURFACE ( 3, 2, ( 
 ( #6553, #15189, #21922 ),
 ( #2228, #13315, #22064 ),
 ( #19764, #8851, #19908 ),
 ( #2372, #17609, #11154 ),
 ( #15614, #2094, #26083 ),
 ( #235, #8997, #4253 ),
 ( #28090, #21786, #17750 ),
 ( #23799, #26364, #24357 ),
 ( #6694, #5062, #19626 ),
 ( #2912, #11697, #8435 ) ),
 .UNSPECIFIED., .F., .F., .F. ) 
 B_SPLINE_SURFACE_WITH_KNOTS ( ( 4, 2, 2, 2, 4 ),
 ( 3, 3 ),
 ( 0.000000000000000000, 0.003993085574633960591, 0.007986171149267921182, 0.01197925672390188177, 0.01597234229853584236 ),
 ( 0.000000000000000000, 1.000000000000000000 ),
 .UNSPECIFIED. ) 
 GEOMETRIC_REPRESENTATION_ITEM ( )  RATIONAL_B_SPLINE_SURFACE ( (
 ( 1.000000000000000000, 0.7071067811865441310, 1.000000000000000000),
 ( 1.000000000000000000, 0.6986941146418389481, 1.000000000000000000),
 ( 1.000000000000000000, 0.6922065170597959671, 1.000000000000000000),
 ( 1.000000000000000000, 0.6834952607772883937, 1.000000000000000000),
 ( 1.000000000000000000, 0.6812778029564220406, 1.000000000000000000),
 ( 1.000000000000000000, 0.6812778029564220406, 1.000000000000000000),
 ( 1.000000000000000000, 0.6834952607749916753, 1.000000000000000000),
 ( 1.000000000000000000, 0.6922065170620920194, 1.000000000000000000),
 ( 1.000000000000000000, 0.6986941146401082214, 1.000000000000000000),
 ( 1.000000000000000000, 0.7071067811865499042, 1.000000000000000000) ) ) 
 REPRESENTATION_ITEM ( '' )  SURFACE ( )  );
#6412=CARTESIAN_POINT ( 'NONE',  ( -241.9743096803475453, -91.18033988749901653, -17.46154499483315448 ) ) ;
#6416=FACE_OUTER_BOUND ( 'NONE', #5530, .T. ) ;
#6417=ADVANCED_FACE ( 'NONE', ( #18764 ), #27510, .F. ) ;
#6418=CARTESIAN_POINT ( 'NONE',  ( -175.0000000000000000, -120.0000000000001847, -69.99999999999998579 ) ) ;
#6421=CARTESIAN_POINT ( 'NONE',  ( -42.99650729631200363, 71.03850157808263077, 99.00000000000000000 ) ) ;
#6425=FACE_OUTER_BOUND ( 'NONE', #9155, .T. ) ;
#6430=LINE ( 'NONE', #21513, #11479 ) ;
#6436=CIRCLE ( 'NONE', #18, 5.000000000000000888 ) ;
#6437=CARTESIAN_POINT ( 'NONE',  ( 92.04920872067096127, 230.5961997032265174, -17.50980340464030505 ) ) ;
#6440=ORIENTED_EDGE ( 'NONE', *, *, #20583, .T. ) ;
#6441=ORIENTED_EDGE ( 'NONE', *, *, #18188, .F. ) ;
#6442=EDGE_LOOP ( 'NONE', ( #23463, #26285, #12295, #13588 ) ) ;
#6446=AXIS2_PLACEMENT_3D ( 'NONE', #13045, #383, #9145 ) ;
#6447=DIRECTION ( 'NONE',  ( -1.000000000000000000, 0.000000000000000000, 0.000000000000000000 ) ) ;
#6448=DIRECTION ( 'NONE',  ( 0.000000000000000000, -1.000000000000000000, 0.000000000000000000 ) ) ;
#6451=DIRECTION ( 'NONE',  ( 1.000000000000000000, 8.673617379884036705E-17, 0.000000000000000000 ) ) ;
#6456=CARTESIAN_POINT ( 'NONE',  ( -233.7109140654491171, 78.16279237795507129, -15.26611692692816824 ) ) ;
#6457=CARTESIAN_POINT ( 'NONE',  ( -68.57415822541635464, 80.97823757117562593, 95.00000000000000000 ) ) ;
#6463=ORIENTED_EDGE ( 'NONE', *, *, #24834, .T. ) ;
#6464=CARTESIAN_POINT ( 'NONE',  ( -224.8814028220360797, 87.10059759008312597, -16.59626922761215795 ) ) ;
#6465=EDGE_CURVE ( 'NONE', #13456, #11112, #21094, .T. ) ;
#6471=ORIENTED_EDGE ( 'NONE', *, *, #17845, .T. ) ;
#6472=VERTEX_POINT ( 'NONE', #10855 ) ;
#6477=CARTESIAN_POINT ( 'NONE',  ( 98.15430812615089451, 116.0637945823775112, -78.75000000033432457 ) ) ;
#6478=CARTESIAN_POINT ( 'NONE',  ( -162.6958652128487586, 119.3823555589419669, -22.14487429185738421 ) ) ;
#6480=CARTESIAN_POINT ( 'NONE',  ( -211.3786312416644364, 87.57134810217682741, 24.25168111795433390 ) ) ;
#6483=AXIS2_PLACEMENT_3D ( 'NONE', #101, #24101, #19919 ) ;
#6494=DIRECTION ( 'NONE',  ( 0.000000000000000000, 1.000000000000000000, 0.000000000000000000 ) ) ;
#6497=EDGE_CURVE ( 'NONE', #27076, #2009, #8715, .T. ) ;
#6504=CARTESIAN_POINT ( 'NONE',  ( -216.4421519707229891, 141.6000904446840707, -15.00000000000000000 ) ) ;
#6505=CARTESIAN_POINT ( 'NONE',  ( -188.6691793476254020, 104.3291597953724761, -32.37965609178030491 ) ) ;
#6507=AXIS2_PLACEMENT_3D ( 'NONE', #891, #7223, #18145 ) ;
#6509=ORIENTED_EDGE ( 'NONE', *, *, #23129, .F. ) ;
#6512=FACE_OUTER_BOUND ( 'NONE', #24004, .T. ) ;
#6514=ORIENTED_EDGE ( 'NONE', *, *, #12535, .F. ) ;
#6515=CARTESIAN_POINT ( 'NONE',  ( -13.43082424514546069, 129.5962963036035944, 16.85783026249312400 ) ) ;
#6520=AXIS2_PLACEMENT_3D ( 'NONE', #11696, #16420, #23015 ) ;
#6523=ADVANCED_FACE ( 'NONE', ( #28216 ), #27929, .T. ) ;
#6524=ORIENTED_EDGE ( 'NONE', *, *, #28294, .T. ) ;
#6528=AXIS2_PLACEMENT_3D ( 'NONE', #22127, #4738, #4315 ) ;
#6533=CARTESIAN_POINT ( 'NONE',  ( -160.0000000000000284, 59.99999999999994316, -70.00000000000001421 ) ) ;
#6535=CARTESIAN_POINT ( 'NONE',  ( -125.2895325436294058, 200.2180533211638362, -15.00000000000000000 ) ) ;
#6542=CARTESIAN_POINT ( 'NONE',  ( -225.9974328972257069, 72.66572410194898168, 17.86196565642464051 ) ) ;
#6543=ORIENTED_EDGE ( 'NONE', *, *, #11101, .F. ) ;
#6549=CARTESIAN_POINT ( 'NONE',  ( 109.9999999999999005, 3.816391647148972452E-14, -25.00000000000000000 ) ) ;
#6551=ORIENTED_EDGE ( 'NONE', *, *, #28012, .F. ) ;
#6553=CARTESIAN_POINT ( 'NONE',  ( -227.8378063125350650, 130.6400894613935293, 13.00000000000000000 ) ) ;
#6556=CARTESIAN_POINT ( 'NONE',  ( 89.99999999999988631, 240.0000000000000284, 6.270166537925822681 ) ) ;
#6558=EDGE_CURVE ( 'NONE', #5346, #18031, #21477, .T. ) ;
#6559=CIRCLE ( 'NONE', #10797, 7.500000000000007105 ) ;
#6561=CARTESIAN_POINT ( 'NONE',  ( -254.3350114625770289, -91.18033988749901653, 0.000000000000000000 ) ) ;
#6562=CARTESIAN_POINT ( 'NONE',  ( -59.48697296830715686, 2.336311854928213219E-15, 99.00000000000000000 ) ) ;
#6564=CARTESIAN_POINT ( 'NONE',  ( -210.7125095212385020, 88.79578285577181873, -22.86806245198074450 ) ) ;
#6565=CARTESIAN_POINT ( 'NONE',  ( -160.0000000000000284, 59.99999999999994316, 45.00000000000000000 ) ) ;
#6571=VECTOR ( 'NONE', #23164, 1000.000000000000000 ) ;
#6575=CARTESIAN_POINT ( 'NONE',  ( 109.9999999999999147, 140.0000000000000000, 45.00000000000000000 ) ) ;
#6577=VECTOR ( 'NONE', #6846, 1000.000000000000000 ) ;
#6586=AXIS2_PLACEMENT_3D ( 'NONE', #23874, #6626, #24017 ) ;
#6589=CYLINDRICAL_SURFACE ( 'NONE', #5493, 5.999999999999991118 ) ;
#6590=CIRCLE ( 'NONE', #4294, 6.204828372381208546 ) ;
#6592=CARTESIAN_POINT ( 'NONE',  ( 156.4999999999998579, 220.0000000000000284, 99.00000000000001421 ) ) ;
#6593=EDGE_CURVE ( 'NONE', #18456, #5833, #8636, .T. ) ;
#6594=CARTESIAN_POINT ( 'NONE',  ( -205.1716483941798401, 60.34345434848681577, 21.58965668827011442 ) ) ;
#6595=CARTESIAN_POINT ( 'NONE',  ( 109.9999999999999147, 140.0000000000000000, -45.00000000000000000 ) ) ;
#6596=CARTESIAN_POINT ( 'NONE',  ( -180.0000000000000284, -70.00000000000004263, 100.0000000000000142 ) ) ;
#6599=ADVANCED_FACE ( 'NONE', ( #504 ), #2279, .F. ) ;
#6601=CARTESIAN_POINT ( 'NONE',  ( -231.0575465263486308, 75.69719229554537776, -15.88027955539508440 ) ) ;
#6604=CARTESIAN_POINT ( 'NONE',  ( -177.8141338791984651, 110.9804198039069263, 30.03957269548647346 ) ) ;
#6607=EDGE_LOOP ( 'NONE', ( #20787, #21320, #14748, #24217 ) ) ;
#6608=AXIS2_PLACEMENT_3D ( 'NONE', #21756, #23625, #26054 ) ;
#6609=CARTESIAN_POINT ( 'NONE',  ( -232.7323212076349535, 91.52112961950480496, -14.99999999999997513 ) ) ;
#6611=ORIENTED_EDGE ( 'NONE', *, *, #4319, .T. ) ;
#6613=AXIS2_PLACEMENT_3D ( 'NONE', #16853, #4047, #2038 ) ;
#6614=ORIENTED_EDGE ( 'NONE', *, *, #28115, .F. ) ;
#6616=CARTESIAN_POINT ( 'NONE',  ( -138.6428522700808230, 66.54464929955099706, 83.00000000000001421 ) ) ;
#6620=CARTESIAN_POINT ( 'NONE',  ( 100.5794065448618255, 118.1137289703157336, -99.99999999995674216 ) ) ;
#6621=CARTESIAN_POINT ( 'NONE',  ( -189.8086322075389774, 92.49158130768422836, -13.00000000000000000 ) ) ;
#6624=CARTESIAN_POINT ( 'NONE',  ( -210.7121506535087576, 88.79643741746845365, 22.86845985951527993 ) ) ;
#6625=AXIS2_PLACEMENT_3D ( 'NONE', #10238, #18995, #5916 ) ;
#6626=DIRECTION ( 'NONE',  ( -0.000000000000000000, 1.000000000000000000, -1.387778780781445429E-16 ) ) ;
#6627=ADVANCED_FACE ( 'NONE', ( #26632 ), #7255, .F. ) ;
#6629=B_SPLINE_CURVE_WITH_KNOTS ( 'NONE', 3,
 ( #25560, #10344, #23413, #8046, #18680, #22994, #3444, #14807, #3869, #5883, #12513, #16536, #9790, #18545, #27292, #21256, #5462, #1577, #14246, #3299, #1156, #25285, #23136, #12237, #17658, #2139, #13222, #6172, #21539, #14949, #23702, #13084, #8474, #6601, #19246, #17231, #21966, #6456, #4008, #11057, #6309, #15087 ),
 .UNSPECIFIED., .F., .F.,
 ( 4, 2, 2, 2, 2, 2, 2, 2, 2, 2, 2, 2, 2, 2, 2, 2, 2, 2, 2, 2, 4 ),
 ( 0.000000000000000000, 0.001589323840935409323, 0.003178647681870818646, 0.006357295363741637291, 0.007946619204677041193, 0.009535943045612444227, 0.01271459072748320866, 0.01907188609122478784, 0.02225053377309557309, 0.02542918145496636181, 0.02860782913683715054, 0.03019715297777251714, 0.03178647681870788028, 0.03496512450057859961, 0.03655444834151396621, 0.03814377218244931894, 0.04132241986431998276, 0.04291174370525530773, 0.04450106754619062577, 0.04767971522806119938, 0.05085836290993178688 ),
 .UNSPECIFIED. ) ;
#6630=ADVANCED_FACE ( 'NONE', ( #11431 ), #11722, .F. ) ;
#6641=LINE ( 'NONE', #11246, #20804 ) ;
#6643=ORIENTED_EDGE ( 'NONE', *, *, #24293, .F. ) ;
#6648=CARTESIAN_POINT ( 'NONE',  ( -194.8905955746074881, 99.56818556745220405, -32.54511976914040616 ) ) ;
#6649=ORIENTED_EDGE ( 'NONE', *, *, #9750, .F. ) ;
#6650=AXIS2_PLACEMENT_3D ( 'NONE', #16028, #20322, #11432 ) ;
#6653=EDGE_CURVE ( 'NONE', #14756, #3239, #5485, .T. ) ;
#6655=DIRECTION ( 'NONE',  ( 0.000000000000000000, -0.000000000000000000, 1.000000000000000000 ) ) ;
#6668=ORIENTED_EDGE ( 'NONE', *, *, #27676, .F. ) ;
#6669=FACE_OUTER_BOUND ( 'NONE', #11408, .T. ) ;
#6670=VECTOR ( 'NONE', #13010, 1000.000000000000000 ) ;
#6674=ORIENTED_EDGE ( 'NONE', *, *, #16437, .F. ) ;
#6677=DIRECTION ( 'NONE',  ( -1.000000000000000000, 0.000000000000000000, 0.000000000000000000 ) ) ;
#6678=CARTESIAN_POINT ( 'NONE',  ( -238.3976651326582328, 69.81518760999665574, -5.405651710414773881 ) ) ;
#6679=DIRECTION ( 'NONE',  ( 1.000000000000000000, 0.000000000000000000, 0.000000000000000000 ) ) ;
#6683=DIRECTION ( 'NONE',  ( -0.000000000000000000, -0.000000000000000000, -1.000000000000000000 ) ) ;
#6688=VERTEX_POINT ( 'NONE', #24782 ) ;
#6689=PLANE ( 'NONE',  #16802 ) ;
#6692=CIRCLE ( 'NONE', #3019, 22.49999999999999289 ) ;
#6694=CARTESIAN_POINT ( 'NONE',  ( -216.6285193170544687, 139.2238166778980712, 12.99999999956374275 ) ) ;
#6695=CARTESIAN_POINT ( 'NONE',  ( 94.60831035301521297, 240.0858928317027221, 18.63379520592308936 ) ) ;
#6696=DIRECTION ( 'NONE',  ( 0.000000000000000000, 0.000000000000000000, -1.000000000000000000 ) ) ;
#6699=CARTESIAN_POINT ( 'NONE',  ( 109.9999999999999432, -120.0000000000001279, 25.00000000000000000 ) ) ;
#6700=EDGE_CURVE ( 'NONE', #18691, #17779, #11997, .T. ) ;
#6705=VECTOR ( 'NONE', #14676, 1000.000000000000000 ) ;
#6707=CARTESIAN_POINT ( 'NONE',  ( -115.3221550338875687, 71.54464929955099706, 83.00000000000001421 ) ) ;
#6710=CARTESIAN_POINT ( 'NONE',  ( -217.2892621185082760, 109.4029876883478352, 15.00000000000000000 ) ) ;
#6717=CARTESIAN_POINT ( 'NONE',  ( -33.76020577399351907, 129.4009239033509573, -15.57932736426030118 ) ) ;
#6719=ORIENTED_EDGE ( 'NONE', *, *, #12645, .F. ) ;
#6720=EDGE_LOOP ( 'NONE', ( #20461, #8466, #2321, #21953 ) ) ;
#6724=DIRECTION ( 'NONE',  ( 1.000000000000000000, 0.000000000000000000, 0.000000000000000000 ) ) ;
#6725=DIRECTION ( 'NONE',  ( -1.541976423090495387E-16, 1.000000000000000000, 0.000000000000000000 ) ) ;
#6728=CARTESIAN_POINT ( 'NONE',  ( -213.6504899993254298, 58.00877466446878827, 34.94433424773627905 ) ) ;
#6735=CARTESIAN_POINT ( 'NONE',  ( -40.40953891503691153, 0.000000000000000000, 100.0000000000000000 ) ) ;
#6739=DIRECTION ( 'NONE',  ( 0.000000000000000000, 0.000000000000000000, 1.000000000000000000 ) ) ;
#6744=CARTESIAN_POINT ( 'NONE',  ( -178.9685328442623131, 110.6385515672100581, 29.32315025982155987 ) ) ;
#6747=ORIENTED_EDGE ( 'NONE', *, *, #20444, .F. ) ;
#6750=ADVANCED_FACE ( 'NONE', ( #21017 ), #5371, .F. ) ;
#6754=DIRECTION ( 'NONE',  ( -1.000000000000000000, 0.000000000000000000, 0.000000000000000000 ) ) ;
#6757=CARTESIAN_POINT ( 'NONE',  ( 90.92319367352099846, 112.0484670279005570, -72.65625000014701129 ) ) ;
#6758=DIRECTION ( 'NONE',  ( 0.000000000000000000, 0.000000000000000000, 1.000000000000000000 ) ) ;
#6760=CARTESIAN_POINT ( 'NONE',  ( -223.8831450509237015, 88.82371471167537891, 14.62991863724387542 ) ) ;
#6767=DIRECTION ( 'NONE',  ( -0.000000000000000000, -0.000000000000000000, 1.000000000000000000 ) ) ;
#6774=B_SPLINE_CURVE_WITH_KNOTS ( 'NONE', 3,
 ( #23254, #16789, #16925, #12348, #22971, #18657, #20951, #3557, #23114, #18797 ),
 .UNSPECIFIED., .F., .F.,
 ( 4, 2, 2, 2, 4 ),
 ( 0.000000000000000000, 0.003185215742235096223, 0.006370431484470192446, 0.009555647226705288669, 0.01274086296894038489 ),
 .UNSPECIFIED. ) ;
#6780=ORIENTED_EDGE ( 'NONE', *, *, #16275, .F. ) ;
#6784=ADVANCED_FACE ( 'NONE', ( #3211 ), #3068, .F. ) ;
#6785=DIRECTION ( 'NONE',  ( 0.000000000000000000, 0.000000000000000000, -1.000000000000000000 ) ) ;
#6787=ORIENTED_EDGE ( 'NONE', *, *, #25525, .T. ) ;
#6789=DIRECTION ( 'NONE',  ( -1.850371707708594316E-16, 1.000000000000000000, -0.000000000000000000 ) ) ;
#6791=VERTEX_POINT ( 'NONE', #27337 ) ;
#6792=ORIENTED_EDGE ( 'NONE', *, *, #22342, .F. ) ;
#6800=DIRECTION ( 'NONE',  ( 1.000000000000000000, 0.000000000000000000, 0.000000000000000000 ) ) ;
#6801=CARTESIAN_POINT ( 'NONE',  ( -160.0000000000000284, 139.9999999999999432, -15.00000000000000000 ) ) ;
#6806=DIRECTION ( 'NONE',  ( -0.000000000000000000, -1.000000000000000000, -0.000000000000000000 ) ) ;
#6807=VERTEX_POINT ( 'NONE', #23042 ) ;
#6808=CARTESIAN_POINT ( 'NONE',  ( -227.3759666274727351, 63.27997354833446764, 7.997465051287307780 ) ) ;
#6810=VECTOR ( 'NONE', #5824, 1000.000000000000000 ) ;
#6811=DIRECTION ( 'NONE',  ( 1.000000000000000000, 0.000000000000000000, 0.000000000000000000 ) ) ;
#6815=CARTESIAN_POINT ( 'NONE',  ( 113.4999999999998863, 220.0000000000000284, -100.0000000000000142 ) ) ;
#6816=DIRECTION ( 'NONE',  ( -0.000000000000000000, -0.000000000000000000, -1.000000000000000000 ) ) ;
#6817=ORIENTED_EDGE ( 'NONE', *, *, #13917, .F. ) ;
#6820=CARTESIAN_POINT ( 'NONE',  ( -219.5796349382799519, 71.26926967086903630, 22.06234792876918149 ) ) ;
#6822=EDGE_CURVE ( 'NONE', #21449, #18495, #19735, .T. ) ;
#6824=AXIS2_PLACEMENT_3D ( 'NONE', #20303, #16293, #5357 ) ;
#6829=AXIS2_PLACEMENT_3D ( 'NONE', #22468, #18304, #24768 ) ;
#6833=CARTESIAN_POINT ( 'NONE',  ( 88.05061285011872485, 239.8951213613607365, 16.09479252966118068 ) ) ;
#6834=VECTOR ( 'NONE', #7811, 1000.000000000000000 ) ;
#6835=CARTESIAN_POINT ( 'NONE',  ( -273.6211430000234373, -91.18033988749901653, -14.64217782292691261 ) ) ;
#6836=AXIS2_PLACEMENT_3D ( 'NONE', #15190, #28363, #8575 ) ;
#6837=DIRECTION ( 'NONE',  ( -0.000000000000000000, -0.000000000000000000, 1.000000000000000000 ) ) ;
#6838=DIRECTION ( 'NONE',  ( -0.000000000000000000, -0.000000000000000000, -1.000000000000000000 ) ) ;
#6841=CYLINDRICAL_SURFACE ( 'NONE', #1010, 43.76444293738735070 ) ;
#6842=CARTESIAN_POINT ( 'NONE',  ( -17.24491960465746132, 75.97823757117562593, 95.00000000000000000 ) ) ;
#6844=DIRECTION ( 'NONE',  ( 0.000000000000000000, 0.000000000000000000, -1.000000000000000000 ) ) ;
#6846=DIRECTION ( 'NONE',  ( 0.000000000000000000, 0.000000000000000000, -1.000000000000000000 ) ) ;
#6848=FACE_OUTER_BOUND ( 'NONE', #23215, .T. ) ;
#6849=AXIS2_PLACEMENT_3D ( 'NONE', #12652, #21531, #12928 ) ;
#6850=EDGE_CURVE ( 'NONE', #13481, #23690, #4596, .T. ) ;
#6853=CARTESIAN_POINT ( 'NONE',  ( -210.0000000000000284, 59.99999999999994316, 17.29233506344265336 ) ) ;
#6854=ORIENTED_EDGE ( 'NONE', *, *, #9877, .T. ) ;
#6856=CARTESIAN_POINT ( 'NONE',  ( 109.7119445822053194, 256.4759837302104302, -40.72317850545796603 ) ) ;
#6858=ADVANCED_FACE ( 'NONE', ( #14857 ), #12864, .T. ) ;
#6863=VECTOR ( 'NONE', #12876, 1000.000000000000000 ) ;
#6865=ORIENTED_EDGE ( 'NONE', *, *, #6405, .F. ) ;
#6867=EDGE_LOOP ( 'NONE', ( #16279, #13488, #7411, #17852 ) ) ;
#6869=CARTESIAN_POINT ( 'NONE',  ( -112.3221550338875687, 22.24192588826928585, 80.00000000000001421 ) ) ;
#6875=CARTESIAN_POINT ( 'NONE',  ( -222.1142713347912263, 61.47487629660645325, 10.02481564199105613 ) ) ;
#6880=CARTESIAN_POINT ( 'NONE',  ( -190.0000000000000284, -2.775557561562891982E-14, 98.28427124746191623 ) ) ;
#6882=AXIS2_PLACEMENT_3D ( 'NONE', #1896, #2042, #19291 ) ;
#6883=EDGE_CURVE ( 'NONE', #2675, #25971, #17901, .T. ) ;
#6884=CARTESIAN_POINT ( 'NONE',  ( -7.230610758732472831, 132.9655077820579265, 15.80094727182378023 ) ) ;
#6887=DIRECTION ( 'NONE',  ( 1.000000000000000000, 0.000000000000000000, 0.000000000000000000 ) ) ;
#6889=ORIENTED_EDGE ( 'NONE', *, *, #28214, .T. ) ;
#6890=CARTESIAN_POINT ( 'NONE',  ( -214.7362006204176339, 86.61744048289359910, -21.86430821152871928 ) ) ;
#6892=CARTESIAN_POINT ( 'NONE',  ( -207.2804935778247568, 89.57475743267312396, -27.31082310662946000 ) ) ;
#6893=ORIENTED_EDGE ( 'NONE', *, *, #12211, .F. ) ;
#6895=VERTEX_POINT ( 'NONE', #14994 ) ;
#6897=CARTESIAN_POINT ( 'NONE',  ( 179.9999999999999147, 330.0000000000000000, 100.0000000000000142 ) ) ;
#6898=AXIS2_PLACEMENT_3D ( 'NONE', #23629, #3939, #6240 ) ;
#6899=EDGE_CURVE ( 'NONE', #15077, #2290, #13800, .T. ) ;
#6900=FACE_OUTER_BOUND ( 'NONE', #23005, .T. ) ;
#6903=CARTESIAN_POINT ( 'NONE',  ( 109.9999999999999005, 3.816391647148972452E-14, 100.0000000000000142 ) ) ;
#6905=ORIENTED_EDGE ( 'NONE', *, *, #2402, .F. ) ;
#6906=CARTESIAN_POINT ( 'NONE',  ( -203.7080335011695809, 92.59420371806315586, 28.49755056600432823 ) ) ;
#6908=EDGE_CURVE ( 'NONE', #6688, #4667, #6436, .T. ) ;
#6912=CARTESIAN_POINT ( 'NONE',  ( -198.1081924558745584, 61.84288891412396083, -30.88603804298208644 ) ) ;
#6913=VERTEX_POINT ( 'NONE', #23890 ) ;
#6915=LINE ( 'NONE', #22722, #21044 ) ;
#6919=DIRECTION ( 'NONE',  ( -0.000000000000000000, 0.000000000000000000, 1.000000000000000000 ) ) ;
#6920=EDGE_LOOP ( 'NONE', ( #8074, #22296, #2182, #5332, #8101, #3077 ) ) ;
#6921=FACE_OUTER_BOUND ( 'NONE', #12712, .T. ) ;
#6922=VECTOR ( 'NONE', #16263, 1000.000000000000000 ) ;
#6925=VERTEX_POINT ( 'NONE', #8235 ) ;
#6928=CARTESIAN_POINT ( 'NONE',  ( -160.0000000000000284, 59.99999999999994316, 98.28427124746191623 ) ) ;
#6930=EDGE_LOOP ( 'NONE', ( #12812, #28287, #6463, #21741 ) ) ;
#6931=DIRECTION ( 'NONE',  ( -1.000000000000000000, -0.000000000000000000, 0.000000000000000000 ) ) ;
#6940=CARTESIAN_POINT ( 'NONE',  ( -8.342823007631203325, 132.5495086141303318, -15.90323448772006643 ) ) ;
#6942=DIRECTION ( 'NONE',  ( 1.000000000000000000, 0.000000000000000000, 0.000000000000000000 ) ) ;
#6943=EDGE_CURVE ( 'NONE', #17824, #15830, #4143, .T. ) ;
#6944=CARTESIAN_POINT ( 'NONE',  ( -210.0000000000000284, 59.99999999999993605, -17.29233506344264626 ) ) ;
#6946=CARTESIAN_POINT ( 'NONE',  ( 134.9999999999998579, 220.0000000000000284, 99.00000000000001421 ) ) ;
#6954=CARTESIAN_POINT ( 'NONE',  ( 134.9999999999998579, 220.0000000000000284, -105.0000000000000284 ) ) ;
#6957=ORIENTED_EDGE ( 'NONE', *, *, #23570, .T. ) ;
#6958=( LENGTH_UNIT ( ) NAMED_UNIT ( * ) SI_UNIT ( .MILLI., .METRE. ) );
#6962=TOROIDAL_SURFACE ( 'NONE', #19330, 16.91094714394370158, 6.204828372381208546 ) ;
#6963=CYLINDRICAL_SURFACE ( 'NONE', #2886, 10.00000000000000888 ) ;
#6966=ORIENTED_EDGE ( 'NONE', *, *, #445, .F. ) ;
#6970=EDGE_CURVE ( 'NONE', #16435, #2005, #11947, .T. ) ;
#6971=ORIENTED_EDGE ( 'NONE', *, *, #18909, .T. ) ;
#6972=ORIENTED_EDGE ( 'NONE', *, *, #25716, .T. ) ;
#6973=CARTESIAN_POINT ( 'NONE',  ( 100.2919976486527247, 242.8371140006016162, 14.10862752716273150 ) ) ;
#6974=AXIS2_PLACEMENT_3D ( 'NONE', #25852, #19251, #1159 ) ;
#6976=EDGE_CURVE ( 'NONE', #5248, #18824, #27969, .T. ) ;
#6977=DIRECTION ( 'NONE',  ( 1.321694076934710155E-16, -1.000000000000000000, 0.000000000000000000 ) ) ;
#6984=DIRECTION ( 'NONE',  ( 1.000000000000000000, 1.153591111524576718E-14, 0.000000000000000000 ) ) ;
#6985=FACE_OUTER_BOUND ( 'NONE', #15560, .T. ) ;
#6988=PLANE ( 'NONE',  #19056 ) ;
#6991=DIRECTION ( 'NONE',  ( 1.000000000000000000, -0.000000000000000000, -0.000000000000000000 ) ) ;
#6994=DIRECTION ( 'NONE',  ( -0.000000000000000000, 0.000000000000000000, 1.000000000000000000 ) ) ;
#6999=VECTOR ( 'NONE', #7610, 1000.000000000000000 ) ;
#7002=CARTESIAN_POINT ( 'NONE',  ( -236.8177751472017007, 82.33896643611703325, -5.000000000000002665 ) ) ;
#7003=ORIENTED_EDGE ( 'NONE', *, *, #11073, .T. ) ;
#7006=ORIENTED_EDGE ( 'NONE', *, *, #19925, .F. ) ;
#7014=EDGE_CURVE ( 'NONE', #2828, #10760, #6023, .T. ) ;
#7015=EDGE_CURVE ( 'NONE', #24201, #16772, #27288, .T. ) ;
#7016=PLANE ( 'NONE',  #2264 ) ;
#7017=CARTESIAN_POINT ( 'NONE',  ( -33.73603230484052773, 129.3982133951581091, 15.58051746129034676 ) ) ;
#7019=CARTESIAN_POINT ( 'NONE',  ( -225.5243807178691213, 62.25611586199291025, 19.08347035850884410 ) ) ;
#7021=PLANE ( 'NONE',  #1187 ) ;
#7022=CIRCLE ( 'NONE', #11641, 60.90601976618767566 ) ;
#7032=CARTESIAN_POINT ( 'NONE',  ( -1.259556330921223433, 135.5648644267808436, 13.59427901309335596 ) ) ;
#7033=DIRECTION ( 'NONE',  ( -1.541976423090495387E-16, 1.000000000000000000, 0.000000000000000000 ) ) ;
#7038=CARTESIAN_POINT ( 'NONE',  ( -205.9966200546697905, 90.40127925949050791, -28.21257754844605969 ) ) ;
#7042=ORIENTED_EDGE ( 'NONE', *, *, #22159, .F. ) ;
#7043=VECTOR ( 'NONE', #19239, 1000.000000000000000 ) ;
#7045=AXIS2_PLACEMENT_3D ( 'NONE', #2056, #26460, #6655 ) ;
#7047=CARTESIAN_POINT ( 'NONE',  ( -155.6312558209752979, 121.5918491723093524, 21.28780381422281920 ) ) ;
#7049=AXIS2_PLACEMENT_3D ( 'NONE', #14285, #16160, #27609 ) ;
#7052=EDGE_CURVE ( 'NONE', #9545, #15146, #18676, .T. ) ;
#7056=CARTESIAN_POINT ( 'NONE',  ( 104.2819297219271562, 239.9331382545718441, -27.31288972538037996 ) ) ;
#7057=DIRECTION ( 'NONE',  ( -0.000000000000000000, 1.000000000000000000, -0.000000000000000000 ) ) ;
#7059=CARTESIAN_POINT ( 'NONE',  ( -213.7039558558103352, 55.82027786946292025, -42.47917487896670963 ) ) ;
#7061=ORIENTED_EDGE ( 'NONE', *, *, #24007, .T. ) ;
#7065=CARTESIAN_POINT ( 'NONE',  ( -224.3418196798764086, 136.6081117166938839, -14.97424725141357094 ) ) ;
#7066=FACE_OUTER_BOUND ( 'NONE', #21655, .T. ) ;
#7072=ORIENTED_EDGE ( 'NONE', *, *, #912, .T. ) ;
#7078=FACE_OUTER_BOUND ( 'NONE', #8252, .T. ) ;
#7081=VECTOR ( 'NONE', #20124, 1000.000000000000000 ) ;
#7083=DIRECTION ( 'NONE',  ( 0.000000000000000000, 0.000000000000000000, -1.000000000000000000 ) ) ;
#7087=VERTEX_POINT ( 'NONE', #6595 ) ;
#7092=CARTESIAN_POINT ( 'NONE',  ( -11.66034562843645439, 131.4488408685630247, -14.75304520776273876 ) ) ;
#7096=CARTESIAN_POINT ( 'NONE',  ( -40.40953891503691153, 0.000000000000000000, 99.00000000000000000 ) ) ;
#7103=ORIENTED_EDGE ( 'NONE', *, *, #13325, .F. ) ;
#7104=VECTOR ( 'NONE', #8898, 1000.000000000000000 ) ;
#7106=EDGE_LOOP ( 'NONE', ( #26139, #8434, #16830, #3855, #27548, #19177, #4502, #6048, #3037, #20566, #24793, #21013, #26534, #21517, #22899, #3060 ) ) ;
#7108=CARTESIAN_POINT ( 'NONE',  ( -218.0684950290402071, 60.60891383183041370, -12.02124378490089285 ) ) ;
#7109=CYLINDRICAL_SURFACE ( 'NONE', #16312, 16.07743405327025243 ) ;
#7112=DIRECTION ( 'NONE',  ( 0.000000000000000000, 0.000000000000000000, 1.000000000000000000 ) ) ;
#7113=VECTOR ( 'NONE', #24174, 1000.000000000000000 ) ;
#7114=VERTEX_POINT ( 'NONE', #19241 ) ;
#7115=CARTESIAN_POINT ( 'NONE',  ( -211.5723746692770817, 73.07838658328543602, 31.37812082757087495 ) ) ;
#7119=ADVANCED_FACE ( 'NONE', ( #25844 ), #13215, .T. ) ;
#7121=EDGE_CURVE ( 'NONE', #14063, #16893, #1848, .T. ) ;
#7126=VERTEX_POINT ( 'NONE', #15084 ) ;
#7127=ORIENTED_EDGE ( 'NONE', *, *, #149, .T. ) ;
#7128=CARTESIAN_POINT ( 'NONE',  ( 106.0806716804939356, 248.0923932631196749, 24.09863730004343552 ) ) ;
#7131=AXIS2_PLACEMENT_3D ( 'NONE', #15442, #25912, #15302 ) ;
#7134=CARTESIAN_POINT ( 'NONE',  ( 65.00000000000000000, -120.0250000000000909, -63.99999999999998579 ) ) ;
#7140=VERTEX_POINT ( 'NONE', #4296 ) ;
#7147=CIRCLE ( 'NONE', #12672, 11.00000000000001066 ) ;
#7148=CIRCLE ( 'NONE', #19078, 5.000000000000004441 ) ;
#7161=CARTESIAN_POINT ( 'NONE',  ( 65.00000000000000000, -120.0250000000000909, -69.99999999999998579 ) ) ;
#7167=FACE_OUTER_BOUND ( 'NONE', #22155, .T. ) ;
#7168=CARTESIAN_POINT ( 'NONE',  ( -228.8737713456696952, 63.73618850396876923, 17.32239903714441809 ) ) ;
#7171=CARTESIAN_POINT ( 'NONE',  ( 79.99999999999997158, 83.92694226569396676, -99.80661736361717828 ) ) ;
#7172=CARTESIAN_POINT ( 'NONE',  ( -206.8654573299152162, 90.47654849149037659, -26.13928083963914517 ) ) ;
#7173=( BOUNDED_SURFACE ( )  B_SPLINE_SURFACE ( 3, 2, ( 
 ( #19248, #25849, #23703 ),
 ( #19812, #28399, #6174 ),
 ( #17511, #27992, #26280 ),
 ( #14951, #4438, #21968 ),
 ( #4009, #12796, #1852 ),
 ( #15522, #2280, #8477 ),
 ( #11058, #3872, #17232 ),
 ( #25991, #6310, #15088 ),
 ( #2000, #9484, #23078 ),
 ( #1236, #20386, #10003 ),
 ( #5009, #18098, #572 ),
 ( #3384, #26853, #7322 ),
 ( #12173, #15949, #20916 ),
 ( #19958, #9336, #16475 ),
 ( #9192, #18760, #11649 ),
 ( #13801, #6884, #25226 ),
 ( #14320, #5545, #27509 ),
 ( #7842, #13364, #15663 ),
 ( #24269, #20097, #4578 ),
 ( #22256, #24557, #7032 ),
 ( #22547, #26989, #22113 ),
 ( #24703, #2421, #9045 ),
 ( #26554, #17798, #4722 ),
 ( #24411, #2858, #429 ) ),
 .UNSPECIFIED., .F., .F., .T. ) 
 B_SPLINE_SURFACE_WITH_KNOTS ( ( 4, 2, 2, 2, 2, 2, 2, 2, 2, 2, 2, 4 ),
 ( 3, 3 ),
 ( 0.000000000000000000, 0.006931781491214596483, 0.01386356298242919297, 0.01732945372803649381, 0.02079534447364379118, 0.02772712596485838593, 0.03465890745607298762, 0.03639185282887663631, 0.03812479820168028499, 0.04159068894728758237, 0.04852247043850217711, 0.05545425192971677186 ),
 ( 0.000000000000000000, 1.000000000000000000 ),
 .UNSPECIFIED. ) 
 GEOMETRIC_REPRESENTATION_ITEM ( )  RATIONAL_B_SPLINE_SURFACE ( (
 ( 1.000000000000000000, 0.8161343730438194166, 1.000000000000000000),
 ( 1.000000000000000000, 0.8224195403628062895, 1.000000000000000000),
 ( 1.000000000000000000, 0.8273233292672230732, 1.000000000000000000),
 ( 1.000000000000000000, 0.8342607332264897479, 1.000000000000000000),
 ( 1.000000000000000000, 0.8362950954338710385, 1.000000000000000000),
 ( 1.000000000000000000, 0.8371032263789185413, 1.000000000000000000),
 ( 1.000000000000000000, 0.8369960692425010285, 1.000000000000000000),
 ( 1.000000000000000000, 0.8360286494151781822, 1.000000000000000000),
 ( 1.000000000000000000, 0.8351716839152490968, 1.000000000000000000),
 ( 1.000000000000000000, 0.8315174131673371827, 1.000000000000000000),
 ( 1.000000000000000000, 0.8276373651588401215, 1.000000000000000000),
 ( 1.000000000000000000, 0.8171610397916245772, 1.000000000000000000),
 ( 1.000000000000000000, 0.8105635768882419878, 1.000000000000000000),
 ( 1.000000000000000000, 0.8007212358742062941, 1.000000000000000000),
 ( 1.000000000000000000, 0.7986706403516325992, 1.000000000000000000),
 ( 1.000000000000000000, 0.7944384422229460174, 1.000000000000000000),
 ( 1.000000000000000000, 0.7922545277786539053, 1.000000000000000000),
 ( 1.000000000000000000, 0.7855097680936570237, 1.000000000000000000),
 ( 1.000000000000000000, 0.7807558079320371380, 1.000000000000000000),
 ( 1.000000000000000000, 0.7658071389224905268, 1.000000000000000000),
 ( 1.000000000000000000, 0.7549214566164625939, 1.000000000000000000),
 ( 1.000000000000000000, 0.7318315617936779205, 1.000000000000000000),
 ( 1.000000000000000000, 0.7196266900043837289, 1.000000000000000000),
 ( 1.000000000000000000, 0.7071067811865477948, 1.000000000000000000) ) ) 
 REPRESENTATION_ITEM ( '' )  SURFACE ( )  );
#7174=AXIS2_PLACEMENT_3D ( 'NONE', #25813, #6141, #13465 ) ;
#7177=CARTESIAN_POINT ( 'NONE',  ( -200.0000000000000284, -120.0000000000001279, 25.00000000000000000 ) ) ;
#7180=CARTESIAN_POINT ( 'NONE',  ( -161.9363290404624820, 118.9535531856865163, 23.59303681828691879 ) ) ;
#7182=ORIENTED_EDGE ( 'NONE', *, *, #14822, .T. ) ;
#7183=ORIENTED_EDGE ( 'NONE', *, *, #24018, .F. ) ;
#7189=ORIENTED_EDGE ( 'NONE', *, *, #15983, .T. ) ;
#7191=ORIENTED_EDGE ( 'NONE', *, *, #14545, .T. ) ;
#7193=DIRECTION ( 'NONE',  ( 0.000000000000000000, 0.000000000000000000, -1.000000000000000000 ) ) ;
#7194=CARTESIAN_POINT ( 'NONE',  ( -133.8788553768147267, 130.0499255244862127, 16.66544065180372414 ) ) ;
#7196=ORIENTED_EDGE ( 'NONE', *, *, #17292, .F. ) ;
#7197=VECTOR ( 'NONE', #2960, 1000.000000000000000 ) ;
#7200=CARTESIAN_POINT ( 'NONE',  ( 179.9999999999999147, 330.0000000000000000, 100.0000000000000142 ) ) ;
#7205=DIRECTION ( 'NONE',  ( -1.000000000000000000, 0.000000000000000000, 0.000000000000000000 ) ) ;
#7206=FACE_OUTER_BOUND ( 'NONE', #17282, .T. ) ;
#7208=CARTESIAN_POINT ( 'NONE',  ( -213.4585383333369180, 57.78353604556345857, -35.98283585097398429 ) ) ;
#7209=CIRCLE ( 'NONE', #23264, 43.76444293738737912 ) ;
#7210=DIRECTION ( 'NONE',  ( 0.000000000000000000, 0.000000000000000000, -1.000000000000000000 ) ) ;
#7212=CARTESIAN_POINT ( 'NONE',  ( -227.3657730843038678, 133.9833936510422632, -14.99191580167116378 ) ) ;
#7218=CARTESIAN_POINT ( 'NONE',  ( -40.40953891503691153, 71.03850157808263077, 99.00000000000000000 ) ) ;
#7222=EDGE_LOOP ( 'NONE', ( #10644, #17277, #26749, #2333 ) ) ;
#7223=DIRECTION ( 'NONE',  ( 1.000000000000000000, -0.000000000000000000, -0.000000000000000000 ) ) ;
#7226=VERTEX_POINT ( 'NONE', #22369 ) ;
#7227=CIRCLE ( 'NONE', #19585, 2.000000000000007550 ) ;
#7230=AXIS2_PLACEMENT_3D ( 'NONE', #13783, #3256, #12049 ) ;
#7231=EDGE_CURVE ( 'NONE', #4081, #10866, #17913, .T. ) ;
#7235=ORIENTED_EDGE ( 'NONE', *, *, #13540, .T. ) ;
#7236=DIRECTION ( 'NONE',  ( -0.000000000000000000, -1.000000000000000000, -0.000000000000000000 ) ) ;
#7238=DIRECTION ( 'NONE',  ( 1.000000000000000000, -0.000000000000000000, -0.000000000000000000 ) ) ;
#7239=CARTESIAN_POINT ( 'NONE',  ( -13.66674585099290873, 130.9048851640479825, -16.37515642400365579 ) ) ;
#7244=ORIENTED_EDGE ( 'NONE', *, *, #11680, .T. ) ;
#7245=DIRECTION ( 'NONE',  ( 0.000000000000000000, 0.000000000000000000, 1.000000000000000000 ) ) ;
#7248=DIRECTION ( 'NONE',  ( 0.000000000000000000, 0.000000000000000000, 1.000000000000000000 ) ) ;
#7249=ORIENTED_EDGE ( 'NONE', *, *, #16464, .F. ) ;
#7251=AXIS2_PLACEMENT_3D ( 'NONE', #13853, #13040, #10733 ) ;
#7255=CYLINDRICAL_SURFACE ( 'NONE', #12846, 24.07986109634097005 ) ;
#7256=DIRECTION ( 'NONE',  ( 0.000000000000000000, -0.000000000000000000, -1.000000000000000000 ) ) ;
#7257=VERTEX_POINT ( 'NONE', #24105 ) ;
#7258=DIRECTION ( 'NONE',  ( -0.000000000000000000, -0.000000000000000000, 1.000000000000000000 ) ) ;
#7260=EDGE_LOOP ( 'NONE', ( #23470, #26147, #17464, #266, #21262, #16489 ) ) ;
#7263=CARTESIAN_POINT ( 'NONE',  ( -233.2943309833541718, 92.06151970357193193, -15.00000000000000000 ) ) ;
#7264=ORIENTED_EDGE ( 'NONE', *, *, #18057, .F. ) ;
#7269=ADVANCED_FACE ( 'NONE', ( #6848 ), #26516, .F. ) ;
#7279=DIRECTION ( 'NONE',  ( 1.000000000000000000, 0.000000000000000000, 0.000000000000000000 ) ) ;
#7281=FACE_OUTER_BOUND ( 'NONE', #11028, .T. ) ;
#7284=CYLINDRICAL_SURFACE ( 'NONE', #13711, 2.000000000000003109 ) ;
#7288=EDGE_CURVE ( 'NONE', #22168, #26591, #492, .T. ) ;
#7289=CIRCLE ( 'NONE', #10477, 80.00000000000000000 ) ;
#7297=VERTEX_POINT ( 'NONE', #28249 ) ;
#7300=VECTOR ( 'NONE', #16675, 1000.000000000000000 ) ;
#7304=DIRECTION ( 'NONE',  ( 0.000000000000000000, 0.000000000000000000, 1.000000000000000000 ) ) ;
#7308=CARTESIAN_POINT ( 'NONE',  ( -52.83157022077657672, 131.8429468099762687, -16.11955406963874537 ) ) ;
#7310=AXIS2_PLACEMENT_3D ( 'NONE', #14128, #7373, #24897 ) ;
#7311=CARTESIAN_POINT ( 'NONE',  ( -213.2358879321101313, 57.03087831670950436, 38.93822867433466683 ) ) ;
#7317=DIRECTION ( 'NONE',  ( 1.000000000000000000, 0.000000000000000000, 0.000000000000000000 ) ) ;
#7319=CARTESIAN_POINT ( 'NONE',  ( 84.91648909967247505, 110.3843228249417479, 70.37109374985131183 ) ) ;
#7320=ADVANCED_FACE ( 'NONE', ( #2247 ), #26245, .T. ) ;
#7322=CARTESIAN_POINT ( 'NONE',  ( -13.76547155678103707, 130.8815623877831911, 14.96787615611629541 ) ) ;
#7325=CARTESIAN_POINT ( 'NONE',  ( -191.5097071395943544, 102.0944051927142340, 32.85252593193306581 ) ) ;
#7327=ORIENTED_EDGE ( 'NONE', *, *, #12776, .F. ) ;
#7331=CARTESIAN_POINT ( 'NONE',  ( 33.10302365956999182, 203.2034914284457159, -13.00000000000000000 ) ) ;
#7334=AXIS2_PLACEMENT_3D ( 'NONE', #16256, #10058, #5180 ) ;
#7336=FACE_OUTER_BOUND ( 'NONE', #4599, .T. ) ;
#7339=ORIENTED_EDGE ( 'NONE', *, *, #15780, .T. ) ;
#7348=CARTESIAN_POINT ( 'NONE',  ( 91.02002523439647064, 230.3620959593083342, -17.09244139626534320 ) ) ;
#7352=DIRECTION ( 'NONE',  ( 0.000000000000000000, 0.000000000000000000, -1.000000000000000000 ) ) ;
#7353=CARTESIAN_POINT ( 'NONE',  ( -194.6040764069587112, 63.06822542404761123, -40.63350569893458442 ) ) ;
#7355=CARTESIAN_POINT ( 'NONE',  ( -279.3160071107327553, -91.18033988749901653, -14.13483123440684253 ) ) ;
#7358=DIRECTION ( 'NONE',  ( 1.321694076934710155E-16, -1.000000000000000000, 0.000000000000000000 ) ) ;
#7365=ORIENTED_EDGE ( 'NONE', *, *, #15435, .F. ) ;
#7366=AXIS2_PLACEMENT_3D ( 'NONE', #20833, #27704, #3864 ) ;
#7367=CARTESIAN_POINT ( 'NONE',  ( 105.2480867101079980, 123.6573351780392613, 85.93750000029402258 ) ) ;
#7368=CARTESIAN_POINT ( 'NONE',  ( -203.2481855153402250, 92.57460631283319685, -29.78692811926998729 ) ) ;
#7373=DIRECTION ( 'NONE',  ( 1.000000000000000000, -0.000000000000000000, -0.000000000000000000 ) ) ;
#7378=EDGE_CURVE ( 'NONE', #11333, #28119, #26173, .T. ) ;
#7380=AXIS2_PLACEMENT_3D ( 'NONE', #20907, #16193, #14042 ) ;
#7381=ADVANCED_FACE ( 'NONE', ( #19003 ), #23033, .F. ) ;
#7382=CARTESIAN_POINT ( 'NONE',  ( 139.9999999999999432, -90.00000000000000000, -100.0000000000000142 ) ) ;
#7384=CARTESIAN_POINT ( 'NONE',  ( -28.21136509376883694, 127.9579735385673018, -17.52291426357238535 ) ) ;
#7385=DIRECTION ( 'NONE',  ( 0.000000000000000000, 0.000000000000000000, 1.000000000000000000 ) ) ;
#7389=ORIENTED_EDGE ( 'NONE', *, *, #20600, .T. ) ;
#7394=CARTESIAN_POINT ( 'NONE',  ( 119.9999999999998863, 330.0000000000000000, 100.0000000000000142 ) ) ;
#7399=CARTESIAN_POINT ( 'NONE',  ( -229.6839157287631394, 64.28192771017235430, -7.255073467994252567 ) ) ;
#7408=ORIENTED_EDGE ( 'NONE', *, *, #6093, .T. ) ;
#7409=ORIENTED_EDGE ( 'NONE', *, *, #5486, .T. ) ;
#7411=ORIENTED_EDGE ( 'NONE', *, *, #28294, .F. ) ;
#7414=ORIENTED_EDGE ( 'NONE', *, *, #20317, .F. ) ;
#7415=CARTESIAN_POINT ( 'NONE',  ( 109.9639884628863058, 258.5863491988774854, 43.28603914701826483 ) ) ;
#7416=EDGE_CURVE ( 'NONE', #24468, #8776, #16549, .T. ) ;
#7420=DIRECTION ( 'NONE',  ( -0.000000000000000000, -0.000000000000000000, 1.000000000000000000 ) ) ;
#7421=DIRECTION ( 'NONE',  ( 1.000000000000000000, 0.000000000000000000, 0.000000000000000000 ) ) ;
#7424=FACE_OUTER_BOUND ( 'NONE', #17376, .T. ) ;
#7425=DIRECTION ( 'NONE',  ( -0.000000000000000000, 1.000000000000000000, -1.387778780781445429E-16 ) ) ;
#7426=CARTESIAN_POINT ( 'NONE',  ( 109.9999999999998863, 330.0000000000000000, -90.00000000000004263 ) ) ;
#7428=STYLED_ITEM('',(#28455),#28156);
#7429=EDGE_LOOP ( 'NONE', ( #8226, #18882, #23369, #15894 ) ) ;
#7430=AXIS2_PLACEMENT_3D ( 'NONE', #27513, #688, #9730 ) ;
#7432=EDGE_CURVE ( 'NONE', #7126, #10815, #20877, .T. ) ;
#7433=CARTESIAN_POINT ( 'NONE',  ( -237.3870311360068683, 121.7710280244218524, -13.00000000000000000 ) ) ;
#7434=CARTESIAN_POINT ( 'NONE',  ( -189.5231184314577604, 157.6231267382823376, 12.99999999999999822 ) ) ;
#7443=AXIS2_PLACEMENT_3D ( 'NONE', #17164, #8122, #15020 ) ;
#7444=VERTEX_POINT ( 'NONE', #9962 ) ;
#7446=ORIENTED_EDGE ( 'NONE', *, *, #21180, .F. ) ;
#7449=DIRECTION ( 'NONE',  ( 1.000000000000000000, 0.000000000000000000, 0.000000000000000000 ) ) ;
#7450=FACE_OUTER_BOUND ( 'NONE', #18532, .T. ) ;
#7452=CARTESIAN_POINT ( 'NONE',  ( -82.62938906138147388, 134.8301624926916986, -15.44879298257729161 ) ) ;
#7456=CARTESIAN_POINT ( 'NONE',  ( -209.5875676835875083, 74.18578632021306873, 35.35260769160358052 ) ) ;
#7458=CARTESIAN_POINT ( 'NONE',  ( -148.2538183076392215, 125.4301416103809288, -17.54546909480966121 ) ) ;
#7459=CARTESIAN_POINT ( 'NONE',  ( 79.99999999999997158, 99.82480251742194355, -92.60160435377096633 ) ) ;
#7461=CARTESIAN_POINT ( 'NONE',  ( 179.9999999999999147, -150.0000000000000284, 100.0000000000000142 ) ) ;
#7466=AXIS2_PLACEMENT_3D ( 'NONE', #18270, #7358, #27023 ) ;
#7468=CARTESIAN_POINT ( 'NONE',  ( 116.3389527600916722, 113.0483370489294686, -100.0000000000000142 ) ) ;
#7470=DIRECTION ( 'NONE',  ( 0.000000000000000000, 0.000000000000000000, -1.000000000000000000 ) ) ;
#7472=ORIENTED_EDGE ( 'NONE', *, *, #4234, .T. ) ;
#7475=LINE ( 'NONE', #20818, #5609 ) ;
#7478=PLANE ( 'NONE',  #576 ) ;
#7479=CARTESIAN_POINT ( 'NONE',  ( -81.45374247556539160, 136.3900883041769134, 15.17089325038065795 ) ) ;
#7485=CARTESIAN_POINT ( 'NONE',  ( 109.9999999999999289, -70.00000000000001421, 70.00000000000001421 ) ) ;
#7495=CARTESIAN_POINT ( 'NONE',  ( -218.5620487852755218, 71.28382977987342883, -22.94473774457503978 ) ) ;
#7500=EDGE_LOOP ( 'NONE', ( #13699, #7828, #20749, #1184 ) ) ;
#7501=VECTOR ( 'NONE', #26050, 1000.000000000000000 ) ;
#7506=ORIENTED_EDGE ( 'NONE', *, *, #13099, .T. ) ;
#7510=CARTESIAN_POINT ( 'NONE',  ( 109.5756401947595862, 134.3783162857569664, 100.0000000000216573 ) ) ;
#7513=ADVANCED_FACE ( 'NONE', ( #23177 ), #5121, .T. ) ;
#7514=VERTEX_POINT ( 'NONE', #10950 ) ;
#7522=CARTESIAN_POINT ( 'NONE',  ( 79.99999999999994316, 80.00000000000001421, 100.0000000000000142 ) ) ;
#7523=ORIENTED_EDGE ( 'NONE', *, *, #17446, .T. ) ;
#7528=DIRECTION ( 'NONE',  ( -0.4767408570798813972, 0.8790438869537404720, 0.000000000000000000 ) ) ;
#7529=CARTESIAN_POINT ( 'NONE',  ( -7.291805129867194424, 132.9340346030435001, -15.80620534190248527 ) ) ;
#7532=DIRECTION ( 'NONE',  ( 1.000000000000000000, 0.000000000000000000, 0.000000000000000000 ) ) ;
#7534=VERTEX_POINT ( 'NONE', #21726 ) ;
#7535=CARTESIAN_POINT ( 'NONE',  ( 65.00000000000000000, -150.0000000000000568, -75.99999999999998579 ) ) ;
#7548=TOROIDAL_SURFACE ( 'NONE', #26793, 21.49999999999998224, 1.000000000000000000 ) ;
#7551=DIRECTION ( 'NONE',  ( 0.000000000000000000, 0.000000000000000000, 1.000000000000000000 ) ) ;
#7552=CARTESIAN_POINT ( 'NONE',  ( 102.7211906516483424, 244.5533218984080293, 17.51413272308122160 ) ) ;
#7554=VECTOR ( 'NONE', #6494, 1000.000000000000000 ) ;
#7562=B_SPLINE_CURVE_WITH_KNOTS ( 'NONE', 3,
 ( #15911, #675, #22791, #23069, #811, #16465, #14173, #3374, #1227, #5395, #12018, #3090, #20343, #9440, #5256, #947, #14310, #18340, #22926, #20764, #26950, #16332 ),
 .UNSPECIFIED., .F., .F.,
 ( 4, 2, 2, 2, 2, 2, 2, 2, 2, 2, 4 ),
 ( 0.000000000000000000, 0.06250000000000000000, 0.1250000000000000000, 0.1875000000000000000, 0.2500000000000000000, 0.3750000000000000000, 0.5000000000000000000, 0.6250000000000000000, 0.7500000000000000000, 0.8750000000000001110, 1.000000000000000000 ),
 .UNSPECIFIED. ) ;
#7563=CARTESIAN_POINT ( 'NONE',  ( 109.9999999999999005, 260.0000000000000000, 45.00000000000000000 ) ) ;
#7564=DIRECTION ( 'NONE',  ( 1.000000000000000000, 0.000000000000000000, 0.000000000000000000 ) ) ;
#7567=CARTESIAN_POINT ( 'NONE',  ( -221.3650667873343139, -91.18033988749901653, 19.29759039828519818 ) ) ;
#7570=LINE ( 'NONE', #9858, #10865 ) ;
#7574=CARTESIAN_POINT ( 'NONE',  ( 0.000000000000000000, 330.0000000000000000, 100.0000000000000142 ) ) ;
#7576=CARTESIAN_POINT ( 'NONE',  ( 99.17397288323584803, 242.2128526578931371, -12.79873440004189966 ) ) ;
#7577=CARTESIAN_POINT ( 'NONE',  ( 23.19384040928324708, 86.94809229719507471, 99.18534753508888002 ) ) ;
#7580=EDGE_CURVE ( 'NONE', #5346, #19329, #6066, .T. ) ;
#7581=DIRECTION ( 'NONE',  ( 1.000000000000000000, 0.000000000000000000, 0.000000000000000000 ) ) ;
#7582=EDGE_LOOP ( 'NONE', ( #26944, #13920, #19726, #2572, #22514, #27301 ) ) ;
#7583=CIRCLE ( 'NONE', #23623, 30.00000000000000000 ) ;
#7585=VECTOR ( 'NONE', #10205, 1000.000000000000000 ) ;
#7586=ORIENTED_EDGE ( 'NONE', *, *, #2428, .T. ) ;
#7587=EDGE_LOOP ( 'NONE', ( #27520, #2778, #27653, #10159, #21037, #14648 ) ) ;
#7588=VERTEX_POINT ( 'NONE', #8515 ) ;
#7589=AXIS2_PLACEMENT_3D ( 'NONE', #12281, #24919, #22903 ) ;
#7591=CARTESIAN_POINT ( 'NONE',  ( -142.4951090877017634, 127.4563655094269023, 16.43271896145171240 ) ) ;
#7592=CARTESIAN_POINT ( 'NONE',  ( -230.8916957670046486, 130.8330661503598833, 15.00000000000000000 ) ) ;
#7596=CARTESIAN_POINT ( 'NONE',  ( -11.61564047653929599, 131.4612359469146838, 14.74843121655267275 ) ) ;
#7604=CARTESIAN_POINT ( 'NONE',  ( 156.4999999999998579, 220.0000000000000284, -100.0000000000000142 ) ) ;
#7609=CARTESIAN_POINT ( 'NONE',  ( 79.99999999999991473, 80.00000000000001421, -100.0000000000000142 ) ) ;
#7610=DIRECTION ( 'NONE',  ( 0.000000000000000000, 0.000000000000000000, -1.000000000000000000 ) ) ;
#7612=VERTEX_POINT ( 'NONE', #25887 ) ;
#7616=ORIENTED_EDGE ( 'NONE', *, *, #25278, .T. ) ;
#7625=EDGE_CURVE ( 'NONE', #12468, #2948, #11050, .T. ) ;
#7628=CARTESIAN_POINT ( 'NONE',  ( -123.8208147886770121, 198.8605305197760913, -15.00000000000000000 ) ) ;
#7631=CARTESIAN_POINT ( 'NONE',  ( 134.9999999999998579, 268.4896896257338881, 84.99999999999995737 ) ) ;
#7634=CARTESIAN_POINT ( 'NONE',  ( -279.3160071107327553, -83.68033988749907337, 0.000000000000000000 ) ) ;
#7635=FACE_BOUND ( 'NONE', #12245, .T. ) ;
#7636=DIRECTION ( 'NONE',  ( 0.000000000000000000, 0.000000000000000000, 1.000000000000000000 ) ) ;
#7637=VERTEX_POINT ( 'NONE', #15127 ) ;
#7639=EDGE_CURVE ( 'NONE', #27397, #19273, #15551, .T. ) ;
#7642=CARTESIAN_POINT ( 'NONE',  ( -240.4233474261503716, 71.57180907113834678, 14.67903078147715235 ) ) ;
#7646=EDGE_CURVE ( 'NONE', #7612, #7786, #26645, .T. ) ;
#7647=VECTOR ( 'NONE', #16335, 1000.000000000000000 ) ;
#7656=ORIENTED_EDGE ( 'NONE', *, *, #14413, .T. ) ;
#7658=DIRECTION ( 'NONE',  ( 1.000000000000000000, 0.000000000000000000, 0.000000000000000000 ) ) ;
#7659=VERTEX_POINT ( 'NONE', #17835 ) ;
#7661=DIRECTION ( 'NONE',  ( 1.321694076934710155E-16, -1.000000000000000000, 0.000000000000000000 ) ) ;
#7667=CARTESIAN_POINT ( 'NONE',  ( 109.9999999999999289, 110.0000000000000142, -45.00000000000000000 ) ) ;
#7674=CARTESIAN_POINT ( 'NONE',  ( -236.3091765109048197, 68.24607436519742976, 5.736201002603997345 ) ) ;
#7680=VERTEX_POINT ( 'NONE', #26738 ) ;
#7681=CARTESIAN_POINT ( 'NONE',  ( -160.0000000000000284, 59.99999999999994316, 45.00000000000000000 ) ) ;
#7686=DIRECTION ( 'NONE',  ( 1.541976423090495387E-16, -1.000000000000000000, 0.000000000000000000 ) ) ;
#7691=VERTEX_POINT ( 'NONE', #11385 ) ;
#7693=ORIENTED_EDGE ( 'NONE', *, *, #11001, .T. ) ;
#7695=CARTESIAN_POINT ( 'NONE',  ( 109.8079904625031276, 257.1776683528518106, 40.10892953524286497 ) ) ;
#7698=CARTESIAN_POINT ( 'NONE',  ( -215.4886702565632106, 139.8420026707766226, 12.99999999999999822 ) ) ;
#7704=DIRECTION ( 'NONE',  ( 1.000000000000000000, 0.000000000000000000, 0.000000000000000000 ) ) ;
#7710=ADVANCED_FACE ( 'NONE', ( #16124 ), #21853, .T. ) ;
#7714=CARTESIAN_POINT ( 'NONE',  ( -221.3650667873343139, -91.18033988749901653, -19.29759039828519818 ) ) ;
#7717=DIRECTION ( 'NONE',  ( -0.000000000000000000, -0.000000000000000000, -1.000000000000000000 ) ) ;
#7727=DIRECTION ( 'NONE',  ( 1.000000000000000000, 0.000000000000000000, 0.000000000000000000 ) ) ;
#7729=CIRCLE ( 'NONE', #14220, 19.07743405327024888 ) ;
#7730=CARTESIAN_POINT ( 'NONE',  ( -92.67942046851547389, 134.7159439475681779, -15.46877993217822400 ) ) ;
#7732=CARTESIAN_POINT ( 'NONE',  ( -180.0000000000000284, -50.00000000000004263, 110.0000000000000284 ) ) ;
#7734=CARTESIAN_POINT ( 'NONE',  ( -160.8326600028555902, 120.2355194873575073, -21.37420696376537776 ) ) ;
#7736=AXIS2_PLACEMENT_3D ( 'NONE', #18929, #5850, #14622 ) ;
#7739=LINE ( 'NONE', #9760, #11847 ) ;
#7740=DIRECTION ( 'NONE',  ( 0.000000000000000000, -1.000000000000000000, -0.000000000000000000 ) ) ;
#7743=CARTESIAN_POINT ( 'NONE',  ( -201.8712871270307971, 91.53752412319902021, -28.77272332722132120 ) ) ;
#7747=ORIENTED_EDGE ( 'NONE', *, *, #14984, .F. ) ;
#7748=EDGE_CURVE ( 'NONE', #7612, #1333, #27122, .T. ) ;
#7749=AXIS2_PLACEMENT_3D ( 'NONE', #10489, #4302, #28276 ) ;
#7751=ORIENTED_EDGE ( 'NONE', *, *, #18188, .T. ) ;
#7754=AXIS2_PLACEMENT_3D ( 'NONE', #18821, #14524, #1716 ) ;
#7763=CARTESIAN_POINT ( 'NONE',  ( 109.9696209020443973, 258.3904084527665077, -43.60594690666008688 ) ) ;
#7766=AXIS2_PLACEMENT_3D ( 'NONE', #6533, #4646, #15739 ) ;
#7769=CARTESIAN_POINT ( 'NONE',  ( -207.4994891700685002, 75.60264349980251097, -44.78213549412046746 ) ) ;
#7771=CARTESIAN_POINT ( 'NONE',  ( -189.5231184314577604, 157.6231267382823091, 15.00000000000000000 ) ) ;
#7772=CARTESIAN_POINT ( 'NONE',  ( -270.1025481742786951, -91.18033988749901653, -14.95564396479129243 ) ) ;
#7773=FACE_OUTER_BOUND ( 'NONE', #13844, .T. ) ;
#7776=ADVANCED_FACE ( 'NONE', ( #10212 ), #25289, .T. ) ;
#7779=VERTEX_POINT ( 'NONE', #3163 ) ;
#7783=AXIS2_PLACEMENT_3D ( 'NONE', #23948, #15048, #26230 ) ;
#7786=VERTEX_POINT ( 'NONE', #23281 ) ;
#7787=EDGE_CURVE ( 'NONE', #19329, #21631, #24376, .T. ) ;
#7788=CARTESIAN_POINT ( 'NONE',  ( 87.74278500246884960, 111.0010834413659921, -71.13281249983540988 ) ) ;
#7789=AXIS2_PLACEMENT_3D ( 'NONE', #7433, #20358, #11895 ) ;
#7790=EDGE_CURVE ( 'NONE', #6688, #19256, #16539, .T. ) ;
#7791=CARTESIAN_POINT ( 'NONE',  ( 107.9379653822511216, 247.3366651132932077, 33.97036151511563418 ) ) ;
#7792=DIRECTION ( 'NONE',  ( -0.000000000000000000, -0.000000000000000000, 1.000000000000000000 ) ) ;
#7794=CARTESIAN_POINT ( 'NONE',  ( -229.4141265690028604, 89.10432210626537142, 15.37309836091423954 ) ) ;
#7795=ORIENTED_EDGE ( 'NONE', *, *, #12508, .F. ) ;
#7796=DIRECTION ( 'NONE',  ( 1.000000000000000000, 1.321694076934710155E-16, 0.000000000000000000 ) ) ;
#7798=ADVANCED_FACE ( 'NONE', ( #25431 ), #1435, .F. ) ;
#7802=DIRECTION ( 'NONE',  ( -0.000000000000000000, 0.000000000000000000, 1.000000000000000000 ) ) ;
#7803=CARTESIAN_POINT ( 'NONE',  ( -183.1437745737416947, 107.7727709130676743, -31.77045322972226060 ) ) ;
#7804=ORIENTED_EDGE ( 'NONE', *, *, #5878, .F. ) ;
#7809=CARTESIAN_POINT ( 'NONE',  ( -12.24491960465745599, 75.97823757117562593, 100.0000000000000000 ) ) ;
#7811=DIRECTION ( 'NONE',  ( 0.000000000000000000, 1.000000000000000000, 0.000000000000000000 ) ) ;
#7819=DIRECTION ( 'NONE',  ( -1.000000000000000000, -2.602085213965211135E-16, 0.000000000000000000 ) ) ;
#7828=ORIENTED_EDGE ( 'NONE', *, *, #24259, .T. ) ;
#7830=CARTESIAN_POINT ( 'NONE',  ( 109.7839892703147058, 255.7665025292604071, 41.33169715143176859 ) ) ;
#7834=DIRECTION ( 'NONE',  ( 0.000000000000000000, 0.000000000000000000, -1.000000000000000000 ) ) ;
#7836=CARTESIAN_POINT ( 'NONE',  ( 65.00000000000000000, -150.0000000000000568, -69.99999999999998579 ) ) ;
#7840=DIRECTION ( 'NONE',  ( -0.000000000000000000, -0.000000000000000000, 1.000000000000000000 ) ) ;
#7842=CARTESIAN_POINT ( 'NONE',  ( -4.528689226187404770, 132.3876760956092085, 15.97891348274549372 ) ) ;
#7843=VECTOR ( 'NONE', #27880, 1000.000000000000000 ) ;
#7844=CARTESIAN_POINT ( 'NONE',  ( 107.4212424090118532, 250.1602674884502164, -27.81180689761807301 ) ) ;
#7845=CARTESIAN_POINT ( 'NONE',  ( 24.13113629555251549, 86.46862463748914251, 99.29534762745656451 ) ) ;
#7847=DIRECTION ( 'NONE',  ( 1.000000000000000000, -0.000000000000000000, -0.000000000000000000 ) ) ;
#7852=EDGE_CURVE ( 'NONE', #17982, #11545, #17033, .T. ) ;
#7854=VERTEX_POINT ( 'NONE', #7634 ) ;
#7859=DIRECTION ( 'NONE',  ( 0.000000000000000000, 0.000000000000000000, 1.000000000000000000 ) ) ;
#7860=CARTESIAN_POINT ( 'NONE',  ( -17.24491960465746132, 80.97823757117562593, 100.0000000000000000 ) ) ;
#7869=CARTESIAN_POINT ( 'NONE',  ( -194.3369914945607491, 63.17511408073718826, 42.65718952139617670 ) ) ;
#7871=CARTESIAN_POINT ( 'NONE',  ( 9.999999999999738876, -50.00000000000004263, 98.28427124746191623 ) ) ;
#7873=CARTESIAN_POINT ( 'NONE',  ( -204.3469586999375736, 91.62841992397034119, 29.24611696590164556 ) ) ;
#7884=EDGE_LOOP ( 'NONE', ( #20530, #118, #1309, #23904 ) ) ;
#7897=CARTESIAN_POINT ( 'NONE',  ( 109.9924055441390891, 259.1950347634139575, -44.30286641876279674 ) ) ;
#7904=CARTESIAN_POINT ( 'NONE',  ( -254.3350114625770289, -91.18033988749901653, -16.36034929305424512 ) ) ;
#7907=DIRECTION ( 'NONE',  ( 1.000000000000000000, 0.000000000000000000, 0.000000000000000000 ) ) ;
#7911=FACE_OUTER_BOUND ( 'NONE', #21672, .T. ) ;
#7915=ORIENTED_EDGE ( 'NONE', *, *, #4995, .F. ) ;
#7919=AXIS2_PLACEMENT_3D ( 'NONE', #17235, #3, #292 ) ;
#7924=ORIENTED_EDGE ( 'NONE', *, *, #1014, .T. ) ;
#7931=VERTEX_POINT ( 'NONE', #27852 ) ;
#7937=CARTESIAN_POINT ( 'NONE',  ( -42.65532241761712839, 131.0044336801082352, -16.34779397420837199 ) ) ;
#7938=CARTESIAN_POINT ( 'NONE',  ( 139.9999999999999716, -120.0000000000000568, -70.00000000000001421 ) ) ;
#7939=AXIS2_PLACEMENT_3D ( 'NONE', #3651, #19027, #27635 ) ;
#7940=DIRECTION ( 'NONE',  ( 1.000000000000000000, 0.000000000000000000, 0.000000000000000000 ) ) ;
#7941=CARTESIAN_POINT ( 'NONE',  ( -202.4538189947720923, 93.28718049315023109, -30.13672334157483235 ) ) ;
#7943=AXIS2_PLACEMENT_3D ( 'NONE', #20464, #3352, #5231 ) ;
#7948=DIRECTION ( 'NONE',  ( -0.000000000000000000, -0.000000000000000000, 1.000000000000000000 ) ) ;
#7951=DIRECTION ( 'NONE',  ( -0.000000000000000000, -0.000000000000000000, 1.000000000000000000 ) ) ;
#7955=CARTESIAN_POINT ( 'NONE',  ( -143.6428522700808230, 20.24192588826928585, 83.00000000000001421 ) ) ;
#7964=TOROIDAL_SURFACE ( 'NONE', #14388, 14.95564396479129243, 3.532530335305412716 ) ;
#7969=ORIENTED_EDGE ( 'NONE', *, *, #25021, .F. ) ;
#7971=AXIS2_PLACEMENT_3D ( 'NONE', #14459, #3521, #5402 ) ;
#7978=DIRECTION ( 'NONE',  ( 0.000000000000000000, 0.000000000000000000, -1.000000000000000000 ) ) ;
#7979=CARTESIAN_POINT ( 'NONE',  ( -224.3698807949888305, 62.17069777283708021, -9.096889663472497389 ) ) ;
#7980=DIRECTION ( 'NONE',  ( 0.2845658198851049314, -0.9586565047779721516, 0.000000000000000000 ) ) ;
#7983=DIRECTION ( 'NONE',  ( 0.000000000000000000, 0.000000000000000000, 1.000000000000000000 ) ) ;
#7985=CONICAL_SURFACE ( 'NONE', #18990, 6.025000000000002132, 0.7853981633974482790 ) ;
#7986=EDGE_CURVE ( 'NONE', #223, #4097, #10602, .T. ) ;
#7988=CARTESIAN_POINT ( 'NONE',  ( 97.40121527157118919, 241.4156563175464782, -11.01273568327458996 ) ) ;
#7992=CIRCLE ( 'NONE', #27698, 2.000000000000003109 ) ;
#8000=EDGE_CURVE ( 'NONE', #18031, #17928, #23417, .T. ) ;
#8002=CARTESIAN_POINT ( 'NONE',  ( -85.27280602623865491, 136.4561170694882435, 13.48388367063513371 ) ) ;
#8003=APPLICATION_CONTEXT ( 'automotive_design' ) ;
#8005=ORIENTED_EDGE ( 'NONE', *, *, #26997, .T. ) ;
#8009=FACE_OUTER_BOUND ( 'NONE', #21384, .T. ) ;
#8015=CARTESIAN_POINT ( 'NONE',  ( -222.7951581118867068, 86.58804311865961267, 17.41104556328208375 ) ) ;
#8022=EDGE_CURVE ( 'NONE', #11217, #7779, #8335, .T. ) ;
#8028=EDGE_CURVE ( 'NONE', #11012, #22407, #18855, .T. ) ;
#8029=ORIENTED_EDGE ( 'NONE', *, *, #24293, .T. ) ;
#8032=ORIENTED_EDGE ( 'NONE', *, *, #15983, .F. ) ;
#8034=ORIENTED_EDGE ( 'NONE', *, *, #24237, .T. ) ;
#8037=DIRECTION ( 'NONE',  ( 1.000000000000000000, 4.163336342344337027E-16, 0.000000000000000000 ) ) ;
#8041=CARTESIAN_POINT ( 'NONE',  ( 109.9999999999999005, 260.0000000000000000, -45.00000000000000000 ) ) ;
#8042=CARTESIAN_POINT ( 'NONE',  ( -23.68004821426667661, 128.1049817043144117, -17.45875844069260907 ) ) ;
#8043=CARTESIAN_POINT ( 'NONE',  ( 79.99999999999991473, 140.0000000000000000, 45.00000000000000000 ) ) ;
#8044=CIRCLE ( 'NONE', #4842, 11.42311362948588105 ) ;
#8045=DIRECTION ( 'NONE',  ( 0.000000000000000000, -0.000000000000000000, -1.000000000000000000 ) ) ;
#8046=CARTESIAN_POINT ( 'NONE',  ( -207.6005680426152082, 75.52797596137341429, -42.89671038906845979 ) ) ;
#8054=EDGE_CURVE ( 'NONE', #20648, #7226, #24836, .T. ) ;
#8058=B_SPLINE_CURVE_WITH_KNOTS ( 'NONE', 3,
 ( #7698, #16461, #15909, #4960, #13751, #2808, #25496, #12302, #10275 ),
 .UNSPECIFIED., .F., .F.,
 ( 4, 2, 1, 2, 4 ),
 ( 0.000000000000000000, 0.003850132855190869542, 0.007700265710381739084, 0.01155039856557260949, 0.01540053142076347817 ),
 .UNSPECIFIED. ) ;
#8061=VECTOR ( 'NONE', #24479, 1000.000000000000000 ) ;
#8067=VECTOR ( 'NONE', #19917, 1000.000000000000000 ) ;
#8068=ORIENTED_EDGE ( 'NONE', *, *, #1946, .F. ) ;
#8073=CARTESIAN_POINT ( 'NONE',  ( 104.4199312700443016, 89.58810137558876363, 100.0000000000000142 ) ) ;
#8074=ORIENTED_EDGE ( 'NONE', *, *, #13050, .F. ) ;
#8076=DIRECTION ( 'NONE',  ( 0.000000000000000000, 0.000000000000000000, -1.000000000000000000 ) ) ;
#8077=EDGE_CURVE ( 'NONE', #1913, #15391, #24413, .T. ) ;
#8078=CARTESIAN_POINT ( 'NONE',  ( -40.35434868956970433, 130.4209029819868704, -15.14570054738094562 ) ) ;
#8079=DIRECTION ( 'NONE',  ( 4.163336342344337027E-16, -1.000000000000000000, 1.387778780781445429E-16 ) ) ;
#8082=CARTESIAN_POINT ( 'NONE',  ( -191.3943905361025770, 102.1783726111194852, -32.85579694620437863 ) ) ;
#8086=( BOUNDED_SURFACE ( )  B_SPLINE_SURFACE ( 3, 2, ( 
 ( #25773, #4223, #14733 ),
 ( #14882, #19458, #21328 ),
 ( #21609, #23486, #4080 ),
 ( #3803, #21466, #6101 ),
 ( #12867, #21760, #23631 ),
 ( #1647, #15163, #10559 ),
 ( #1780, #1510, #28059 ),
 ( #27784, #12589, #8405 ),
 ( #25918, #23914, #17160 ),
 ( #2066, #6242, #19035 ),
 ( #26058, #8264, #3941 ),
 ( #13014, #15017, #10704 ),
 ( #14591, #25634, #10417 ),
 ( #10842, #12727, #23347 ),
 ( #19600, #23768, #7979 ),
 ( #6381, #1921, #28202 ),
 ( #8121, #19171, #16747 ),
 ( #8549, #17297, #16881 ),
 ( #25501, #5817, #3658 ),
 ( #12446, #21185, #27916 ),
 ( #17017, #5327, #27158 ),
 ( #3160, #22287, #459 ),
 ( #7495, #22854, #24442 ),
 ( #11950, #319, #5186 ),
 ( #11533, #20126, #20552 ),
 ( #9368, #20273, #2598 ),
 ( #13973, #20414, #16260 ),
 ( #605, #22579, #22721 ),
 ( #9073, #4752, #26735 ),
 ( #13828, #13537, #3024 ),
 ( #18126, #11812, #14104 ),
 ( #17831, #2741, #9218 ),
 ( #26884, #7208, #877 ),
 ( #24586, #9648, #6912 ),
 ( #18405, #2889, #11382 ),
 ( #22431, #15981, #15692 ),
 ( #17980, #25012, #26584 ),
 ( #13684, #7059, #15843 ),
 ( #24732, #4894, #11678 ),
 ( #5040, #742, #9511 ),
 ( #18266, #27017, #7353 ),
 ( #16121, #24872, #25705 ),
 ( #16951, #27426, #1294 ),
 ( #3722, #5608, #16399 ),
 ( #7769, #16812, #20973 ),
 ( #5746, #18819, #23278 ) ),
 .UNSPECIFIED., .F., .F., .F. ) 
 B_SPLINE_SURFACE_WITH_KNOTS ( ( 4, 2, 2, 2, 2, 2, 2, 2, 2, 2, 2, 2, 2, 2, 2, 2, 2, 2, 2, 2, 2, 2, 4 ),
 ( 3, 3 ),
 ( -1.040834085586084257E-17, 0.004062158184156347031, 0.008124316368312704470, 0.01015539546039088276, 0.01218647455246906278, 0.01624863273662541935, 0.01827971182870359590, 0.02031079092078177592, 0.02437294910493813249, 0.02640402819701630904, 0.02843510728909448906, 0.03249726547325084564, 0.03655942365740720568, 0.03859050274948538223, 0.04062158184156355878, 0.04468374002571991882, 0.04874589820987627886, 0.05280805639403263196, 0.05687021457818899201, 0.05890129367026716856, 0.06093237276234535205, 0.06296345185442353554, 0.06499453094650170515 ),
 ( 0.000000000000000000, 1.000000000000000000 ),
 .UNSPECIFIED. ) 
 GEOMETRIC_REPRESENTATION_ITEM ( )  RATIONAL_B_SPLINE_SURFACE ( (
 ( 1.000000000000000000, 0.7071067811865475727, 1.000000000000000000),
 ( 1.000000000000000000, 0.7127618277282021797, 1.000000000000000000),
 ( 1.000000000000000000, 0.7177019917273029792, 1.000000000000000000),
 ( 1.000000000000000000, 0.7259809929037955856, 1.000000000000000000),
 ( 1.000000000000000000, 0.7293222386929405499, 1.000000000000000000),
 ( 1.000000000000000000, 0.7329411530155929277, 1.000000000000000000),
 ( 1.000000000000000000, 0.7339161091547367066, 1.000000000000000000),
 ( 1.000000000000000000, 0.7353380047207777048, 1.000000000000000000),
 ( 1.000000000000000000, 0.7357895841719410690, 1.000000000000000000),
 ( 1.000000000000000000, 0.7363489957920964502, 1.000000000000000000),
 ( 1.000000000000000000, 0.7356640979630035826, 1.000000000000000000),
 ( 1.000000000000000000, 0.7329334158298154156, 1.000000000000000000),
 ( 1.000000000000000000, 0.7317386460501513756, 1.000000000000000000),
 ( 1.000000000000000000, 0.7287527534628306380, 1.000000000000000000),
 ( 1.000000000000000000, 0.7269678409233529814, 1.000000000000000000),
 ( 1.000000000000000000, 0.7207930214947959602, 1.000000000000000000),
 ( 1.000000000000000000, 0.7155672824331829052, 1.000000000000000000),
 ( 1.000000000000000000, 0.7060917826293188204, 1.000000000000000000),
 ( 1.000000000000000000, 0.7026601427809967548, 1.000000000000000000),
 ( 1.000000000000000000, 0.6952527892509502427, 1.000000000000000000),
 ( 1.000000000000000000, 0.6912624871067051258, 1.000000000000000000),
 ( 1.000000000000000000, 0.6786163957653905676, 1.000000000000000000),
 ( 1.000000000000000000, 0.6692836425643465814, 1.000000000000000000),
 ( 1.000000000000000000, 0.6490371914779309304, 1.000000000000000000),
 ( 1.000000000000000000, 0.6381215166341221989, 1.000000000000000000),
 ( 1.000000000000000000, 0.6207537710089482408, 1.000000000000000000),
 ( 1.000000000000000000, 0.6147992736454299667, 1.000000000000000000),
 ( 1.000000000000000000, 0.6026007117946927671, 1.000000000000000000),
 ( 1.000000000000000000, 0.5963421480512035577, 1.000000000000000000),
 ( 1.000000000000000000, 0.5773189341497990679, 1.000000000000000000),
 ( 1.000000000000000000, 0.5643376819679217782, 1.000000000000000000),
 ( 1.000000000000000000, 0.5383412250590065007, 1.000000000000000000),
 ( 1.000000000000000000, 0.5253226519624610846, 1.000000000000000000),
 ( 1.000000000000000000, 0.5000277150692035155, 1.000000000000000000),
 ( 1.000000000000000000, 0.4877436159665405335, 1.000000000000000000),
 ( 1.000000000000000000, 0.4650351994093656072, 1.000000000000000000),
 ( 1.000000000000000000, 0.4547962088601842923, 1.000000000000000000),
 ( 1.000000000000000000, 0.4420154047700521338, 1.000000000000000000),
 ( 1.000000000000000000, 0.4381857281609657373, 1.000000000000000000),
 ( 1.000000000000000000, 0.4315381087321277787, 1.000000000000000000),
 ( 1.000000000000000000, 0.4287205967313478805, 1.000000000000000000),
 ( 1.000000000000000000, 0.4242344318730199015, 1.000000000000000000),
 ( 1.000000000000000000, 0.4225662398543922893, 1.000000000000000000),
 ( 1.000000000000000000, 0.4204880647989017173, 1.000000000000000000),
 ( 1.000000000000000000, 0.4200800889062838439, 1.000000000000000000),
 ( 1.000000000000000000, 0.4203293914240995299, 1.000000000000000000) ) ) 
 REPRESENTATION_ITEM ( '' )  SURFACE ( )  );
#8087=AXIS2_PLACEMENT_3D ( 'NONE', #18616, #25220, #23073 ) ;
#8092=DIRECTION ( 'NONE',  ( 0.000000000000000000, 0.000000000000000000, -1.000000000000000000 ) ) ;
#8093=ORIENTED_EDGE ( 'NONE', *, *, #12791, .T. ) ;
#8095=CARTESIAN_POINT ( 'NONE',  ( 0.000000000000000000, -18.01420295945611727, 100.0000000000000000 ) ) ;
#8099=DIRECTION ( 'NONE',  ( 1.000000000000000000, 0.000000000000000000, 0.000000000000000000 ) ) ;
#8101=ORIENTED_EDGE ( 'NONE', *, *, #26992, .T. ) ;
#8105=ORIENTED_EDGE ( 'NONE', *, *, #3994, .T. ) ;
#8106=AXIS2_PLACEMENT_3D ( 'NONE', #11260, #19723, #4481 ) ;
#8107=ORIENTED_EDGE ( 'NONE', *, *, #11215, .T. ) ;
#8111=ORIENTED_EDGE ( 'NONE', *, *, #26805, .F. ) ;
#8115=LINE ( 'NONE', #3653, #5277 ) ;
#8116=DIRECTION ( 'NONE',  ( 0.000000000000000000, 1.000000000000000000, 0.000000000000000000 ) ) ;
#8117=CARTESIAN_POINT ( 'NONE',  ( -71.37541315349507443, 230.0000000000000000, 15.00000000000000000 ) ) ;
#8118=CARTESIAN_POINT ( 'NONE',  ( -200.0000000000000284, -62.36067977499792647, 25.00000000000000000 ) ) ;
#8119=LINE ( 'NONE', #16880, #23651 ) ;
#8121=CARTESIAN_POINT ( 'NONE',  ( -223.4403667166176604, 71.79593500864021394, -19.27754551403313599 ) ) ;
#8122=DIRECTION ( 'NONE',  ( -0.8790438869537371414, -0.4767408570798871148, -0.000000000000000000 ) ) ;
#8126=ORIENTED_EDGE ( 'NONE', *, *, #25021, .T. ) ;
#8129=CARTESIAN_POINT ( 'NONE',  ( 134.9999999999998579, 220.0000000000000284, -100.0000000000000142 ) ) ;
#8130=CARTESIAN_POINT ( 'NONE',  ( 14.18877312265928659, 89.71084980560162592, 98.38498031279395661 ) ) ;
#8140=CARTESIAN_POINT ( 'NONE',  ( -92.83229342711496201, 134.7610587320406239, 15.46096080868298550 ) ) ;
#8141=ORIENTED_EDGE ( 'NONE', *, *, #3636, .F. ) ;
#8142=ORIENTED_EDGE ( 'NONE', *, *, #4671, .T. ) ;
#8143=CARTESIAN_POINT ( 'NONE',  ( 112.6399768800337284, 222.5565040444928115, 96.77053691278567271 ) ) ;
#8144=AXIS2_PLACEMENT_3D ( 'NONE', #13074, #15079, #26120 ) ;
#8146=FACE_OUTER_BOUND ( 'NONE', #16646, .T. ) ;
#8148=CARTESIAN_POINT ( 'NONE',  ( -144.0689309099013258, 125.7628306214139116, -18.57776427790886231 ) ) ;
#8152=CARTESIAN_POINT ( 'NONE',  ( 30.92500016277389108, -41.52323098288959358, 99.96966619038498436 ) ) ;
#8153=CARTESIAN_POINT ( 'NONE',  ( -230.8220000157087668, 92.55346088012031203, -13.02757477273544851 ) ) ;
#8155=CARTESIAN_POINT ( 'NONE',  ( -207.1201485044495030, 89.67250137467401316, 27.42661007367943071 ) ) ;
#8160=VERTEX_POINT ( 'NONE', #20389 ) ;
#8161=AXIS2_PLACEMENT_3D ( 'NONE', #11498, #2852, #850 ) ;
#8165=ORIENTED_EDGE ( 'NONE', *, *, #25672, .T. ) ;
#8167=CARTESIAN_POINT ( 'NONE',  ( 105.7413873646182765, 247.3652972445293017, -29.41146778674738371 ) ) ;
#8169=ORIENTED_EDGE ( 'NONE', *, *, #8054, .T. ) ;
#8170=EDGE_LOOP ( 'NONE', ( #20139, #1826, #7795, #11521, #2046, #8165, #5445, #834, #17214, #14649 ) ) ;
#8174=ORIENTED_EDGE ( 'NONE', *, *, #11047, .T. ) ;
#8176=VECTOR ( 'NONE', #9723, 1000.000000000000000 ) ;
#8178=FACE_BOUND ( 'NONE', #1422, .T. ) ;
#8182=CARTESIAN_POINT ( 'NONE',  ( 9.345921402568846403, 139.9999999999999716, -15.00000000000000000 ) ) ;
#8185=CARTESIAN_POINT ( 'NONE',  ( -210.7172313291012529, 103.7585653882801182, 5.000000000000002665 ) ) ;
#8188=PLANE ( 'NONE',  #1324 ) ;
#8191=ORIENTED_EDGE ( 'NONE', *, *, #13766, .F. ) ;
#8192=CARTESIAN_POINT ( 'NONE',  ( -196.7966726397505681, 98.32233333166497857, 31.72664882486916937 ) ) ;
#8193=CIRCLE ( 'NONE', #25642, 30.00000000000000000 ) ;
#8194=PRODUCT_DEFINITION_SHAPE ( 'NONE', 'NONE',  #13176 ) ;
#8195=EDGE_CURVE ( 'NONE', #22168, #26863, #9772, .T. ) ;
#8197=DIRECTION ( 'NONE',  ( 1.000000000000000000, 3.469446951953614189E-16, -0.000000000000000000 ) ) ;
#8201=VECTOR ( 'NONE', #7792, 1000.000000000000000 ) ;
#8202=ORIENTED_EDGE ( 'NONE', *, *, #20931, .F. ) ;
#8203=CARTESIAN_POINT ( 'NONE',  ( 111.0641325991587252, 99.15168937823351314, 100.0000000000000142 ) ) ;
#8204=EDGE_CURVE ( 'NONE', #6807, #9810, #1853, .T. ) ;
#8206=ORIENTED_EDGE ( 'NONE', *, *, #27503, .F. ) ;
#8207=ORIENTED_EDGE ( 'NONE', *, *, #1721, .T. ) ;
#8209=CYLINDRICAL_SURFACE ( 'NONE', #10220, 5.999999999999991118 ) ;
#8211=CARTESIAN_POINT ( 'NONE',  ( -187.3345487617074809, 105.2479335822991970, -31.76775584780962802 ) ) ;
#8214=CARTESIAN_POINT ( 'NONE',  ( 118.4313905926795769, 122.3304618272157285, 100.0000000000000142 ) ) ;
#8220=DIRECTION ( 'NONE',  ( -1.000000000000000000, 0.000000000000000000, 0.000000000000000000 ) ) ;
#8226=ORIENTED_EDGE ( 'NONE', *, *, #10910, .T. ) ;
#8228=DIRECTION ( 'NONE',  ( -1.000000000000000000, 0.000000000000000000, 0.000000000000000000 ) ) ;
#8231=ORIENTED_EDGE ( 'NONE', *, *, #19170, .T. ) ;
#8235=CARTESIAN_POINT ( 'NONE',  ( 79.99999999999994316, -40.00000000000002842, 100.0000000000000142 ) ) ;
#8236=CARTESIAN_POINT ( 'NONE',  ( -217.8036320994844175, 87.77465520521086262, 17.64589920944733592 ) ) ;
#8250=EDGE_CURVE ( 'NONE', #26218, #16662, #20667, .T. ) ;
#8252=EDGE_LOOP ( 'NONE', ( #17748, #26898, #26108, #8107 ) ) ;
#8256=ADVANCED_FACE ( 'NONE', ( #13950 ), #2360, .T. ) ;
#8259=DIRECTION ( 'NONE',  ( -0.5975062131282553590, 0.8018642810807399268, 0.000000000000000000 ) ) ;
#8260=( BOUNDED_SURFACE ( )  B_SPLINE_SURFACE ( 3, 2, ( 
 ( #1737, #27736, #21282 ),
 ( #10514, #20862, #27451 ),
 ( #19272, #12118, #9949 ),
 ( #7794, #25310, #4175 ),
 ( #15260, #4034, #1876 ),
 ( #17537, #12964, #21715 ),
 ( #13112, #17398, #6334 ),
 ( #21993, #12822, #2446 ),
 ( #11081, #23872, #22 ),
 ( #17119, #2026, #6760 ),
 ( #19838, #2301, #24015 ),
 ( #8643, #10801, #17682 ),
 ( #26012, #4322, #15543 ),
 ( #21565, #10656, #19558 ),
 ( #17257, #4457, #28299 ),
 ( #28161, #8501, #8925 ),
 ( #11229, #15117, #24159 ),
 ( #26158, #8780, #21858 ),
 ( #2162, #26300, #14975 ),
 ( #19415, #26434, #19698 ),
 ( #6480, #10941, #6624 ),
 ( #24291, #15404, #13245 ),
 ( #163, #13385, #4600 ),
 ( #22136, #19980, #311 ),
 ( #25873, #6199, #23724 ),
 ( #22424, #20121, #11527 ),
 ( #597, #26727, #15686 ),
 ( #13824, #24437, #22572 ),
 ( #17972, #11672, #6906 ),
 ( #2736, #737, #16115 ) ),
 .UNSPECIFIED., .F., .F., .T. ) 
 B_SPLINE_SURFACE_WITH_KNOTS ( ( 4, 2, 2, 2, 2, 2, 2, 2, 2, 2, 2, 2, 2, 2, 4 ),
 ( 3, 3 ),
 ( -1.674008154317618846E-16, 0.004796186164130087151, 0.005995232705162650139, 0.007194279246195213993, 0.009592372328260340836, 0.01199046541032546681, 0.01438855849239059452, 0.01918474465652084820, 0.02158283773858597418, 0.02398093082065110015, 0.02877711698478135557, 0.03117521006684648155, 0.03357330314891161099, 0.03597139623097674044, 0.03836948931304186294 ),
 ( 0.000000000000000000, 1.000000000000000000 ),
 .UNSPECIFIED. ) 
 GEOMETRIC_REPRESENTATION_ITEM ( )  RATIONAL_B_SPLINE_SURFACE ( (
 ( 1.000000000000000000, 0.7071067811865487940, 1.000000000000000000),
 ( 1.000000000000000000, 0.7015663335576025617, 1.000000000000000000),
 ( 1.000000000000000000, 0.6988942011281563671, 1.000000000000000000),
 ( 1.000000000000000000, 0.6998716252125488646, 1.000000000000000000),
 ( 1.000000000000000000, 0.7002827442718724260, 1.000000000000000000),
 ( 1.000000000000000000, 0.7015526314445608147, 1.000000000000000000),
 ( 1.000000000000000000, 0.7024157372324350002, 1.000000000000000000),
 ( 1.000000000000000000, 0.7056510234290841455, 1.000000000000000000),
 ( 1.000000000000000000, 0.7086699596806621537, 1.000000000000000000),
 ( 1.000000000000000000, 0.7163055651782664901, 1.000000000000000000),
 ( 1.000000000000000000, 0.7209222552121633543, 1.000000000000000000),
 ( 1.000000000000000000, 0.7316018280031438836, 1.000000000000000000),
 ( 1.000000000000000000, 0.7377022142498353974, 1.000000000000000000),
 ( 1.000000000000000000, 0.7574495109011171179, 1.000000000000000000),
 ( 1.000000000000000000, 0.7725906048390918102, 1.000000000000000000),
 ( 1.000000000000000000, 0.7967368853332368328, 1.000000000000000000),
 ( 1.000000000000000000, 0.8050277828824107251, 1.000000000000000000),
 ( 1.000000000000000000, 0.8218659741008048636, 1.000000000000000000),
 ( 1.000000000000000000, 0.8303227012387988104, 1.000000000000000000),
 ( 1.000000000000000000, 0.8554219935177965750, 1.000000000000000000),
 ( 1.000000000000000000, 0.8718289199487448959, 1.000000000000000000),
 ( 1.000000000000000000, 0.8949179238641020717, 1.000000000000000000),
 ( 1.000000000000000000, 0.9023622371838861955, 1.000000000000000000),
 ( 1.000000000000000000, 0.9165667567816626615, 1.000000000000000000),
 ( 1.000000000000000000, 0.9233430263196975574, 1.000000000000000000),
 ( 1.000000000000000000, 0.9359270949453182276, 1.000000000000000000),
 ( 1.000000000000000000, 0.9416870872377598456, 1.000000000000000000),
 ( 1.000000000000000000, 0.9518583203832227113, 1.000000000000000000),
 ( 1.000000000000000000, 0.9562707360545653623, 1.000000000000000000),
 ( 1.000000000000000000, 0.9597817246759329235, 1.000000000000000000) ) ) 
 REPRESENTATION_ITEM ( '' )  SURFACE ( )  );
#8264=CARTESIAN_POINT ( 'NONE',  ( -232.3551040745953458, 65.57906652092701449, -15.97735746865810214 ) ) ;
#8266=ORIENTED_EDGE ( 'NONE', *, *, #4124, .F. ) ;
#8270=CARTESIAN_POINT ( 'NONE',  ( 112.8630565061748285, 224.0572848923304718, -97.00605251950301522 ) ) ;
#8271=EDGE_LOOP ( 'NONE', ( #16017, #15974 ) ) ;
#8273=DIRECTION ( 'NONE',  ( -0.000000000000000000, -0.000000000000000000, -1.000000000000000000 ) ) ;
#8274=DIRECTION ( 'NONE',  ( -1.000000000000000000, 0.000000000000000000, 0.000000000000000000 ) ) ;
#8286=EDGE_CURVE ( 'NONE', #8829, #14508, #998, .T. ) ;
#8290=CARTESIAN_POINT ( 'NONE',  ( 115.6411010564578561, 208.5333949360010308, 99.00000000000001421 ) ) ;
#8291=CARTESIAN_POINT ( 'NONE',  ( -147.4641305970645533, 124.6152932964712221, -19.24112557280262692 ) ) ;
#8297=CARTESIAN_POINT ( 'NONE',  ( -217.9384205093021194, 87.80450100948937120, -17.58362224480991998 ) ) ;
#8298=EDGE_CURVE ( 'NONE', #7786, #13440, #23002, .T. ) ;
#8301=PLANE ( 'NONE',  #7174 ) ;
#8307=VECTOR ( 'NONE', #11169, 1000.000000000000000 ) ;
#8309=DIRECTION ( 'NONE',  ( -0.000000000000000000, 1.000000000000000000, -1.387778780781445429E-16 ) ) ;
#8315=CARTESIAN_POINT ( 'NONE',  ( 93.89426149340872030, 239.9406732612796986, -18.26413231114277380 ) ) ;
#8319=TOROIDAL_SURFACE ( 'NONE', #2813, 49.99999999999999289, 30.00000000000000000 ) ;
#8325=CARTESIAN_POINT ( 'NONE',  ( -17.24491960465747553, -23.01420295945612082, 80.00000000000001421 ) ) ;
#8334=DIRECTION ( 'NONE',  ( -8.673617379884036705E-17, 1.000000000000000000, 0.000000000000000000 ) ) ;
#8335=LINE ( 'NONE', #25851, #520 ) ;
#8337=AXIS2_PLACEMENT_3D ( 'NONE', #5520, #7686, #27483 ) ;
#8340=CARTESIAN_POINT ( 'NONE',  ( -196.7364259845711274, 98.11380229803960162, 32.13449563926383945 ) ) ;
#8345=ORIENTED_EDGE ( 'NONE', *, *, #10170, .F. ) ;
#8346=EDGE_CURVE ( 'NONE', #20004, #10474, #21175, .T. ) ;
#8348=EDGE_CURVE ( 'NONE', #12401, #88, #23679, .T. ) ;
#8354=CARTESIAN_POINT ( 'NONE',  ( 84.91648909973973502, 110.3843228243604528, -100.0000000000108571 ) ) ;
#8356=CARTESIAN_POINT ( 'NONE',  ( 109.9757146194093878, 258.3900549775689797, 43.60574715434479032 ) ) ;
#8372=ORIENTED_EDGE ( 'NONE', *, *, #20410, .T. ) ;
#8373=AXIS2_PLACEMENT_3D ( 'NONE', #23240, #9606, #18922 ) ;
#8376=CARTESIAN_POINT ( 'NONE',  ( -196.7142546509254828, 98.38667968879231296, 31.27696485703440743 ) ) ;
#8378=CARTESIAN_POINT ( 'NONE',  ( -210.6527369349483081, 88.81635720432898040, 22.91843903506385871 ) ) ;
#8388=CARTESIAN_POINT ( 'NONE',  ( -141.7296954651576755, 126.5025729468090816, 18.19659924392545136 ) ) ;
#8389=EDGE_CURVE ( 'NONE', #230, #23293, #19929, .T. ) ;
#8390=CARTESIAN_POINT ( 'NONE',  ( -180.5882078327868214, 109.6574160033507468, -29.97001359623425643 ) ) ;
#8391=ORIENTED_EDGE ( 'NONE', *, *, #23750, .T. ) ;
#8397=CIRCLE ( 'NONE', #8868, 1.999999999999997113 ) ;
#8400=DIRECTION ( 'NONE',  ( 1.000000000000000000, 0.000000000000000000, 0.000000000000000000 ) ) ;
#8405=CARTESIAN_POINT ( 'NONE',  ( -234.0991496467425463, 66.75367139654701987, -6.159314286175092690 ) ) ;
#8409=CARTESIAN_POINT ( 'NONE',  ( -210.0000000000000000, -120.0000000000001705, 100.0000000000000142 ) ) ;
#8411=VERTEX_POINT ( 'NONE', #6853 ) ;
#8414=ADVANCED_FACE ( 'NONE', ( #15783 ), #3287, .T. ) ;
#8423=AXIS2_PLACEMENT_3D ( 'NONE', #9691, #11856, #18453 ) ;
#8426=EDGE_CURVE ( 'NONE', #14300, #16598, #538, .T. ) ;
#8429=AXIS2_PLACEMENT_3D ( 'NONE', #12275, #5506, #783 ) ;
#8434=ORIENTED_EDGE ( 'NONE', *, *, #5342, .T. ) ;
#8435=CARTESIAN_POINT ( 'NONE',  ( -216.4421519707229606, 141.6000904446840707, 15.00000000000000000 ) ) ;
#8436=CARTESIAN_POINT ( 'NONE',  ( -96.34017497949227504, 134.5464908775736887, -15.49978530010318956 ) ) ;
#8437=PLANE ( 'NONE',  #17551 ) ;
#8438=CARTESIAN_POINT ( 'NONE',  ( -151.5242873510758272, 124.1880030070812921, -19.47963555966862970 ) ) ;
#8441=LINE ( 'NONE', #8583, #26400 ) ;
#8442=CARTESIAN_POINT ( 'NONE',  ( -222.3167885473197600, 86.50371922326300478, -17.61937429740468630 ) ) ;
#8444=CARTESIAN_POINT ( 'NONE',  ( -210.0000000000000284, 59.99999999999993605, 100.0000000000000142 ) ) ;
#8445=EDGE_CURVE ( 'NONE', #19837, #19335, #14303, .T. ) ;
#8448=FACE_OUTER_BOUND ( 'NONE', #25584, .T. ) ;
#8450=ORIENTED_EDGE ( 'NONE', *, *, #14671, .T. ) ;
#8452=FACE_OUTER_BOUND ( 'NONE', #2386, .T. ) ;
#8454=DIRECTION ( 'NONE',  ( 0.000000000000000000, 0.000000000000000000, 1.000000000000000000 ) ) ;
#8456=ORIENTED_EDGE ( 'NONE', *, *, #6899, .F. ) ;
#8457=CARTESIAN_POINT ( 'NONE',  ( 106.7826897485120696, 249.1041097334270091, -25.92390487272609079 ) ) ;
#8466=ORIENTED_EDGE ( 'NONE', *, *, #15885, .T. ) ;
#8467=DIRECTION ( 'NONE',  ( 0.000000000000000000, 0.000000000000000000, -1.000000000000000000 ) ) ;
#8474=CARTESIAN_POINT ( 'NONE',  ( -229.8504134091503204, 74.77134060501161628, -16.24524307967075032 ) ) ;
#8475=VECTOR ( 'NONE', #23411, 1000.000000000000000 ) ;
#8476=ADVANCED_FACE ( 'NONE', ( #961 ), #3387, .F. ) ;
#8477=CARTESIAN_POINT ( 'NONE',  ( -28.13887543485015286, 129.1552015491647865, 15.69125477524985257 ) ) ;
#8481=VECTOR ( 'NONE', #13625, 1000.000000000000000 ) ;
#8483=CARTESIAN_POINT ( 'NONE',  ( -180.3681537315997900, 109.4804799639990875, 30.93612761857035309 ) ) ;
#8484=LINE ( 'NONE', #12808, #25480 ) ;
#8490=CARTESIAN_POINT ( 'NONE',  ( -227.8378063125350366, 130.6400894613935577, -13.00000000000000178 ) ) ;
#8491=LINE ( 'NONE', #19405, #25513 ) ;
#8497=CARTESIAN_POINT ( 'NONE',  ( 111.0641325991587252, 99.15168937823352735, -100.0000000000000142 ) ) ;
#8498=CARTESIAN_POINT ( 'NONE',  ( 91.02001408115319236, 230.3620936502381085, 17.09243702347552585 ) ) ;
#8501=CARTESIAN_POINT ( 'NONE',  ( -216.8679380397482248, 87.78479877776845797, 20.07711282125457330 ) ) ;
#8502=EDGE_LOOP ( 'NONE', ( #7235, #22200, #27766, #10131 ) ) ;
#8506=CARTESIAN_POINT ( 'NONE',  ( -43.02437977270766112, 129.0347155322979233, -14.93735646117640492 ) ) ;
#8509=ADVANCED_FACE ( 'NONE', ( #11897 ), #6962, .F. ) ;
#8514=ADVANCED_FACE ( 'NONE', ( #18213 ), #3731, .T. ) ;
#8515=CARTESIAN_POINT ( 'NONE',  ( 134.9999999999998579, 330.0000000000000000, 84.99999999999995737 ) ) ;
#8519=VERTEX_POINT ( 'NONE', #4977 ) ;
#8520=CIRCLE ( 'NONE', #24577, 30.00000000000000000 ) ;
#8522=CARTESIAN_POINT ( 'NONE',  ( -178.9773280279911205, 110.6332285672180120, 29.32662861827880363 ) ) ;
#8523=CARTESIAN_POINT ( 'NONE',  ( -40.77942248602414566, 129.1863037768054596, -17.01095293969337519 ) ) ;
#8528=ORIENTED_EDGE ( 'NONE', *, *, #14485, .F. ) ;
#8530=CARTESIAN_POINT ( 'NONE',  ( -163.7479997171323305, 118.1529936970674726, -24.32116846398825416 ) ) ;
#8534=CARTESIAN_POINT ( 'NONE',  ( -71.37541315349507443, 150.2892445414773590, 5.000000000000002665 ) ) ;
#8536=AXIS2_PLACEMENT_3D ( 'NONE', #13499, #17653, #21829 ) ;
#8538=VERTEX_POINT ( 'NONE', #24955 ) ;
#8541=DIRECTION ( 'NONE',  ( -0.000000000000000000, -0.000000000000000000, 1.000000000000000000 ) ) ;
#8545=EDGE_CURVE ( 'NONE', #24488, #7444, #5271, .T. ) ;
#8546=EDGE_CURVE ( 'NONE', #2404, #20577, #18435, .T. ) ;
#8549=CARTESIAN_POINT ( 'NONE',  ( -222.1843861435924907, 71.54148064076224500, -20.10873357379266935 ) ) ;
#8555=CARTESIAN_POINT ( 'NONE',  ( 112.8464227643157329, 215.9386697890600999, -96.99047740776124726 ) ) ;
#8557=CARTESIAN_POINT ( 'NONE',  ( -224.2511286692390513, 62.13136325095026535, 9.143584677369513969 ) ) ;
#8559=DIRECTION ( 'NONE',  ( -1.000000000000000000, 0.000000000000000000, 0.000000000000000000 ) ) ;
#8564=CARTESIAN_POINT ( 'NONE',  ( -235.6754299164472854, 80.57958899222390414, 15.03010587785140650 ) ) ;
#8568=AXIS2_PLACEMENT_3D ( 'NONE', #530, #7704, #18203 ) ;
#8570=LINE ( 'NONE', #6549, #1661 ) ;
#8571=EDGE_CURVE ( 'NONE', #16727, #12559, #22100, .T. ) ;
#8572=ORIENTED_EDGE ( 'NONE', *, *, #5268, .F. ) ;
#8573=ORIENTED_EDGE ( 'NONE', *, *, #11750, .F. ) ;
#8575=DIRECTION ( 'NONE',  ( 1.000000000000000000, 0.000000000000000000, 0.000000000000000000 ) ) ;
#8577=CARTESIAN_POINT ( 'NONE',  ( 48.45469728424487244, 192.9461374953035033, 15.00000000000000000 ) ) ;
#8583=CARTESIAN_POINT ( 'NONE',  ( 79.99999999999992895, 240.0000000000000284, 5.000000000000002665 ) ) ;
#8584=CARTESIAN_POINT ( 'NONE',  ( -219.8865548899133842, 87.95092811395369381, -16.46640705182500497 ) ) ;
#8592=DIRECTION ( 'NONE',  ( 0.000000000000000000, 0.000000000000000000, -1.000000000000000000 ) ) ;
#8597=CARTESIAN_POINT ( 'NONE',  ( 106.7420202941123080, 244.4253804639438670, -31.38183343148740789 ) ) ;
#8599=DIRECTION ( 'NONE',  ( 1.000000000000000000, 2.602085213965211135E-16, -0.000000000000000000 ) ) ;
#8600=ORIENTED_EDGE ( 'NONE', *, *, #9379, .F. ) ;
#8603=ORIENTED_EDGE ( 'NONE', *, *, #19756, .F. ) ;
#8606=CARTESIAN_POINT ( 'NONE',  ( -17.24491960465745777, 24.64876300893806160, 95.00000000000000000 ) ) ;
#8608=PLANE ( 'NONE',  #3190 ) ;
#8612=CIRCLE ( 'NONE', #4926, 21.49999999999999289 ) ;
#8619=DIRECTION ( 'NONE',  ( 0.000000000000000000, 0.000000000000000000, 1.000000000000000000 ) ) ;
#8620=ADVANCED_FACE ( 'NONE', ( #28075 ), #25511, .F. ) ;
#8621=FACE_OUTER_BOUND ( 'NONE', #5014, .T. ) ;
#8623=DIRECTION ( 'NONE',  ( 1.000000000000000000, -0.000000000000000000, -0.000000000000000000 ) ) ;
#8627=CARTESIAN_POINT ( 'NONE',  ( -233.2943309833541718, 92.06151970357193193, -15.00000000000000000 ) ) ;
#8634=CARTESIAN_POINT ( 'NONE',  ( -224.0246150495856625, 134.1142769380917912, -12.98324324876687719 ) ) ;
#8635=DIRECTION ( 'NONE',  ( 0.000000000000000000, 0.000000000000000000, -1.000000000000000000 ) ) ;
#8636=B_SPLINE_CURVE_WITH_KNOTS ( 'NONE', 3,
 ( #24070, #2211, #72, #8834, #6678, #15456, #22629, #9415, #15743, #11136, #7399, #2496, #24490, #11578, #26930, #19891, #5232, #7108, #4650, #16166, #4799, #361, #13586, #13732 ),
 .UNSPECIFIED., .F., .F.,
 ( 4, 2, 2, 2, 2, 2, 2, 2, 2, 2, 2, 4 ),
 ( 0.000000000000000000, 0.005230979107866756510, 0.01046195821573351302, 0.01307744776966689344, 0.01569293732360027213, 0.02092391643146711971, 0.02353940598540057300, 0.02615489553933402281, 0.03138587464720085651, 0.03400136420113424041, 0.03661685375506761042, 0.04184783286293437127 ),
 .UNSPECIFIED. ) ;
#8638=ORIENTED_EDGE ( 'NONE', *, *, #15780, .F. ) ;
#8639=CARTESIAN_POINT ( 'NONE',  ( 109.9999999999999432, 140.0000000000000000, -100.0000000000000142 ) ) ;
#8641=CARTESIAN_POINT ( 'NONE',  ( -178.8341066938216386, 110.7300218161632444, -29.28299286780852029 ) ) ;
#8643=CARTESIAN_POINT ( 'NONE',  ( -223.0240206785557859, 86.63361387472085084, 17.31476664850702107 ) ) ;
#8648=DIRECTION ( 'NONE',  ( 0.000000000000000000, -0.000000000000000000, 1.000000000000000000 ) ) ;
#8649=AXIS2_PLACEMENT_3D ( 'NONE', #24102, #17058, #25817 ) ;
#8660=CARTESIAN_POINT ( 'NONE',  ( -162.7087466801204698, 119.3764571194343915, 22.15020238234947669 ) ) ;
#8661=CARTESIAN_POINT ( 'NONE',  ( -214.1043220540802565, 88.03185359167697754, 20.18450238099627825 ) ) ;
#8662=ORIENTED_EDGE ( 'NONE', *, *, #9300, .F. ) ;
#8663=ORIENTED_EDGE ( 'NONE', *, *, #445, .T. ) ;
#8666=CARTESIAN_POINT ( 'NONE',  ( -215.4886702565632106, 139.8420026707766226, 12.99999999999999822 ) ) ;
#8668=CARTESIAN_POINT ( 'NONE',  ( -186.8676103567957227, 105.5662940401322629, -31.69060553503991073 ) ) ;
#8670=ORIENTED_EDGE ( 'NONE', *, *, #23217, .T. ) ;
#8672=VECTOR ( 'NONE', #8971, 1000.000000000000000 ) ;
#8676=ORIENTED_EDGE ( 'NONE', *, *, #6653, .F. ) ;
#8678=FACE_BOUND ( 'NONE', #4061, .T. ) ;
#8681=FACE_OUTER_BOUND ( 'NONE', #5238, .T. ) ;
#8684=LINE ( 'NONE', #6801, #2245 ) ;
#8685=ORIENTED_EDGE ( 'NONE', *, *, #11674, .F. ) ;
#8694=AXIS2_PLACEMENT_3D ( 'NONE', #15061, #2249, #22083 ) ;
#8696=CARTESIAN_POINT ( 'NONE',  ( -210.0000000000000000, -150.0000000000002558, 100.0000000000000142 ) ) ;
#8698=LINE ( 'NONE', #10716, #12925 ) ;
#8699=CARTESIAN_POINT ( 'NONE',  ( -112.3221550338875687, 17.24192588826928585, 83.00000000000001421 ) ) ;
#8701=CARTESIAN_POINT ( 'NONE',  ( -226.4422656491013299, 72.85741102083747478, 17.64402269315965910 ) ) ;
#8702=ORIENTED_EDGE ( 'NONE', *, *, #14087, .F. ) ;
#8704=EDGE_LOOP ( 'NONE', ( #16486, #22487, #6406, #3568 ) ) ;
#8708=AXIS2_PLACEMENT_3D ( 'NONE', #28175, #4336, #4469 ) ;
#8715=CIRCLE ( 'NONE', #1907, 49.99999999999998579 ) ;
#8716=CARTESIAN_POINT ( 'NONE',  ( -160.0000000000000284, 59.99999999999994316, 110.0000000000000284 ) ) ;
#8717=FACE_OUTER_BOUND ( 'NONE', #9079, .T. ) ;
#8720=CARTESIAN_POINT ( 'NONE',  ( -215.3975081536182756, 87.85043416605050481, -19.22867602304995671 ) ) ;
#8724=DIRECTION ( 'NONE',  ( -0.000000000000000000, -0.000000000000000000, -1.000000000000000000 ) ) ;
#8733=ORIENTED_EDGE ( 'NONE', *, *, #20852, .F. ) ;
#8734=AXIS2_PLACEMENT_3D ( 'NONE', #6303, #21396, #10769 ) ;
#8735=CARTESIAN_POINT ( 'NONE',  ( 99.67744569821567779, 242.4823527582474014, -13.37113024292605878 ) ) ;
#8737=CARTESIAN_POINT ( 'NONE',  ( -40.35451784973074751, 130.4209458812801756, -15.14568436839074117 ) ) ;
#8740=ORIENTED_EDGE ( 'NONE', *, *, #13712, .T. ) ;
#8746=CARTESIAN_POINT ( 'NONE',  ( 115.6411010564592061, 231.4666050640012998, 99.00000000000001421 ) ) ;
#8749=DIRECTION ( 'NONE',  ( 0.000000000000000000, 0.000000000000000000, -1.000000000000000000 ) ) ;
#8752=CARTESIAN_POINT ( 'NONE',  ( -215.0107612850210899, 71.82996193033663701, 26.64107447012230878 ) ) ;
#8754=DIRECTION ( 'NONE',  ( 1.000000000000000000, 0.000000000000000000, -0.000000000000000000 ) ) ;
#8755=CARTESIAN_POINT ( 'NONE',  ( 134.9999999999998579, 171.5103103742661688, -84.99999999999997158 ) ) ;
#8758=CARTESIAN_POINT ( 'NONE',  ( 33.10302365956999182, 203.2034914284457159, -15.00000000000000000 ) ) ;
#8763=ORIENTED_EDGE ( 'NONE', *, *, #11750, .T. ) ;
#8764=VERTEX_POINT ( 'NONE', #4376 ) ;
#8765=CARTESIAN_POINT ( 'NONE',  ( -160.5161435040798779, 120.3804527765386752, 22.28951900308573286 ) ) ;
#8768=DIRECTION ( 'NONE',  ( 1.000000000000000000, -0.000000000000000000, -0.000000000000000000 ) ) ;
#8769=ORIENTED_EDGE ( 'NONE', *, *, #3961, .T. ) ;
#8773=DIRECTION ( 'NONE',  ( 1.000000000000000000, 0.000000000000000000, 0.000000000000000000 ) ) ;
#8774=CARTESIAN_POINT ( 'NONE',  ( -273.6211430000234373, -91.18033988749901653, 0.000000000000000000 ) ) ;
#8776=VERTEX_POINT ( 'NONE', #24073 ) ;
#8780=CARTESIAN_POINT ( 'NONE',  ( -214.9847395972752508, 87.90486964456984254, 21.25064676488950255 ) ) ;
#8799=VECTOR ( 'NONE', #22472, 1000.000000000000000 ) ;
#8802=CARTESIAN_POINT ( 'NONE',  ( -192.2959713312834538, 101.7311354626386333, -32.42984626233510426 ) ) ;
#8805=ORIENTED_EDGE ( 'NONE', *, *, #26998, .F. ) ;
#8806=FACE_OUTER_BOUND ( 'NONE', #9492, .T. ) ;
#8809=EDGE_CURVE ( 'NONE', #606, #26119, #17522, .T. ) ;
#8812=DIRECTION ( 'NONE',  ( -0.7892793597178168197, -0.6140342761796225846, 2.738362868812879575E-15 ) ) ;
#8820=CARTESIAN_POINT ( 'NONE',  ( -175.0000000000000000, -120.0000000000001705, 76.02500000000001990 ) ) ;
#8822=EDGE_CURVE ( 'NONE', #22331, #13033, #9747, .T. ) ;
#8823=AXIS2_PLACEMENT_3D ( 'NONE', #25563, #1582, #12664 ) ;
#8825=DIRECTION ( 'NONE',  ( -0.000000000000000000, -0.000000000000000000, -1.000000000000000000 ) ) ;
#8828=LINE ( 'NONE', #17729, #2456 ) ;
#8829=VERTEX_POINT ( 'NONE', #8699 ) ;
#8831=VECTOR ( 'NONE', #14156, 1000.000000000000114 ) ;
#8834=CARTESIAN_POINT ( 'NONE',  ( -239.7229382034104788, 70.94047833162919403, -5.249966640536483986 ) ) ;
#8836=CARTESIAN_POINT ( 'NONE',  ( -68.57415822541635464, -23.01420295945612082, 80.00000000000001421 ) ) ;
#8839=CARTESIAN_POINT ( 'NONE',  ( -227.7492452350401493, 73.49917159638472697, 17.05328293002254014 ) ) ;
#8851=CARTESIAN_POINT ( 'NONE',  ( -225.9601317720700990, 132.4444111280423613, 15.07876772301852064 ) ) ;
#8852=CARTESIAN_POINT ( 'NONE',  ( 96.18084660807321029, 232.2996298045118522, 19.72083291508481295 ) ) ;
#8856=FACE_OUTER_BOUND ( 'NONE', #50, .T. ) ;
#8860=FACE_OUTER_BOUND ( 'NONE', #20208, .T. ) ;
#8868=AXIS2_PLACEMENT_3D ( 'NONE', #4920, #8812, #17858 ) ;
#8870=EDGE_CURVE ( 'NONE', #18977, #3239, #18458, .T. ) ;
#8872=CARTESIAN_POINT ( 'NONE',  ( 111.2621361164573131, 140.0000000000000000, 95.03618980370902136 ) ) ;
#8874=EDGE_CURVE ( 'NONE', #5833, #26994, #20607, .T. ) ;
#8882=ORIENTED_EDGE ( 'NONE', *, *, #26431, .T. ) ;
#8884=EDGE_CURVE ( 'NONE', #8985, #19265, #27596, .T. ) ;
#8885=ORIENTED_EDGE ( 'NONE', *, *, #15432, .F. ) ;
#8894=CARTESIAN_POINT ( 'NONE',  ( -214.6111699653978349, 58.62522005596079566, 31.77808924749080788 ) ) ;
#8896=DIRECTION ( 'NONE',  ( -1.000000000000000000, 0.000000000000000000, 0.000000000000000000 ) ) ;
#8898=DIRECTION ( 'NONE',  ( -0.000000000000000000, -0.000000000000000000, 1.000000000000000000 ) ) ;
#8901=ADVANCED_FACE ( 'NONE', ( #20325 ), #10192, .T. ) ;
#8902=ADVANCED_FACE ( 'NONE', ( #9419 ), #20469, .T. ) ;
#8905=EDGE_CURVE ( 'NONE', #23195, #15531, #14025, .T. ) ;
#8906=CARTESIAN_POINT ( 'NONE',  ( 51.56615429303207065, 203.2034914284457159, 15.00000000000000000 ) ) ;
#8909=ORIENTED_EDGE ( 'NONE', *, *, #27850, .F. ) ;
#8910=EDGE_LOOP ( 'NONE', ( #8670, #21267 ) ) ;
#8912=CARTESIAN_POINT ( 'NONE',  ( -224.1705500038237346, 86.90025305032594360, -16.85721464638110234 ) ) ;
#8913=CARTESIAN_POINT ( 'NONE',  ( -203.9013263906359441, 92.43596962530546080, -29.05832367954837281 ) ) ;
#8916=VERTEX_POINT ( 'NONE', #5236 ) ;
#8918=CARTESIAN_POINT ( 'NONE',  ( -226.9194690495522764, 131.5555540326517985, -13.00000000000000178 ) ) ;
#8919=CARTESIAN_POINT ( 'NONE',  ( -137.5210505075045262, 129.0054383906156374, 17.05624534316643803 ) ) ;
#8921=CARTESIAN_POINT ( 'NONE',  ( 94.38583646783695258, 113.6320904521875548, -75.15625000023771918 ) ) ;
#8925=CARTESIAN_POINT ( 'NONE',  ( -216.0630910827463254, 87.83017798286152811, 18.79139027124664096 ) ) ;
#8926=CIRCLE ( 'NONE', #19018, 5.000000000000004441 ) ;
#8928=LINE ( 'NONE', #17403, #3400 ) ;
#8929=AXIS2_PLACEMENT_3D ( 'NONE', #27965, #21514, #4127 ) ;
#8931=EDGE_CURVE ( 'NONE', #1390, #14300, #24639, .T. ) ;
#8937=DIRECTION ( 'NONE',  ( -0.8314772792026879911, 0.5555587585212703461, 0.000000000000000000 ) ) ;
#8941=CARTESIAN_POINT ( 'NONE',  ( -143.0445616319559008, 68.96623314385857384, 82.96749942560525426 ) ) ;
#8942=ORIENTED_EDGE ( 'NONE', *, *, #25848, .F. ) ;
#8945=EDGE_LOOP ( 'NONE', ( #9879, #2319, #24213, #15036, #10800 ) ) ;
#8948=CARTESIAN_POINT ( 'NONE',  ( -185.5061758263113632, 106.4823051942665302, -31.41754718802355839 ) ) ;
#8949=VERTEX_POINT ( 'NONE', #12566 ) ;
#8950=CIRCLE ( 'NONE', #25010, 2.586968381275096984 ) ;
#8956=CARTESIAN_POINT ( 'NONE',  ( -0.4700637257060664709, 134.1129467060154070, 15.56863088294750064 ) ) ;
#8958=CYLINDRICAL_SURFACE ( 'NONE', #19525, 41.00000000000000711 ) ;
#8964=CARTESIAN_POINT ( 'NONE',  ( -209.4684130045736197, 67.32370550333207859, -34.40586572994357084 ) ) ;
#8965=DIRECTION ( 'NONE',  ( 0.000000000000000000, 1.000000000000000000, 0.000000000000000000 ) ) ;
#8966=VERTEX_POINT ( 'NONE', #5800 ) ;
#8971=DIRECTION ( 'NONE',  ( 0.000000000000000000, 0.000000000000000000, -1.000000000000000000 ) ) ;
#8974=CARTESIAN_POINT ( 'NONE',  ( -215.0412094859541980, 60.20193349634168101, 13.76727271988285040 ) ) ;
#8976=EDGE_CURVE ( 'NONE', #2948, #27477, #22139, .T. ) ;
#8978=DIRECTION ( 'NONE',  ( 1.000000000000000000, -0.000000000000000000, -0.000000000000000000 ) ) ;
#8985=VERTEX_POINT ( 'NONE', #5661 ) ;
#8987=ORIENTED_EDGE ( 'NONE', *, *, #13845, .F. ) ;
#8990=CIRCLE ( 'NONE', #24125, 6.025000000000002132 ) ;
#8996=ORIENTED_EDGE ( 'NONE', *, *, #9459, .T. ) ;
#8997=CARTESIAN_POINT ( 'NONE',  ( -220.9676528974450491, 136.4492860810096317, 15.12837422688856925 ) ) ;
#8998=CARTESIAN_POINT ( 'NONE',  ( 102.0190107526936174, 244.0003474240143078, 16.44012727447546496 ) ) ;
#9001=DIRECTION ( 'NONE',  ( -0.000000000000000000, 1.000000000000000000, -1.387778780781445429E-16 ) ) ;
#9007=CARTESIAN_POINT ( 'NONE',  ( -230.8916957670046486, 130.8330661503599117, -15.00000000000000000 ) ) ;
#9010=VECTOR ( 'NONE', #15, 1000.000000000000000 ) ;
#9013=ADVANCED_FACE ( 'NONE', ( #23607 ), #3778, .F. ) ;
#9016=DIRECTION ( 'NONE',  ( -2.602085213965210642E-16, 1.000000000000000000, 0.000000000000000000 ) ) ;
#9017=CARTESIAN_POINT ( 'NONE',  ( -225.7036482868739427, -91.18033988749901653, -18.91107291867258411 ) ) ;
#9018=( BOUNDED_SURFACE ( )  B_SPLINE_SURFACE ( 3, 2, ( 
 ( #10073, #23420, #14389 ),
 ( #3730, #21406, #1720 ),
 ( #23147, #19253, #23001 ),
 ( #8340, #8192, #18825 ),
 ( #12243, #27573, #25435 ),
 ( #25150, #12520, #12103 ),
 ( #16681, #27715, #21264 ),
 ( #5755, #14529, #16822 ),
 ( #25997, #10638, #28143 ),
 ( #12945, #11065, #23709 ),
 ( #17666, #10921, #19394 ),
 ( #21696, #2286, #13370 ),
 ( #8483, #10784, #11210 ),
 ( #17520, #15245, #6744 ),
 ( #21548, #17237, #6180 ),
 ( #25855, #19819, #4159 ),
 ( #2007, #4584, #23998 ),
 ( #26419, #19682, #19542 ),
 ( #4309, #6, #6315 ),
 ( #14956, #24143, #2148 ),
 ( #19964, #12802, #21842 ),
 ( #13094, #8765, #22121 ) ),
 .UNSPECIFIED., .F., .F., .F. ) 
 B_SPLINE_SURFACE_WITH_KNOTS ( ( 4, 2, 2, 2, 2, 2, 2, 2, 2, 2, 4 ),
 ( 3, 3 ),
 ( 0.000000000000000000, 0.006464363597911549145, 0.01292872719582309829, 0.01616090899477887199, 0.01939309079373464917, 0.02585745439164619658, 0.02908963619060197028, 0.03232181798955774399, 0.03878618158746929834, 0.04525054518538084575, 0.05171490878329239316 ),
 ( 0.000000000000000000, 1.000000000000000000 ),
 .UNSPECIFIED. ) 
 GEOMETRIC_REPRESENTATION_ITEM ( )  RATIONAL_B_SPLINE_SURFACE ( (
 ( 1.000000000000000000, 0.9597817246759321463, 1.000000000000000000),
 ( 1.000000000000000000, 0.9644978604548086754, 1.000000000000000000),
 ( 1.000000000000000000, 0.9684366129255929101, 1.000000000000000000),
 ( 1.000000000000000000, 0.9744801429909556445, 1.000000000000000000),
 ( 1.000000000000000000, 0.9765856948512464664, 1.000000000000000000),
 ( 1.000000000000000000, 0.9781316547679167472, 1.000000000000000000),
 ( 1.000000000000000000, 0.9783777913778298752, 1.000000000000000000),
 ( 1.000000000000000000, 0.9782912468864014555, 1.000000000000000000),
 ( 1.000000000000000000, 0.9779594306925435410, 1.000000000000000000),
 ( 1.000000000000000000, 0.9761609493688950812, 1.000000000000000000),
 ( 1.000000000000000000, 0.9738931452053198878, 1.000000000000000000),
 ( 1.000000000000000000, 0.9691275407867268044, 1.000000000000000000),
 ( 1.000000000000000000, 0.9673113114069962215, 1.000000000000000000),
 ( 1.000000000000000000, 0.9632590755101273494, 1.000000000000000000),
 ( 1.000000000000000000, 0.9610203127353997843, 1.000000000000000000),
 ( 1.000000000000000000, 0.9537484340619055700, 1.000000000000000000),
 ( 1.000000000000000000, 0.9481631559643158846, 1.000000000000000000),
 ( 1.000000000000000000, 0.9357596895728105268, 1.000000000000000000),
 ( 1.000000000000000000, 0.9289410327529883382, 1.000000000000000000),
 ( 1.000000000000000000, 0.9142674582240357672, 1.000000000000000000),
 ( 1.000000000000000000, 0.9064119848472056429, 1.000000000000000000),
 ( 1.000000000000000000, 0.8981184559478653240, 1.000000000000000000) ) ) 
 REPRESENTATION_ITEM ( '' )  SURFACE ( )  );
#9021=CARTESIAN_POINT ( 'NONE',  ( 109.9999999999998863, 260.0000000000000000, -45.00000000000000000 ) ) ;
#9023=DIRECTION ( 'NONE',  ( 0.000000000000000000, 0.000000000000000000, 1.000000000000000000 ) ) ;
#9028=ORIENTED_EDGE ( 'NONE', *, *, #17194, .F. ) ;
#9031=VECTOR ( 'NONE', #6931, 1000.000000000000000 ) ;
#9032=LINE ( 'NONE', #13640, #20532 ) ;
#9038=CARTESIAN_POINT ( 'NONE',  ( -212.5256769160629631, 72.66764018259519275, 29.94823517519424527 ) ) ;
#9039=FACE_OUTER_BOUND ( 'NONE', #20536, .T. ) ;
#9045=CARTESIAN_POINT ( 'NONE',  ( 4.492022713026529779, 138.9219254684496718, 13.09535121465864727 ) ) ;
#9047=CARTESIAN_POINT ( 'NONE',  ( -167.6265986190112187, 116.3518912474305296, 25.91344288888009473 ) ) ;
#9054=CARTESIAN_POINT ( 'NONE',  ( -205.5650550490929902, 90.70191985663102230, -28.50364138414912318 ) ) ;
#9055=EDGE_LOOP ( 'NONE', ( #19863, #13100, #8126, #335 ) ) ;
#9056=ORIENTED_EDGE ( 'NONE', *, *, #24444, .F. ) ;
#9059=CARTESIAN_POINT ( 'NONE',  ( -137.1120637285174269, 127.8502071294020368, 17.56806758514733247 ) ) ;
#9064=ADVANCED_FACE ( 'NONE', ( #6079 ), #14861, .T. ) ;
#9068=VECTOR ( 'NONE', #2129, 1000.000000000000000 ) ;
#9073=CARTESIAN_POINT ( 'NONE',  ( -214.0383293111087539, 72.11341309493322171, -27.85175881924293506 ) ) ;
#9076=CARTESIAN_POINT ( 'NONE',  ( -225.9729034214342391, 132.4331356209129922, -12.99353264123096885 ) ) ;
#9077=CARTESIAN_POINT ( 'NONE',  ( -180.0000000000000284, -40.00000000000004974, 70.00000000000000000 ) ) ;
#9079=EDGE_LOOP ( 'NONE', ( #28396, #16623, #4703, #7408 ) ) ;
#9085=CARTESIAN_POINT ( 'NONE',  ( -142.3242417476000981, 69.93676590415873306, 82.90331240453681971 ) ) ;
#9086=ORIENTED_EDGE ( 'NONE', *, *, #24082, .F. ) ;
#9087=ORIENTED_EDGE ( 'NONE', *, *, #5464, .T. ) ;
#9089=CARTESIAN_POINT ( 'NONE',  ( -199.9534950421034125, 95.77273280906791797, -30.16924513461026081 ) ) ;
#9093=EDGE_CURVE ( 'NONE', #4814, #17928, #24852, .T. ) ;
#9100=ORIENTED_EDGE ( 'NONE', *, *, #8077, .F. ) ;
#9102=AXIS2_PLACEMENT_3D ( 'NONE', #16912, #13570, #11119 ) ;
#9105=CARTESIAN_POINT ( 'NONE',  ( -27.08985507592738173, 129.1630599246555562, -15.68767261356309284 ) ) ;
#9107=DIRECTION ( 'NONE',  ( -1.000000000000000000, -8.673617379884036705E-17, -0.000000000000000000 ) ) ;
#9108=CARTESIAN_POINT ( 'NONE',  ( -180.0000000000000284, -50.00000000000004263, 110.0000000000000284 ) ) ;
#9118=LINE ( 'NONE', #26208, #3817 ) ;
#9119=DIRECTION ( 'NONE',  ( 0.000000000000000000, 0.000000000000000000, 1.000000000000000000 ) ) ;
#9123=ORIENTED_EDGE ( 'NONE', *, *, #549, .T. ) ;
#9124=CIRCLE ( 'NONE', #19683, 22.49999999999999289 ) ;
#9133=CIRCLE ( 'NONE', #14188, 53.86582179324592090 ) ;
#9138=ORIENTED_EDGE ( 'NONE', *, *, #22171, .T. ) ;
#9139=CARTESIAN_POINT ( 'NONE',  ( 98.16608178754300695, 241.2913188899314036, 20.91842009985186124 ) ) ;
#9143=AXIS2_PLACEMENT_3D ( 'NONE', #1395, #18921, #18366 ) ;
#9145=DIRECTION ( 'NONE',  ( 1.000000000000000000, 0.000000000000000000, 0.000000000000000000 ) ) ;
#9147=DIRECTION ( 'NONE',  ( 0.000000000000000000, 1.000000000000000000, 0.000000000000000000 ) ) ;
#9148=CARTESIAN_POINT ( 'NONE',  ( 134.9999999999998579, 220.0000000000000284, -105.0000000000000284 ) ) ;
#9152=DIRECTION ( 'NONE',  ( -0.000000000000000000, 1.000000000000000000, -1.387778780781445429E-16 ) ) ;
#9153=DIRECTION ( 'NONE',  ( -0.000000000000000000, 0.000000000000000000, 1.000000000000000000 ) ) ;
#9155=EDGE_LOOP ( 'NONE', ( #22309, #9317, #17220, #1912 ) ) ;
#9161=VERTEX_POINT ( 'NONE', #439 ) ;
#9167=VERTEX_POINT ( 'NONE', #15138 ) ;
#9175=CIRCLE ( 'NONE', #16960, 10.70611877156249214 ) ;
#9176=ADVANCED_FACE ( 'NONE', ( #2575 ), #1037, .T. ) ;
#9178=DIRECTION ( 'NONE',  ( -1.530283246943720875E-16, 1.000000000000000000, -0.000000000000000000 ) ) ;
#9180=CARTESIAN_POINT ( 'NONE',  ( -220.6363270246480965, 61.10744949787188318, 10.70339401868985796 ) ) ;
#9181=CARTESIAN_POINT ( 'NONE',  ( -107.3221550338875687, 22.24192588826928585, 80.00000000000001421 ) ) ;
#9182=CARTESIAN_POINT ( 'NONE',  ( -187.8924994060663494, 156.4650759647683742, -13.00000000000000000 ) ) ;
#9189=EDGE_CURVE ( 'NONE', #20219, #8776, #18106, .T. ) ;
#9191=EDGE_CURVE ( 'NONE', #5762, #1390, #23516, .T. ) ;
#9192=CARTESIAN_POINT ( 'NONE',  ( -7.763489797328277930, 131.2264966167943498, 16.31092294497945971 ) ) ;
#9193=LINE ( 'NONE', #26701, #438 ) ;
#9198=CARTESIAN_POINT ( 'NONE',  ( -212.2922668275968192, 87.25497565882355389, -23.57411103248302453 ) ) ;
#9202=ORIENTED_EDGE ( 'NONE', *, *, #16273, .F. ) ;
#9203=EDGE_LOOP ( 'NONE', ( #15426, #22675 ) ) ;
#9204=CARTESIAN_POINT ( 'NONE',  ( 139.9999999999999147, 4.857225732735056078E-14, 70.00000000000001421 ) ) ;
#9205=AXIS2_PLACEMENT_3D ( 'NONE', #4493, #6800, #17437 ) ;
#9206=CARTESIAN_POINT ( 'NONE',  ( -160.0000000000000284, 119.7660240611718763, 22.85081902853006142 ) ) ;
#9207=ORIENTED_EDGE ( 'NONE', *, *, #20903, .F. ) ;
#9210=AXIS2_PLACEMENT_3D ( 'NONE', #27467, #3622, #5788 ) ;
#9211=EDGE_CURVE ( 'NONE', #7931, #17036, #5167, .T. ) ;
#9218=CARTESIAN_POINT ( 'NONE',  ( -200.3909388570902763, 61.22025098964611090, -27.25552298266465456 ) ) ;
#9219=ORIENTED_EDGE ( 'NONE', *, *, #19756, .T. ) ;
#9221=CARTESIAN_POINT ( 'NONE',  ( -190.0000000000000284, 59.99999999999995026, 80.00000000000001421 ) ) ;
#9222=DIRECTION ( 'NONE',  ( 0.000000000000000000, 0.000000000000000000, 1.000000000000000000 ) ) ;
#9228=AXIS2_PLACEMENT_3D ( 'NONE', #10917, #12798, #19250 ) ;
#9230=CARTESIAN_POINT ( 'NONE',  ( -141.6010952119794126, 70.58289405497825442, 82.86345960551251721 ) ) ;
#9238=EDGE_LOOP ( 'NONE', ( #25407, #6747 ) ) ;
#9240=VECTOR ( 'NONE', #7425, 1000.000000000000000 ) ;
#9243=FACE_OUTER_BOUND ( 'NONE', #2549, .T. ) ;
#9250=CARTESIAN_POINT ( 'NONE',  ( 5.594927750205532568, 137.4232256183554171, -15.08939307562826215 ) ) ;
#9257=CARTESIAN_POINT ( 'NONE',  ( -210.7172313291012529, 103.7585653882801182, 5.000000000000002665 ) ) ;
#9261=DIRECTION ( 'NONE',  ( -1.000000000000000000, 0.000000000000000000, 0.000000000000000000 ) ) ;
#9264=CIRCLE ( 'NONE', #22574, 43.76444293738737912 ) ;
#9270=DIRECTION ( 'NONE',  ( -1.000000000000000000, 0.000000000000000000, -0.000000000000000000 ) ) ;
#9271=AXIS2_PLACEMENT_3D ( 'NONE', #26602, #331, #24312 ) ;
#9274=CARTESIAN_POINT ( 'NONE',  ( -124.9781469243919076, 222.2250949724356985, 15.00000000000000000 ) ) ;
#9283=CARTESIAN_POINT ( 'NONE',  ( 106.7420202941122653, 244.4253804639437533, 31.38183343148724092 ) ) ;
#9292=CARTESIAN_POINT ( 'NONE',  ( 139.9999999999999147, 4.857225732735056709E-14, -70.00000000000001421 ) ) ;
#9295=CARTESIAN_POINT ( 'NONE',  ( 8.117852850209610338, 141.5785587194356197, -13.00000000000000000 ) ) ;
#9296=DIRECTION ( 'NONE',  ( -0.5555587585212683477, -0.8314772792026894344, 0.000000000000000000 ) ) ;
#9297=DIRECTION ( 'NONE',  ( 0.000000000000000000, 0.000000000000000000, -1.000000000000000000 ) ) ;
#9299=DIRECTION ( 'NONE',  ( 0.000000000000000000, 0.000000000000000000, 1.000000000000000000 ) ) ;
#9300=EDGE_CURVE ( 'NONE', #21416, #7297, #7475, .T. ) ;
#9303=DIRECTION ( 'NONE',  ( 0.8153095126952284444, -0.5790253867566337309, 0.000000000000000000 ) ) ;
#9309=CARTESIAN_POINT ( 'NONE',  ( 109.5201339680999837, 255.4997179839799060, -37.19466046300052398 ) ) ;
#9311=CARTESIAN_POINT ( 'NONE',  ( 157.4999999999998579, 220.0000000000000284, 90.00000000000002842 ) ) ;
#9312=AXIS2_PLACEMENT_3D ( 'NONE', #8185, #27564, #6026 ) ;
#9315=ORIENTED_EDGE ( 'NONE', *, *, #16567, .F. ) ;
#9317=ORIENTED_EDGE ( 'NONE', *, *, #587, .F. ) ;
#9318=DIRECTION ( 'NONE',  ( -0.000000000000000000, 1.000000000000000000, -0.000000000000000000 ) ) ;
#9321=CARTESIAN_POINT ( 'NONE',  ( -47.47939869681532343, 132.2278273089350762, -14.48490952286894640 ) ) ;
#9325=CARTESIAN_POINT ( 'NONE',  ( -221.9864287755669068, 60.98533040124961246, 21.67821222924225211 ) ) ;
#9326=CARTESIAN_POINT ( 'NONE',  ( -40.40953891503691153, 71.03850157808263077, 99.00000000000000000 ) ) ;
#9331=CARTESIAN_POINT ( 'NONE',  ( -231.3807819610386218, 93.01706144896263595, -12.99999999999997691 ) ) ;
#9335=CARTESIAN_POINT ( 'NONE',  ( 79.99999999999992895, 110.0000000000000000, 70.00000000000001421 ) ) ;
#9336=CARTESIAN_POINT ( 'NONE',  ( -8.816046456736254200, 132.3922476905560472, 15.94591420432834461 ) ) ;
#9337=EDGE_CURVE ( 'NONE', #15531, #17645, #9771, .T. ) ;
#9341=EDGE_LOOP ( 'NONE', ( #2863, #24651, #22659, #15533, #18974 ) ) ;
#9346=ORIENTED_EDGE ( 'NONE', *, *, #11995, .T. ) ;
#9353=CARTESIAN_POINT ( 'NONE',  ( -135.2491457716903653, 129.6667746786781947, 15.43809234620010962 ) ) ;
#9359=DIRECTION ( 'NONE',  ( -1.000000000000000000, 0.000000000000000000, 0.000000000000000000 ) ) ;
#9360=DIRECTION ( 'NONE',  ( 1.000000000000000000, 8.759632170410045475E-15, 0.000000000000000000 ) ) ;
#9363=( BOUNDED_SURFACE ( )  B_SPLINE_SURFACE ( 3, 2, ( 
 ( #4994, #5287, #18509 ),
 ( #27254, #1117, #9321 ),
 ( #7308, #24833, #22820 ),
 ( #14207, #22956, #26976 ),
 ( #22682, #3260, #20374 ),
 ( #20517, #27388, #9886 ),
 ( #7452, #12197, #16222 ),
 ( #14069, #3120, #18644 ),
 ( #7730, #2984, #16498 ),
 ( #25250, #14344, #3404 ),
 ( #11775, #559, #18085 ),
 ( #13787, #22534, #2844 ),
 ( #703, #9472, #18229 ),
 ( #16082, #5143, #6272 ),
 ( #25808, #17049, #23665 ),
 ( #23517, #12758, #14909 ),
 ( #27810, #3970, #6133 ),
 ( #23376, #10168, #1397 ),
 ( #21497, #18927, #3685 ),
 ( #16776, #1815, #28095 ),
 ( #8148, #19343, #21217 ),
 ( #15046, #25665, #10590 ),
 ( #18783, #16911, #12620 ),
 ( #3830, #8438, #1258 ),
 ( #27669, #25528, #14764 ),
 ( #21359, #17192, #25951 ),
 ( #20937, #23803, #1677 ),
 ( #4113, #10447, #10027 ) ),
 .UNSPECIFIED., .F., .F., .F. ) 
 B_SPLINE_SURFACE_WITH_KNOTS ( ( 4, 2, 2, 2, 2, 2, 2, 2, 2, 2, 2, 2, 2, 4 ),
 ( 3, 3 ),
 ( -6.071532165918824830E-18, 0.01498678567651468181, 0.02997357135302937056, 0.04496035702954406105, 0.05245374986780140802, 0.05620044628693007804, 0.05994714270605874806, 0.07493392838257342814, 0.08992071405908812209, 0.09741410689734547601, 0.1049074997356028160, 0.1086541961547314861, 0.1124008925738601561, 0.1198942854121174961 ),
 ( 0.000000000000000000, 1.000000000000000000 ),
 .UNSPECIFIED. ) 
 GEOMETRIC_REPRESENTATION_ITEM ( )  RATIONAL_B_SPLINE_SURFACE ( (
 ( 1.000000000000000000, 0.8161343730438194166, 1.000000000000000000),
 ( 1.000000000000000000, 0.8053590984426869381, 1.000000000000000000),
 ( 1.000000000000000000, 0.7960137040925352458, 1.000000000000000000),
 ( 1.000000000000000000, 0.7808453201752241224, 1.000000000000000000),
 ( 1.000000000000000000, 0.7750273194348902273, 1.000000000000000000),
 ( 1.000000000000000000, 0.7674151632800794154, 1.000000000000000000),
 ( 1.000000000000000000, 0.7656231679750936658, 1.000000000000000000),
 ( 1.000000000000000000, 0.7661290450854815193, 1.000000000000000000),
 ( 1.000000000000000000, 0.7668277142013406600, 1.000000000000000000),
 ( 1.000000000000000000, 0.7686712949395471117, 1.000000000000000000),
 ( 1.000000000000000000, 0.7694194103377227645, 1.000000000000000000),
 ( 1.000000000000000000, 0.7711707737263995277, 1.000000000000000000),
 ( 1.000000000000000000, 0.7721740736493929447, 1.000000000000000000),
 ( 1.000000000000000000, 0.7778076735771930483, 1.000000000000000000),
 ( 1.000000000000000000, 0.7842969395606893546, 1.000000000000000000),
 ( 1.000000000000000000, 0.8005680270097221829, 1.000000000000000000),
 ( 1.000000000000000000, 0.8103469025248568602, 1.000000000000000000),
 ( 1.000000000000000000, 0.8268680461880919541, 1.000000000000000000),
 ( 1.000000000000000000, 0.8326830769007559363, 1.000000000000000000),
 ( 1.000000000000000000, 0.8448194715605038541, 1.000000000000000000),
 ( 1.000000000000000000, 0.8511408365003451104, 1.000000000000000000),
 ( 1.000000000000000000, 0.8609175397525088425, 1.000000000000000000),
 ( 1.000000000000000000, 0.8642255213344454123, 1.000000000000000000),
 ( 1.000000000000000000, 0.8709250352162014597, 1.000000000000000000),
 ( 1.000000000000000000, 0.8743096907132095197, 1.000000000000000000),
 ( 1.000000000000000000, 0.8844861762812324946, 1.000000000000000000),
 ( 1.000000000000000000, 0.8913208799372495106, 1.000000000000000000),
 ( 1.000000000000000000, 0.8981184559478653240, 1.000000000000000000) ) ) 
 REPRESENTATION_ITEM ( '' )  SURFACE ( )  );
#9364=DIRECTION ( 'NONE',  ( 1.000000000000000000, 0.000000000000000000, 0.000000000000000000 ) ) ;
#9367=DIRECTION ( 'NONE',  ( 1.000000000000000000, 1.530283246943720875E-16, 0.000000000000000000 ) ) ;
#9368=CARTESIAN_POINT ( 'NONE',  ( -215.3445465745174658, 71.74628434702670177, -26.24848034640785954 ) ) ;
#9369=AXIS2_PLACEMENT_3D ( 'NONE', #6592, #6448, #25984 ) ;
#9371=DIRECTION ( 'NONE',  ( -1.000000000000000000, -1.530283246943720875E-16, 0.000000000000000000 ) ) ;
#9372=CARTESIAN_POINT ( 'NONE',  ( -215.4886702565632675, 139.8420026707765942, -15.00000000000000178 ) ) ;
#9373=DIRECTION ( 'NONE',  ( 1.000000000000000000, 0.000000000000000000, 0.000000000000000000 ) ) ;
#9379=EDGE_CURVE ( 'NONE', #8966, #6472, #4233, .T. ) ;
#9380=CYLINDRICAL_SURFACE ( 'NONE', #13959, 2.586968381275096984 ) ;
#9382=VERTEX_POINT ( 'NONE', #22838 ) ;
#9384=CARTESIAN_POINT ( 'NONE',  ( 108.2273028577272385, 129.5338070839680711, 99.99999999997838529 ) ) ;
#9388=ORIENTED_EDGE ( 'NONE', *, *, #22266, .T. ) ;
#9390=DIRECTION ( 'NONE',  ( 1.000000000000000000, 0.000000000000000000, 0.000000000000000000 ) ) ;
#9396=CARTESIAN_POINT ( 'NONE',  ( 145.9999999999998863, 220.0000000000000284, 100.0000000000000142 ) ) ;
#9399=ADVANCED_FACE ( 'NONE', ( #22701 ), #4390, .T. ) ;
#9401=CARTESIAN_POINT ( 'NONE',  ( -5.362442292600443139, 133.6996795038672587, -14.05115172523858469 ) ) ;
#9402=LINE ( 'NONE', #22466, #9990 ) ;
#9404=DIRECTION ( 'NONE',  ( -0.000000000000000000, -0.000000000000000000, 1.000000000000000000 ) ) ;
#9405=ORIENTED_EDGE ( 'NONE', *, *, #23823, .T. ) ;
#9407=DIRECTION ( 'NONE',  ( 1.040834085586083310E-14, 0.000000000000000000, 1.000000000000000000 ) ) ;
#9408=DIRECTION ( 'NONE',  ( 0.8018642810807392607, 0.5975062131282562472, 0.000000000000000000 ) ) ;
#9412=CARTESIAN_POINT ( 'NONE',  ( -243.4285414610288001, 74.63108012613848530, 5.000000000000001776 ) ) ;
#9413=ORIENTED_EDGE ( 'NONE', *, *, #22140, .T. ) ;
#9415=CARTESIAN_POINT ( 'NONE',  ( -234.1469129038715096, 66.78385994367806688, -6.149209796590396238 ) ) ;
#9419=FACE_OUTER_BOUND ( 'NONE', #18110, .T. ) ;
#9423=CARTESIAN_POINT ( 'NONE',  ( -43.02437977270766822, 129.7200458115292747, 16.81627168235289815 ) ) ;
#9425=DIRECTION ( 'NONE',  ( 8.659560562354934091E-17, 0.7071067811865474617, -0.7071067811865476838 ) ) ;
#9430=VECTOR ( 'NONE', #5813, 1000.000000000000000 ) ;
#9431=VERTEX_POINT ( 'NONE', #26254 ) ;
#9435=CARTESIAN_POINT ( 'NONE',  ( 96.29556199549340079, 241.0127520899143576, 10.03785181564020235 ) ) ;
#9437=CARTESIAN_POINT ( 'NONE',  ( -42.99650729631200363, 36.92584315232891612, 100.0000000000000000 ) ) ;
#9438=CARTESIAN_POINT ( 'NONE',  ( -56.48697296830715686, 1.968917815184006985E-15, 99.00000000000000000 ) ) ;
#9439=VECTOR ( 'NONE', #5616, 1000.000000000000000 ) ;
#9440=CARTESIAN_POINT ( 'NONE',  ( 100.5794065449870942, 118.1137289701970872, -81.24999999966573228 ) ) ;
#9443=LINE ( 'NONE', #3093, #7197 ) ;
#9447=CARTESIAN_POINT ( 'NONE',  ( -180.0000000000000284, -70.00000000000004263, -25.00000000000000000 ) ) ;
#9451=CARTESIAN_POINT ( 'NONE',  ( -17.24491960465746132, 75.97823757117562593, 100.0000000000000000 ) ) ;
#9452=DIRECTION ( 'NONE',  ( -1.000000000000000000, 0.000000000000000000, 0.000000000000000000 ) ) ;
#9457=CARTESIAN_POINT ( 'NONE',  ( 109.9999999999998863, 260.0000000000000000, -45.00000000000000000 ) ) ;
#9459=EDGE_CURVE ( 'NONE', #19265, #24488, #11327, .T. ) ;
#9463=EDGE_LOOP ( 'NONE', ( #12843, #12665, #24220 ) ) ;
#9472=CARTESIAN_POINT ( 'NONE',  ( -101.6427404889548711, 135.8129376563426831, -15.24817990273632340 ) ) ;
#9473=AXIS2_PLACEMENT_3D ( 'NONE', #21984, #8635, #17390 ) ;
#9474=DIRECTION ( 'NONE',  ( 1.000000000000000000, 0.000000000000000000, 0.000000000000000000 ) ) ;
#9475=CARTESIAN_POINT ( 'NONE',  ( -213.2464434226970980, 57.29534669709770611, 37.98348409338887421 ) ) ;
#9477=CARTESIAN_POINT ( 'NONE',  ( -42.53273978471831640, 130.9733465240572627, -14.93735646117640492 ) ) ;
#9478=CARTESIAN_POINT ( 'NONE',  ( -63.57415822541634043, 24.64876300893806160, 95.00000000000000000 ) ) ;
#9479=CARTESIAN_POINT ( 'NONE',  ( -225.7503879793210899, 89.48004551377478322, -13.96212495524699015 ) ) ;
#9480=AXIS2_PLACEMENT_3D ( 'NONE', #19173, #27643, #1649 ) ;
#9483=CARTESIAN_POINT ( 'NONE',  ( 105.2480867101079980, 123.6573351780392613, 85.93750000029402258 ) ) ;
#9484=CARTESIAN_POINT ( 'NONE',  ( -23.59768067310782413, 129.3237483323889592, 16.93303552989647898 ) ) ;
#9487=CARTESIAN_POINT ( 'NONE',  ( -63.57415822541634043, -23.01420295945612082, 80.00000000000001421 ) ) ;
#9489=ORIENTED_EDGE ( 'NONE', *, *, #23404, .T. ) ;
#9491=DIRECTION ( 'NONE',  ( -1.000000000000000000, -1.321694076934710155E-16, 0.000000000000000000 ) ) ;
#9492=EDGE_LOOP ( 'NONE', ( #8909, #6266, #7414, #3533 ) ) ;
#9495=ADVANCED_FACE ( 'NONE', ( #15497 ), #18494, .F. ) ;
#9498=CARTESIAN_POINT ( 'NONE',  ( -138.3093778148924571, 127.5098211573111087, 17.72095338322215952 ) ) ;
#9502=PLANE ( 'NONE',  #3992 ) ;
#9503=EDGE_CURVE ( 'NONE', #20254, #15707, #16654, .T. ) ;
#9506=CARTESIAN_POINT ( 'NONE',  ( 89.55287500703019532, 230.0961521423384113, -16.54242257938075156 ) ) ;
#9510=CIRCLE ( 'NONE', #11811, 39.99999999999999289 ) ;
#9511=CARTESIAN_POINT ( 'NONE',  ( -194.7277720219268815, 63.01928361507884091, -39.96465835449415493 ) ) ;
#9512=AXIS2_PLACEMENT_3D ( 'NONE', #18079, #7304, #20792 ) ;
#9513=DIRECTION ( 'NONE',  ( -1.000000000000000000, 0.000000000000000000, 0.000000000000000000 ) ) ;
#9519=CARTESIAN_POINT ( 'NONE',  ( -243.5753208290495309, 74.80993601160373885, 14.84129168367922702 ) ) ;
#9520=CARTESIAN_POINT ( 'NONE',  ( -160.0000000000000568, 90.00000000000001421, 98.28427124746191623 ) ) ;
#9521=EDGE_LOOP ( 'NONE', ( #18846, #11506, #521, #4057 ) ) ;
#9524=CARTESIAN_POINT ( 'NONE',  ( 90.17595424772805757, 111.7661400908348384, 72.22656249985354293 ) ) ;
#9525=CARTESIAN_POINT ( 'NONE',  ( -202.5288808976002599, 93.61334720101866935, -29.67947843847759870 ) ) ;
#9526=ORIENTED_EDGE ( 'NONE', *, *, #10051, .T. ) ;
#9529=DIRECTION ( 'NONE',  ( 0.000000000000000000, -1.000000000000000000, 0.000000000000000000 ) ) ;
#9532=ORIENTED_EDGE ( 'NONE', *, *, #10332, .F. ) ;
#9540=CARTESIAN_POINT ( 'NONE',  ( -25.32102446532049811, 128.0228448628550098, -17.49457884177929046 ) ) ;
#9543=CARTESIAN_POINT ( 'NONE',  ( -196.7918453702777128, 68.51688903468615877, 83.00000000000001421 ) ) ;
#9545=VERTEX_POINT ( 'NONE', #14469 ) ;
#9556=CARTESIAN_POINT ( 'NONE',  ( 134.9999999999998579, 220.0000000000000284, 99.00000000000001421 ) ) ;
#9558=ORIENTED_EDGE ( 'NONE', *, *, #1241, .F. ) ;
#9562=CARTESIAN_POINT ( 'NONE',  ( 89.99999999999994316, -90.00000000000001421, 100.0000000000000142 ) ) ;
#9566=ORIENTED_EDGE ( 'NONE', *, *, #28214, .F. ) ;
#9568=ORIENTED_EDGE ( 'NONE', *, *, #6042, .F. ) ;
#9569=CONICAL_SURFACE ( 'NONE', #8649, 21.20097097723064294, 0.08885387018394180769 ) ;
#9571=ORIENTED_EDGE ( 'NONE', *, *, #27885, .F. ) ;
#9572=ORIENTED_EDGE ( 'NONE', *, *, #5425, .T. ) ;
#9573=CARTESIAN_POINT ( 'NONE',  ( 109.9760533923134744, 258.8696700914142070, 43.04221176963723394 ) ) ;
#9576=CARTESIAN_POINT ( 'NONE',  ( -175.0000000000000000, -120.0000000000001847, -63.97499999999998721 ) ) ;
#9577=CARTESIAN_POINT ( 'NONE',  ( 134.9999999999998579, 220.0000000000000284, -100.0000000000000142 ) ) ;
#9582=CARTESIAN_POINT ( 'NONE',  ( -156.8436863811591593, 180.7779002010535692, -13.00000000000000000 ) ) ;
#9595=LINE ( 'NONE', #18215, #12088 ) ;
#9599=ORIENTED_EDGE ( 'NONE', *, *, #8931, .T. ) ;
#9603=ORIENTED_EDGE ( 'NONE', *, *, #14198, .F. ) ;
#9604=CARTESIAN_POINT ( 'NONE',  ( -108.0099734903331807, 135.2217844244274545, 13.71957698657085345 ) ) ;
#9606=DIRECTION ( 'NONE',  ( 0.000000000000000000, 0.000000000000000000, 1.000000000000000000 ) ) ;
#9607=CIRCLE ( 'NONE', #4516, 6.204828372381208546 ) ;
#9609=CARTESIAN_POINT ( 'NONE',  ( -27.00683456900459234, 129.1643779576224063, 15.68707256237481928 ) ) ;
#9610=AXIS2_PLACEMENT_3D ( 'NONE', #23696, #27702, #17081 ) ;
#9611=CARTESIAN_POINT ( 'NONE',  ( -194.6040764069587112, 63.06822542404761123, 40.63350569893458442 ) ) ;
#9612=DIRECTION ( 'NONE',  ( 0.000000000000000000, 0.000000000000000000, 1.000000000000000000 ) ) ;
#9615=CARTESIAN_POINT ( 'NONE',  ( 79.99999999999994316, 108.4677831376940560, -79.66646975086558768 ) ) ;
#9616=CARTESIAN_POINT ( 'NONE',  ( -221.7152077904632677, 88.25158514949524147, -15.54860131211836993 ) ) ;
#9617=CARTESIAN_POINT ( 'NONE',  ( 134.9999999999998579, 220.0000000000000284, 99.00000000000001421 ) ) ;
#9619=CARTESIAN_POINT ( 'NONE',  ( 33.10302365956999182, 203.2034914284457159, 15.00000000000000000 ) ) ;
#9621=CIRCLE ( 'NONE', #6836, 22.49999999999999289 ) ;
#9629=EDGE_CURVE ( 'NONE', #6895, #14227, #9595, .T. ) ;
#9630=AXIS2_PLACEMENT_3D ( 'NONE', #21969, #17512, #15664 ) ;
#9631=CARTESIAN_POINT ( 'NONE',  ( 90.00000000000024158, 240.0000000000000284, -6.270166537925966566 ) ) ;
#9632=EDGE_CURVE ( 'NONE', #11042, #13747, #18358, .T. ) ;
#9635=ORIENTED_EDGE ( 'NONE', *, *, #20310, .T. ) ;
#9642=CIRCLE ( 'NONE', #17433, 5.999999999999991118 ) ;
#9644=CARTESIAN_POINT ( 'NONE',  ( 91.50132543202619217, 230.4711603839584768, -17.28742811890413478 ) ) ;
#9645=AXIS2_PLACEMENT_3D ( 'NONE', #27236, #3385, #16343 ) ;
#9647=CYLINDRICAL_SURFACE ( 'NONE', #11441, 9.999999999999994671 ) ;
#9648=CARTESIAN_POINT ( 'NONE',  ( -213.2464434226970980, 57.29534669709769901, -37.98348409338405673 ) ) ;
#9649=ADVANCED_FACE ( 'NONE', ( #19476 ), #6401, .T. ) ;
#9652=DIRECTION ( 'NONE',  ( -0.000000000000000000, 0.000000000000000000, 1.000000000000000000 ) ) ;
#9660=FACE_OUTER_BOUND ( 'NONE', #22524, .T. ) ;
#9661=LINE ( 'NONE', #25438, #23207 ) ;
#9663=ORIENTED_EDGE ( 'NONE', *, *, #8884, .F. ) ;
#9665=CARTESIAN_POINT ( 'NONE',  ( 109.5756401952765486, 134.3783162856070703, 89.68749999971406339 ) ) ;
#9669=CARTESIAN_POINT ( 'NONE',  ( -76.25760768171835480, 219.6666220619077876, 12.99999999999999822 ) ) ;
#9670=FACE_OUTER_BOUND ( 'NONE', #6442, .T. ) ;
#9672=ORIENTED_EDGE ( 'NONE', *, *, #25535, .T. ) ;
#9677=CARTESIAN_POINT ( 'NONE',  ( -71.37541315349507443, 230.0000000000000000, -15.00000000000000000 ) ) ;
#9679=CARTESIAN_POINT ( 'NONE',  ( 0.8309465671043746449, 136.6869851649963721, -15.12344959194870420 ) ) ;
#9681=CARTESIAN_POINT ( 'NONE',  ( -214.3828916364065833, 175.2783111443768576, 12.99999999999999822 ) ) ;
#9691=CARTESIAN_POINT ( 'NONE',  ( -189.8086322075389774, 92.49158130768422836, 15.00000000000000000 ) ) ;
#9692=DIRECTION ( 'NONE',  ( 0.8314772792026894344, -0.5555587585212683477, 0.000000000000000000 ) ) ;
#9694=ORIENTED_EDGE ( 'NONE', *, *, #11480, .F. ) ;
#9701=CARTESIAN_POINT ( 'NONE',  ( 99.17402272717502854, 242.2128782075101867, 12.79878931498954486 ) ) ;
#9704=CARTESIAN_POINT ( 'NONE',  ( -160.0000000000000284, 119.7660240611718905, -22.85081902853004721 ) ) ;
#9707=EDGE_LOOP ( 'NONE', ( #10395, #6543, #8600, #17322 ) ) ;
#9710=CARTESIAN_POINT ( 'NONE',  ( 107.9865739111272944, 251.1735473298315355, 29.61538987307772430 ) ) ;
#9720=DIRECTION ( 'NONE',  ( 0.000000000000000000, 0.000000000000000000, 1.000000000000000000 ) ) ;
#9723=DIRECTION ( 'NONE',  ( 0.000000000000000000, 0.7071067811865476838, 0.7071067811865474617 ) ) ;
#9727=AXIS2_PLACEMENT_3D ( 'NONE', #27542, #18658, #5582 ) ;
#9730=DIRECTION ( 'NONE',  ( 0.000000000000000000, -0.000000000000000000, -1.000000000000000000 ) ) ;
#9731=ORIENTED_EDGE ( 'NONE', *, *, #18839, .F. ) ;
#9733=ADVANCED_FACE ( 'NONE', ( #17180 ), #19331, .T. ) ;
#9738=CIRCLE ( 'NONE', #20736, 10.00000000000000888 ) ;
#9743=LINE ( 'NONE', #26836, #20974 ) ;
#9747=CIRCLE ( 'NONE', #11109, 11.00000000000001066 ) ;
#9748=FACE_OUTER_BOUND ( 'NONE', #27517, .T. ) ;
#9750=EDGE_CURVE ( 'NONE', #8949, #14118, #4586, .T. ) ;
#9753=CARTESIAN_POINT ( 'NONE',  ( -214.1728591254723142, 55.16903133821974592, 44.30008786503535845 ) ) ;
#9760=CARTESIAN_POINT ( 'NONE',  ( -146.6428522700808230, 74.54464929955099706, 83.00000000000001421 ) ) ;
#9761=CARTESIAN_POINT ( 'NONE',  ( 134.9999999999998579, 220.0000000000000284, 153.1081322850112940 ) ) ;
#9765=CARTESIAN_POINT ( 'NONE',  ( 114.5273445118729541, 107.2595481030940761, -100.0000000000000142 ) ) ;
#9766=CARTESIAN_POINT ( 'NONE',  ( 157.4999999999998579, 220.0000000000000284, -84.99999999999997158 ) ) ;
#9771=LINE ( 'NONE', #18528, #12514 ) ;
#9772=B_SPLINE_CURVE_WITH_KNOTS ( 'NONE', 3,
 ( #291, #7180, #2860, #9047, #26283, #15384, #17950, #6604, #15951, #24138, #22695, #11791, #1130, #24986, #23115, #7325, #5302, #1271, #22972, #2999, #27133, #25405 ),
 .UNSPECIFIED., .F., .F.,
 ( 4, 2, 2, 2, 2, 2, 2, 2, 2, 2, 4 ),
 ( 0.000000000000000000, 0.006670623320370424290, 0.01334124664074084858, 0.02001186996111127200, 0.02334718162129648458, 0.02668249328148169716, 0.03335311660185202171, 0.03668842826203719265, 0.04002373992222235666, 0.04669436324259268467, 0.05336498656296301268 ),
 .UNSPECIFIED. ) ;
#9775=ORIENTED_EDGE ( 'NONE', *, *, #6970, .T. ) ;
#9778=TOROIDAL_SURFACE ( 'NONE', #7939, 55.86582179324592090, 2.000000000000000000 ) ;
#9782=AXIS2_PLACEMENT_3D ( 'NONE', #4301, #17369, #10485 ) ;
#9784=EDGE_CURVE ( 'NONE', #12221, #4097, #10861, .T. ) ;
#9787=DIRECTION ( 'NONE',  ( 1.000000000000000000, -8.220356446306165096E-16, 0.000000000000000000 ) ) ;
#9788=CARTESIAN_POINT ( 'NONE',  ( 79.99999999999992895, 110.0000000000000000, -100.0000000000000142 ) ) ;
#9789=CARTESIAN_POINT ( 'NONE',  ( 124.9999999999998579, 220.0000000000000284, -99.00000000000001421 ) ) ;
#9790=CARTESIAN_POINT ( 'NONE',  ( -210.1614673636062207, 73.84361952687928010, -34.09424755233946769 ) ) ;
#9794=EDGE_LOOP ( 'NONE', ( #13265, #2660, #11041, #25973, #3166, #21702 ) ) ;
#9797=CIRCLE ( 'NONE', #25378, 6.000000000000005329 ) ;
#9798=CARTESIAN_POINT ( 'NONE',  ( -228.6046226639666088, 73.96500373646588855, 16.69423931604977085 ) ) ;
#9801=AXIS2_PLACEMENT_3D ( 'NONE', #14596, #18619, #18348 ) ;
#9802=ORIENTED_EDGE ( 'NONE', *, *, #1014, .F. ) ;
#9803=CARTESIAN_POINT ( 'NONE',  ( 100.5794065448834402, 118.1137289702941047, 99.99999999995674216 ) ) ;
#9806=ORIENTED_EDGE ( 'NONE', *, *, #25316, .F. ) ;
#9810=VERTEX_POINT ( 'NONE', #11004 ) ;
#9812=EDGE_LOOP ( 'NONE', ( #7523, #19041, #21817, #15429 ) ) ;
#9814=CARTESIAN_POINT ( 'NONE',  ( -76.25760768171836901, 154.8982798170083299, -13.00000000000000000 ) ) ;
#9821=CARTESIAN_POINT ( 'NONE',  ( -210.0000000000000284, 59.99999999999993605, 70.00000000000000000 ) ) ;
#9824=ORIENTED_EDGE ( 'NONE', *, *, #2428, .F. ) ;
#9826=CARTESIAN_POINT ( 'NONE',  ( -63.57415822541634043, 0.000000000000000000, 100.0000000000000000 ) ) ;
#9831=DIRECTION ( 'NONE',  ( 0.000000000000000000, 0.000000000000000000, 1.000000000000000000 ) ) ;
#9832=DIRECTION ( 'NONE',  ( 0.5555587585212683477, 0.8314772792026894344, 0.000000000000000000 ) ) ;
#9836=CARTESIAN_POINT ( 'NONE',  ( -210.0000000000000284, 59.99999999999993605, 100.0000000000000142 ) ) ;
#9839=CARTESIAN_POINT ( 'NONE',  ( -112.5534411697180559, 133.0508595578523909, 15.80357080798902913 ) ) ;
#9842=AXIS2_PLACEMENT_3D ( 'NONE', #11683, #7636, #21375 ) ;
#9845=ORIENTED_EDGE ( 'NONE', *, *, #21025, .T. ) ;
#9851=LINE ( 'NONE', #18049, #25910 ) ;
#9852=CARTESIAN_POINT ( 'NONE',  ( -216.4421519707229891, 141.6000904446840707, -15.00000000000000000 ) ) ;
#9853=AXIS2_PLACEMENT_3D ( 'NONE', #8506, #12406, #6339 ) ;
#9854=DIRECTION ( 'NONE',  ( 0.000000000000000000, 1.000000000000000000, -1.224646799147353207E-16 ) ) ;
#9857=ADVANCED_FACE ( 'NONE', ( #4945 ), #6963, .F. ) ;
#9858=CARTESIAN_POINT ( 'NONE',  ( -219.2467648448761395, 139.5102435001769265, -15.00000000000000000 ) ) ;
#9863=VERTEX_POINT ( 'NONE', #19615 ) ;
#9866=DIRECTION ( 'NONE',  ( 0.8018642810807398158, 0.5975062131282554700, -0.000000000000000000 ) ) ;
#9877=EDGE_CURVE ( 'NONE', #14406, #23088, #26936, .T. ) ;
#9878=ORIENTED_EDGE ( 'NONE', *, *, #9337, .F. ) ;
#9879=ORIENTED_EDGE ( 'NONE', *, *, #8445, .T. ) ;
#9880=VECTOR ( 'NONE', #10820, 1000.000000000000000 ) ;
#9883=CARTESIAN_POINT ( 'NONE',  ( 89.99999999999994316, -90.00000000000001421, -70.00000000000001421 ) ) ;
#9886=CARTESIAN_POINT ( 'NONE',  ( -77.52803642472932211, 136.3040012171963156, -13.50820732054850559 ) ) ;
#9890=CARTESIAN_POINT ( 'NONE',  ( -90.19911340583169590, 136.4341784506709416, -13.48770749977458294 ) ) ;
#9892=ADVANCED_FACE ( 'NONE', ( #796 ), #3075, .F. ) ;
#9895=CARTESIAN_POINT ( 'NONE',  ( -208.4641541919228871, 89.68079096126031402, -24.78256666906890260 ) ) ;
#9897=DIRECTION ( 'NONE',  ( 1.000000000000000000, 0.000000000000000000, 0.000000000000000000 ) ) ;
#9901=ORIENTED_EDGE ( 'NONE', *, *, #16934, .T. ) ;
#9905=AXIS2_PLACEMENT_3D ( 'NONE', #12523, #16823, #25713 ) ;
#9907=ORIENTED_EDGE ( 'NONE', *, *, #21024, .F. ) ;
#9915=AXIS2_PLACEMENT_3D ( 'NONE', #2135, #13646, #8896 ) ;
#9916=ADVANCED_FACE ( 'NONE', ( #656 ), #16316, .T. ) ;
#9917=EDGE_LOOP ( 'NONE', ( #3313, #5200, #10711, #4137 ) ) ;
#9918=LINE ( 'NONE', #22711, #5252 ) ;
#9920=DIRECTION ( 'NONE',  ( 1.000000000000000000, 0.000000000000000000, 0.000000000000000000 ) ) ;
#9922=CARTESIAN_POINT ( 'NONE',  ( 101.6154897312858338, 236.6169605195232748, -24.18002435645406933 ) ) ;
#9923=CARTESIAN_POINT ( 'NONE',  ( -4.730967070951327180, 132.3085785638695029, -15.99979783535312983 ) ) ;
#9924=CARTESIAN_POINT ( 'NONE',  ( -112.3221550338875687, 69.54464929955099706, 83.00000000000001421 ) ) ;
#9926=DIRECTION ( 'NONE',  ( -0.000000000000000000, 0.000000000000000000, 1.000000000000000000 ) ) ;
#9934=DIRECTION ( 'NONE',  ( 0.2759800118297804916, -0.9611633748070274041, 0.000000000000000000 ) ) ;
#9937=AXIS2_PLACEMENT_3D ( 'NONE', #16054, #25084, #5399 ) ;
#9940=EDGE_CURVE ( 'NONE', #11012, #1342, #28043, .T. ) ;
#9944=ORIENTED_EDGE ( 'NONE', *, *, #7790, .F. ) ;
#9945=CARTESIAN_POINT ( 'NONE',  ( 79.99999999999991473, 110.0000000000000142, -70.00000000000001421 ) ) ;
#9946=CARTESIAN_POINT ( 'NONE',  ( 93.83231682052215206, 231.2056562043867984, 18.37428548869055334 ) ) ;
#9949=CARTESIAN_POINT ( 'NONE',  ( -229.6754219177769301, 91.64948492225875043, 13.10942810910360912 ) ) ;
#9951=TOROIDAL_SURFACE ( 'NONE', #3522, 421.5408555545579929, 7.500000000000000000 ) ;
#9952=CARTESIAN_POINT ( 'NONE',  ( 1.982541115402066017E-14, -150.0000000000000568, 100.0000000000000142 ) ) ;
#9956=CARTESIAN_POINT ( 'NONE',  ( 9.999999999999964473, 60.00000000000001421, 100.0000000000000142 ) ) ;
#9962=CARTESIAN_POINT ( 'NONE',  ( -141.6428522700808230, 74.54464929955099706, 80.00000000000001421 ) ) ;
#9965=ORIENTED_EDGE ( 'NONE', *, *, #4707, .F. ) ;
#9973=CARTESIAN_POINT ( 'NONE',  ( -214.3828916364065833, 175.2783111443768576, 12.99999999999999822 ) ) ;
#9976=AXIS2_PLACEMENT_3D ( 'NONE', #13527, #593, #9359 ) ;
#9978=CLOSED_SHELL ( 'NONE', ( #17937, #4050, #22931, #20228, #12190, #8509, #15540, #6627, #22494, #285, #9013, #24267, #3043, #20483, #8414, #9176, #8514, #23375, #4547, #6599, #987, #11583, #23139, #4947, #3760, #15991, #1107, #13447, #10050, #26765, #22461, #11078, #337, #14552, #14911, #8901, #27154, #9857, #15585, #10765, #5948, #1745, #702, #2298, #19718, #9495, #26359, #21373, #17581, #6417, #227, #15520, #12453, #7798, #12701, #7381, #13819, #24647, #5905, #27985, #8902, #1249, #13968, #26687, #25756, #27054, #1678, #1501, #22228, #6630, #4331, #21732, #15108, #13319, #18251, #937, #1045, #22388, #7513, #1275, #14798, #13015, #3563, #26691, #10788, #10686, #21776, #4128, #5421, #11453, #10730, #21407, #5874, #2879, #6784, #20831, #16067, #19048, #132, #12123, #5680, #17432, #14383, #24590, #4188, #14717, #17047, #5310, #12347, #22553, #21463, #19985, #15231, #23072, #4927, #18630, #26116, #23663, #17100, #22818, #443, #27380, #26367, #23694, #20867, #5529, #2854, #10486, #26594, #9064, #6169, #7119, #23252, #10776, #5573, #18689, #9892, #10632, #21656, #19669, #7776, #22822, #9916, #8620, #17514, #27344, #12930, #25317, #10389, #4148, #11131, #10966, #14467, #14437, #17327, #15682, #24723, #9399, #21064, #10720, #15095, #21223, #17003, #20766, #21870, #4749, #8256, #9, #7320, #5067, #6858, #4896, #16386, #7710, #13394, #26380, #14206, #20690, #1219, #14052, #25211, #1504, #5102, #15958, #14963, #25687, #14428, #16924, #20040, #27684, #20028, #24360, #11448, #22067, #18129, #310, #27260, #16594, #5656, #10852, #19716, #14506, #13283, #19822, #15952, #19905, #1143, #14638, #21187, #20241, #8476, #12786, #23851, #26332, #960, #20701, #19301, #2239, #10688, #14971, #22292, #10459, #18487, #21667, #27466, #22855, #3765, #17963, #6750, #673, #16641, #13312, #21027, #7269, #13223, #28256, #3370, #25242, #5557, #9649, #23664, #2967, #26429, #13168, #6523, #1046, #14712, #27261, #9733, #10589, #2761, #20691, #23013, #19881, #11342 ) ) ;
#9979=EDGE_CURVE ( 'NONE', #18699, #22168, #22101, .T. ) ;
#9982=CARTESIAN_POINT ( 'NONE',  ( 109.9934396465123001, 259.4709655040182383, 44.08366846580944554 ) ) ;
#9983=ORIENTED_EDGE ( 'NONE', *, *, #16942, .F. ) ;
#9985=DIRECTION ( 'NONE',  ( 1.000000000000000000, -0.000000000000000000, -0.000000000000000000 ) ) ;
#9990=VECTOR ( 'NONE', #26916, 1000.000000000000000 ) ;
#9991=CARTESIAN_POINT ( 'NONE',  ( -221.3650667873343139, -91.18033988749901653, 0.000000000000000000 ) ) ;
#9992=LINE ( 'NONE', #23065, #24306 ) ;
#9993=AXIS2_PLACEMENT_3D ( 'NONE', #26535, #20224, #556 ) ;
#9995=CARTESIAN_POINT ( 'NONE',  ( 116.8899838958981974, 206.6356889813898192, -99.51050955275447052 ) ) ;
#9997=CARTESIAN_POINT ( 'NONE',  ( 134.9999999999998579, -327.2004514666934369, 84.99999999999995737 ) ) ;
#9998=CARTESIAN_POINT ( 'NONE',  ( -205.7061355896894383, 146.0477147645469813, 15.00000000000000000 ) ) ;
#10003=CARTESIAN_POINT ( 'NONE',  ( -20.30805539402063431, 129.6344908925467223, 15.47809640394222086 ) ) ;
#10006=CARTESIAN_POINT ( 'NONE',  ( 100.4596362579077464, 242.9371632374793819, -14.31520527065961979 ) ) ;
#10009=CARTESIAN_POINT ( 'NONE',  ( -217.2892621185082760, 109.4029876883478352, -13.00000000000000000 ) ) ;
#10013=ORIENTED_EDGE ( 'NONE', *, *, #10296, .T. ) ;
#10017=VERTEX_POINT ( 'NONE', #17143 ) ;
#10026=AXIS2_PLACEMENT_3D ( 'NONE', #15068, #1980, #10757 ) ;
#10027=CARTESIAN_POINT ( 'NONE',  ( -160.8326600028555617, 120.2355194873574931, -21.37420696376538132 ) ) ;
#10028=CARTESIAN_POINT ( 'NONE',  ( -214.3828916364065833, 175.2783111443768576, 15.00000000000000000 ) ) ;
#10029=TOROIDAL_SURFACE ( 'NONE', #17359, 55.86582179324592090, 2.000000000000000000 ) ;
#10031=CARTESIAN_POINT ( 'NONE',  ( -135.1351637729545700, 129.7127537419684700, -15.41371473069906095 ) ) ;
#10034=CARTESIAN_POINT ( 'NONE',  ( -175.0000000000000000, -120.0000000000001705, 64.00000000000002842 ) ) ;
#10036=DIRECTION ( 'NONE',  ( 1.000000000000000000, 0.000000000000000000, 0.000000000000000000 ) ) ;
#10039=EDGE_CURVE ( 'NONE', #4814, #24608, #1491, .T. ) ;
#10040=DIRECTION ( 'NONE',  ( 0.000000000000000000, -2.498359269027536321E-16, 1.000000000000000000 ) ) ;
#10047=ORIENTED_EDGE ( 'NONE', *, *, #5128, .F. ) ;
#10049=VECTOR ( 'NONE', #15450, 1000.000000000000000 ) ;
#10050=ADVANCED_FACE ( 'NONE', ( #19019 ), #19296, .F. ) ;
#10051=EDGE_CURVE ( 'NONE', #26218, #26681, #12025, .T. ) ;
#10052=AXIS2_PLACEMENT_3D ( 'NONE', #9956, #21429, #23731 ) ;
#10054=ORIENTED_EDGE ( 'NONE', *, *, #26503, .F. ) ;
#10055=EDGE_LOOP ( 'NONE', ( #20715, #16848, #11184, #27883, #3396, #9731, #7586, #24652 ) ) ;
#10058=DIRECTION ( 'NONE',  ( 1.000000000000000000, 0.000000000000000000, 0.000000000000000000 ) ) ;
#10065=B_SPLINE_CURVE_WITH_KNOTS ( 'NONE', 3,
 ( #11643, #14214, #16091, #27263, #13648, #7172, #848, #9895, #22964, #15946, #5294, #24696, #2708, #3267, #18651, #12059, #24551, #14077, #9616, #5003, #4860, #9479, #22828, #13796, #11496, #20662, #566, #16368, #9331, #22543 ),
 .UNSPECIFIED., .F., .F.,
 ( 4, 2, 2, 2, 2, 2, 2, 2, 2, 2, 2, 2, 2, 2, 4 ),
 ( 3.469446951953614189E-18, 0.002229328859797958130, 0.004458657719595912790, 0.006687986579393867884, 0.008917315439191822110, 0.01337597315878773230, 0.01783463087838364075, 0.02006395973818160192, 0.02229328859797955961, 0.02452261745777752078, 0.02675194631757547847, 0.03121060403717131754, 0.03232526846707026169, 0.03343993289696921278, 0.03566926175676703170 ),
 .UNSPECIFIED. ) ;
#10069=CARTESIAN_POINT ( 'NONE',  ( 9.345921402568846403, 139.9999999999999716, -15.00000000000000000 ) ) ;
#10070=DIRECTION ( 'NONE',  ( 0.000000000000000000, 0.000000000000000000, 1.000000000000000000 ) ) ;
#10072=EDGE_LOOP ( 'NONE', ( #26358, #11768, #25724, #15397 ) ) ;
#10073=CARTESIAN_POINT ( 'NONE',  ( -203.2481855153402250, 92.57460631283321106, 29.78692811926997308 ) ) ;
#10074=AXIS2_PLACEMENT_3D ( 'NONE', #21393, #25552, #1843 ) ;
#10076=ORIENTED_EDGE ( 'NONE', *, *, #9632, .F. ) ;
#10082=CARTESIAN_POINT ( 'NONE',  ( 99.60675733924549036, 85.63108538499666622, 100.0000000000000142 ) ) ;
#10084=CARTESIAN_POINT ( 'NONE',  ( -28.05246235954390244, 188.0718642840173516, -13.00000000000000000 ) ) ;
#10088=AXIS2_PLACEMENT_3D ( 'NONE', #2822, #11616, #16062 ) ;
#10089=DIRECTION ( 'NONE',  ( 0.000000000000000000, 0.000000000000000000, 1.000000000000000000 ) ) ;
#10092=CARTESIAN_POINT ( 'NONE',  ( 118.9718481642008641, 125.5986290015192708, 100.0000000000000142 ) ) ;
#10107=( BOUNDED_SURFACE ( )  B_SPLINE_SURFACE ( 3, 2, ( 
 ( #13985, #13838, #16130 ),
 ( #4905, #9519, #2901 ),
 ( #1024, #24880, #5194 ),
 ( #5335, #7642, #18415 ),
 ( #11543, #11686, #22441 ),
 ( #752, #25154, #18276 ),
 ( #16407, #22729, #3033 ),
 ( #11821, #20561, #27166 ),
 ( #16269, #11959, #25022 ),
 ( #14114, #2751, #22863 ),
 ( #3169, #20702, #9798 ),
 ( #18554, #5472, #24598 ),
 ( #26544, #26843, #4568 ),
 ( #17939, #7168, #19666 ),
 ( #18089, #22391, #2704 ),
 ( #6875, #15373, #15941 ),
 ( #9180, #7019, #2270 ),
 ( #562, #24128, #24690 ),
 ( #419, #2411, #26689 ),
 ( #13497, #20087, #19804 ),
 ( #4999, #9325, #12967 ),
 ( #2557, #24546, #11490 ),
 ( #279, #22246, #21827 ),
 ( #19947, #20232, #11194 ),
 ( #4855, #15805, #2133 ),
 ( #13644, #17502, #26268 ),
 ( #10907, #128, #8752 ),
 ( #6594, #4429, #15655 ),
 ( #13214, #24401, #21959 ),
 ( #11051, #8894, #17651 ),
 ( #13355, #26405, #9038 ),
 ( #17788, #6728, #11343 ),
 ( #22105, #4712, #15512 ),
 ( #24260, #9475, #16225 ),
 ( #16638, #7311, #7456 ),
 ( #20801, #18231, #25393 ),
 ( #26978, #3408, #20377 ),
 ( #705, #16086, #25251 ),
 ( #842, #18370, #27529 ),
 ( #14072, #2987, #16364 ),
 ( #9611, #24837, #5147 ),
 ( #5570, #14210, #27123 ),
 ( #7869, #9753, #22823 ),
 ( #25108, #18647, #24976 ),
 ( #22538, #27390, #20519 ),
 ( #13937, #13791, #5289 ) ),
 .UNSPECIFIED., .F., .F., .T. ) 
 B_SPLINE_SURFACE_WITH_KNOTS ( ( 4, 2, 2, 2, 2, 2, 2, 2, 2, 2, 2, 2, 2, 2, 2, 2, 2, 2, 2, 2, 2, 2, 4 ),
 ( 3, 3 ),
 ( 1.734723475976807094E-18, 0.004062158184156357439, 0.008124316368312713144, 0.01015539546039089143, 0.01218647455246906972, 0.01624863273662542629, 0.01827971182870360284, 0.02031079092078178286, 0.02437294910493813943, 0.02640402819701631598, 0.02843510728909449600, 0.03249726547325085257, 0.03655942365740720568, 0.03859050274948538917, 0.04062158184156356572, 0.04468374002571992576, 0.04874589820987627886, 0.05280805639403263196, 0.05687021457818899201, 0.05890129367026716856, 0.06093237276234535205, 0.06296345185442353554, 0.06499453094650170515 ),
 ( 0.000000000000000000, 1.000000000000000000 ),
 .UNSPECIFIED. ) 
 GEOMETRIC_REPRESENTATION_ITEM ( )  RATIONAL_B_SPLINE_SURFACE ( (
 ( 1.000000000000000000, 0.7071067811865475727, 1.000000000000000000),
 ( 1.000000000000000000, 0.7127618277282585790, 1.000000000000000000),
 ( 1.000000000000000000, 0.7177019917272278171, 1.000000000000000000),
 ( 1.000000000000000000, 0.7259809929038707477, 1.000000000000000000),
 ( 1.000000000000000000, 0.7293222386929405499, 1.000000000000000000),
 ( 1.000000000000000000, 0.7329411530155929277, 1.000000000000000000),
 ( 1.000000000000000000, 0.7339161091547746762, 1.000000000000000000),
 ( 1.000000000000000000, 0.7353380047207397352, 1.000000000000000000),
 ( 1.000000000000000000, 0.7357895841719410690, 1.000000000000000000),
 ( 1.000000000000000000, 0.7363489957920964502, 1.000000000000000000),
 ( 1.000000000000000000, 0.7356640979630035826, 1.000000000000000000),
 ( 1.000000000000000000, 0.7329334158298154156, 1.000000000000000000),
 ( 1.000000000000000000, 0.7317386460502656176, 1.000000000000000000),
 ( 1.000000000000000000, 0.7287527534627166181, 1.000000000000000000),
 ( 1.000000000000000000, 0.7269678409236182137, 1.000000000000000000),
 ( 1.000000000000000000, 0.7207930214942670499, 1.000000000000000000),
 ( 1.000000000000000000, 0.7155672824331827941, 1.000000000000000000),
 ( 1.000000000000000000, 0.7060917826293187094, 1.000000000000000000),
 ( 1.000000000000000000, 0.7026601427810345024, 1.000000000000000000),
 ( 1.000000000000000000, 0.6952527892509122731, 1.000000000000000000),
 ( 1.000000000000000000, 0.6912624871066671561, 1.000000000000000000),
 ( 1.000000000000000000, 0.6786163957654665069, 1.000000000000000000),
 ( 1.000000000000000000, 0.6692836425642715303, 1.000000000000000000),
 ( 1.000000000000000000, 0.6490371914780060925, 1.000000000000000000),
 ( 1.000000000000000000, 0.6381215166341221989, 1.000000000000000000),
 ( 1.000000000000000000, 0.6207537710089482408, 1.000000000000000000),
 ( 1.000000000000000000, 0.6147992736454299667, 1.000000000000000000),
 ( 1.000000000000000000, 0.6026007117946927671, 1.000000000000000000),
 ( 1.000000000000000000, 0.5963421480515447293, 1.000000000000000000),
 ( 1.000000000000000000, 0.5773189341491167248, 1.000000000000000000),
 ( 1.000000000000000000, 0.5643376819677715650, 1.000000000000000000),
 ( 1.000000000000000000, 0.5383412250591570469, 1.000000000000000000),
 ( 1.000000000000000000, 0.5253226519624610846, 1.000000000000000000),
 ( 1.000000000000000000, 0.5000277150692035155, 1.000000000000000000),
 ( 1.000000000000000000, 0.4877436159665405335, 1.000000000000000000),
 ( 1.000000000000000000, 0.4650351994093656072, 1.000000000000000000),
 ( 1.000000000000000000, 0.4547962088601842923, 1.000000000000000000),
 ( 1.000000000000000000, 0.4420154047700521338, 1.000000000000000000),
 ( 1.000000000000000000, 0.4381857281609657373, 1.000000000000000000),
 ( 1.000000000000000000, 0.4315381087321277787, 1.000000000000000000),
 ( 1.000000000000000000, 0.4287205967313478805, 1.000000000000000000),
 ( 1.000000000000000000, 0.4242344318730199015, 1.000000000000000000),
 ( 1.000000000000000000, 0.4225662398543922893, 1.000000000000000000),
 ( 1.000000000000000000, 0.4204880647989017173, 1.000000000000000000),
 ( 1.000000000000000000, 0.4200800889062838439, 1.000000000000000000),
 ( 1.000000000000000000, 0.4203293914240995299, 1.000000000000000000) ) ) 
 REPRESENTATION_ITEM ( '' )  SURFACE ( )  );
#10110=CARTESIAN_POINT ( 'NONE',  ( -56.48697296830715686, 1.968917815184006985E-15, 99.00000000000000000 ) ) ;
#10112=LINE ( 'NONE', #10252, #14194 ) ;
#10113=AXIS2_PLACEMENT_3D ( 'NONE', #7955, #20603, #5658 ) ;
#10116=FACE_OUTER_BOUND ( 'NONE', #11901, .T. ) ;
#10117=DIRECTION ( 'NONE',  ( 1.000000000000000000, -0.000000000000000000, -0.000000000000000000 ) ) ;
#10121=CARTESIAN_POINT ( 'NONE',  ( 134.9999999999998579, 220.0000000000000284, -90.00000000000002842 ) ) ;
#10124=CARTESIAN_POINT ( 'NONE',  ( 108.6430962847606736, 252.6780396303561247, 32.26456250497143685 ) ) ;
#10131=ORIENTED_EDGE ( 'NONE', *, *, #4797, .T. ) ;
#10134=LINE ( 'NONE', #25213, #9430 ) ;
#10145=CARTESIAN_POINT ( 'NONE',  ( -217.0264852877946566, -91.18033988749901653, 0.000000000000000000 ) ) ;
#10146=ORIENTED_EDGE ( 'NONE', *, *, #13882, .F. ) ;
#10150=CARTESIAN_POINT ( 'NONE',  ( 26.84558326594468625, 84.84596205450714024, 99.61258732158417217 ) ) ;
#10151=DIRECTION ( 'NONE',  ( -1.000000000000000000, 0.000000000000000000, 0.000000000000000000 ) ) ;
#10159=ORIENTED_EDGE ( 'NONE', *, *, #6593, .T. ) ;
#10160=CARTESIAN_POINT ( 'NONE',  ( -52.82053747318527570, 131.8412021680207431, 16.12000459196658397 ) ) ;
#10164=CARTESIAN_POINT ( 'NONE',  ( -189.8086322075389774, 92.49158130768422836, 12.99999999999999822 ) ) ;
#10168=CARTESIAN_POINT ( 'NONE',  ( -134.9821047572740156, 129.7556574183901432, -16.76521942151183708 ) ) ;
#10170=EDGE_CURVE ( 'NONE', #17928, #27752, #26180, .T. ) ;
#10171=FACE_OUTER_BOUND ( 'NONE', #14440, .T. ) ;
#10176=CARTESIAN_POINT ( 'NONE',  ( -205.4481996895170539, 90.78692297191672367, 28.57879081633423368 ) ) ;
#10179=DIRECTION ( 'NONE',  ( 0.000000000000000000, 0.000000000000000000, -1.000000000000000000 ) ) ;
#10180=EDGE_LOOP ( 'NONE', ( #28008, #18255, #4174, #16522 ) ) ;
#10183=VERTEX_POINT ( 'NONE', #8666 ) ;
#10187=ORIENTED_EDGE ( 'NONE', *, *, #16555, .T. ) ;
#10189=CIRCLE ( 'NONE', #26231, 9.999999999999991118 ) ;
#10192=TOROIDAL_SURFACE ( 'NONE', #16174, 11.00000000000001066, 1.000000000000000000 ) ;
#10193=ORIENTED_EDGE ( 'NONE', *, *, #12476, .T. ) ;
#10194=EDGE_CURVE ( 'NONE', #22091, #8949, #17978, .T. ) ;
#10200=LINE ( 'NONE', #1708, #7043 ) ;
#10201=AXIS2_PLACEMENT_3D ( 'NONE', #14127, #23435, #1316 ) ;
#10202=CARTESIAN_POINT ( 'NONE',  ( -7.973710589631370027, 131.1492272393548433, -16.33314721351600340 ) ) ;
#10203=TOROIDAL_SURFACE ( 'NONE', #16629, 11.00000000000001066, 1.000000000000000000 ) ;
#10205=DIRECTION ( 'NONE',  ( -0.000000000000000000, -0.000000000000000000, 1.000000000000000000 ) ) ;
#10207=CARTESIAN_POINT ( 'NONE',  ( -248.1546605714623013, -91.18033988749901653, 10.70611877156249214 ) ) ;
#10210=DIRECTION ( 'NONE',  ( 0.000000000000000000, 0.000000000000000000, -1.000000000000000000 ) ) ;
#10212=FACE_OUTER_BOUND ( 'NONE', #25862, .T. ) ;
#10216=VERTEX_POINT ( 'NONE', #6504 ) ;
#10219=EDGE_CURVE ( 'NONE', #18978, #19273, #21739, .T. ) ;
#10220=AXIS2_PLACEMENT_3D ( 'NONE', #14972, #19268, #10089 ) ;
#10223=CARTESIAN_POINT ( 'NONE',  ( 118.9718481642008641, 125.5986290015192708, 100.0000000000000142 ) ) ;
#10227=ORIENTED_EDGE ( 'NONE', *, *, #19364, .T. ) ;
#10235=ORIENTED_EDGE ( 'NONE', *, *, #5464, .F. ) ;
#10238=CARTESIAN_POINT ( 'NONE',  ( -524.0002167759885197, -169.4627935898112696, 0.000000000000000000 ) ) ;
#10243=PLANE ( 'NONE',  #27999 ) ;
#10249=AXIS2_PLACEMENT_3D ( 'NONE', #13192, #103, #26097 ) ;
#10252=CARTESIAN_POINT ( 'NONE',  ( -112.3221550338875687, 17.24192588826928585, 83.00000000000001421 ) ) ;
#10254=CARTESIAN_POINT ( 'NONE',  ( -201.6077923708984656, 94.40672121051507304, 29.51043390529410004 ) ) ;
#10256=CARTESIAN_POINT ( 'NONE',  ( -230.8252095005209128, 92.50430350379889433, 12.99999999999994849 ) ) ;
#10261=CARTESIAN_POINT ( 'NONE',  ( -160.0000000000000284, 119.7660240611718763, 22.85081902853005431 ) ) ;
#10262=CARTESIAN_POINT ( 'NONE',  ( 107.1322492465393736, 249.6642686020492476, 26.92713756708314321 ) ) ;
#10272=ORIENTED_EDGE ( 'NONE', *, *, #17716, .F. ) ;
#10273=AXIS2_PLACEMENT_3D ( 'NONE', #13580, #22330, #26923 ) ;
#10275=CARTESIAN_POINT ( 'NONE',  ( -227.8378063125350650, 130.6400894613935293, 12.99999999999999822 ) ) ;
#10276=DIRECTION ( 'NONE',  ( 0.000000000000000000, -1.387778780781445429E-16, -1.000000000000000000 ) ) ;
#10278=CARTESIAN_POINT ( 'NONE',  ( 115.6411010564591777, 208.5333949359988139, -99.00000000000001421 ) ) ;
#10279=FACE_OUTER_BOUND ( 'NONE', #8910, .T. ) ;
#10280=FACE_OUTER_BOUND ( 'NONE', #14936, .T. ) ;
#10283=LINE ( 'NONE', #14458, #8176 ) ;
#10288=CARTESIAN_POINT ( 'NONE',  ( 97.02586881228830862, 241.2701687844766809, -10.66912238342227681 ) ) ;
#10289=CARTESIAN_POINT ( 'NONE',  ( 20.33006372853257560, 88.24318430726339102, 98.85875548193735085 ) ) ;
#10292=ORIENTED_EDGE ( 'NONE', *, *, #25428, .T. ) ;
#10296=EDGE_CURVE ( 'NONE', #13033, #22331, #16610, .T. ) ;
#10299=CARTESIAN_POINT ( 'NONE',  ( -82.72216334395888282, 136.4210859576436974, 13.48999651779888254 ) ) ;
#10302=CARTESIAN_POINT ( 'NONE',  ( 114.6860526936801534, 210.2756460775362086, 98.48425370696797643 ) ) ;
#10304=CARTESIAN_POINT ( 'NONE',  ( -150.9620302853898295, 123.3689204320809125, -20.02690237861579803 ) ) ;
#10306=PLANE ( 'NONE',  #11935 ) ;
#10309=CARTESIAN_POINT ( 'NONE',  ( -225.7036482868739427, -91.18033988749901653, 0.000000000000000000 ) ) ;
#10310=CARTESIAN_POINT ( 'NONE',  ( 19.81673173095627050, -48.35333013564442695, 98.81407962859346128 ) ) ;
#10311=CARTESIAN_POINT ( 'NONE',  ( -220.2847051492696551, 86.26875468262431923, -18.58588010854248651 ) ) ;
#10314=CARTESIAN_POINT ( 'NONE',  ( -208.8144187295359302, 88.72373865873345267, 26.17480155654782337 ) ) ;
#10316=CARTESIAN_POINT ( 'NONE',  ( -160.0000000000000284, 79.99999999999994316, -70.00000000000001421 ) ) ;
#10317=DIRECTION ( 'NONE',  ( 1.000000000000000000, 0.000000000000000000, 0.000000000000000000 ) ) ;
#10319=EDGE_CURVE ( 'NONE', #16689, #15640, #2377, .T. ) ;
#10323=ORIENTED_EDGE ( 'NONE', *, *, #1773, .T. ) ;
#10325=CARTESIAN_POINT ( 'NONE',  ( 106.0806716805053611, 248.0923932631361595, -24.09863730005714544 ) ) ;
#10332=EDGE_CURVE ( 'NONE', #12221, #3706, #10189, .T. ) ;
#10333=ORIENTED_EDGE ( 'NONE', *, *, #27848, .T. ) ;
#10335=ORIENTED_EDGE ( 'NONE', *, *, #26233, .T. ) ;
#10340=CARTESIAN_POINT ( 'NONE',  ( -0.4949115998893022783, 134.1005191953554743, -15.57096562799038963 ) ) ;
#10344=CARTESIAN_POINT ( 'NONE',  ( -207.5044420441007560, 75.59897387903043864, -44.47015349860520672 ) ) ;
#10354=PLANE ( 'NONE',  #22739 ) ;
#10363=B_SPLINE_CURVE_WITH_KNOTS ( 'NONE', 3,
 ( #19926, #15208, #17483, #8872, #26247, #14922, #28108, #12912, #23962, #23818 ),
 .UNSPECIFIED., .F., .F.,
 ( 4, 2, 2, 2, 4 ),
 ( 0.000000000000000000, 0.2500000000000000000, 0.5000000000000000000, 0.7500000000000000000, 1.000000000000000000 ),
 .UNSPECIFIED. ) ;
#10370=CARTESIAN_POINT ( 'NONE',  ( -185.9688816675270289, 106.1730371456491753, -31.51842731530989639 ) ) ;
#10379=DIRECTION ( 'NONE',  ( 0.7059982162894324897, -0.7082136108520787898, 0.000000000000000000 ) ) ;
#10382=CARTESIAN_POINT ( 'NONE',  ( 134.9999999999998579, 220.0000000000000284, 99.00000000000001421 ) ) ;
#10383=AXIS2_PLACEMENT_3D ( 'NONE', #13290, #10844, #19602 ) ;
#10386=FACE_OUTER_BOUND ( 'NONE', #1616, .T. ) ;
#10388=CARTESIAN_POINT ( 'NONE',  ( 118.3276951936840220, 235.1525654889200894, 99.88760442621966718 ) ) ;
#10389=ADVANCED_FACE ( 'NONE', ( #7078 ), #17994, .F. ) ;
#10395=ORIENTED_EDGE ( 'NONE', *, *, #20436, .T. ) ;
#10403=ORIENTED_EDGE ( 'NONE', *, *, #13584, .T. ) ;
#10408=VERTEX_POINT ( 'NONE', #27442 ) ;
#10412=CARTESIAN_POINT ( 'NONE',  ( 8.117852850209656523, 141.5785587194356481, 12.99999999999999822 ) ) ;
#10413=CARTESIAN_POINT ( 'NONE',  ( -230.8916957670046486, 130.8330661503599117, -5.000000000000002665 ) ) ;
#10417=CARTESIAN_POINT ( 'NONE',  ( -226.6532499065050388, 62.99057865342161477, -8.245540320822751568 ) ) ;
#10418=ORIENTED_EDGE ( 'NONE', *, *, #6350, .T. ) ;
#10427=AXIS2_PLACEMENT_3D ( 'NONE', #1809, #19340, #19487 ) ;
#10428=CARTESIAN_POINT ( 'NONE',  ( 33.10302365956999182, 221.6666220619077876, 15.00000000000000000 ) ) ;
#10438=ORIENTED_EDGE ( 'NONE', *, *, #12293, .T. ) ;
#10443=CARTESIAN_POINT ( 'NONE',  ( 113.0677398990922313, 214.9520504348329553, 97.20864094219221840 ) ) ;
#10447=CARTESIAN_POINT ( 'NONE',  ( -160.5161435040798494, 120.3804527765386752, -22.28951900308573641 ) ) ;
#10448=CARTESIAN_POINT ( 'NONE',  ( -200.0000000000000284, 0.000000000000000000, 25.00000000000000000 ) ) ;
#10450=DIRECTION ( 'NONE',  ( -0.8018642810807398158, -0.5975062131282554700, 0.000000000000000000 ) ) ;
#10451=CARTESIAN_POINT ( 'NONE',  ( -211.3659712544258298, 88.58350419819547028, -23.76025086788270357 ) ) ;
#10458=ORIENTED_EDGE ( 'NONE', *, *, #801, .F. ) ;
#10459=ADVANCED_FACE ( 'NONE', ( #21850 ), #10791, .F. ) ;
#10463=DIRECTION ( 'NONE',  ( 0.000000000000000000, -1.000000000000000000, 0.000000000000000000 ) ) ;
#10465=DIRECTION ( 'NONE',  ( 0.000000000000000000, 0.000000000000000000, -1.000000000000000000 ) ) ;
#10468=CARTESIAN_POINT ( 'NONE',  ( 94.58250724493984762, 231.5191281348355119, -18.77838886173819688 ) ) ;
#10469=ORIENTED_EDGE ( 'NONE', *, *, #17819, .T. ) ;
#10474=VERTEX_POINT ( 'NONE', #26148 ) ;
#10475=VERTEX_POINT ( 'NONE', #15252 ) ;
#10477=AXIS2_PLACEMENT_3D ( 'NONE', #1824, #10598, #6146 ) ;
#10485=DIRECTION ( 'NONE',  ( 1.000000000000000000, 0.000000000000000000, 0.000000000000000000 ) ) ;
#10486=ADVANCED_FACE ( 'NONE', ( #13 ), #24006, .F. ) ;
#10488=AXIS2_PLACEMENT_3D ( 'NONE', #1931, #5967, #21194 ) ;
#10489=CARTESIAN_POINT ( 'NONE',  ( -68.57415822541635464, -23.01420295945612082, 100.0000000000000000 ) ) ;
#10491=FACE_OUTER_BOUND ( 'NONE', #4622, .T. ) ;
#10495=DIRECTION ( 'NONE',  ( -0.8018642810807398158, -0.5975062131282554700, 0.000000000000000000 ) ) ;
#10496=VECTOR ( 'NONE', #21471, 1000.000000000000000 ) ;
#10498=CIRCLE ( 'NONE', #9102, 21.20097097723064294 ) ;
#10500=EDGE_LOOP ( 'NONE', ( #11, #24495, #11145, #19374 ) ) ;
#10508=CARTESIAN_POINT ( 'NONE',  ( 82.68942924492586144, 110.0997128792066206, -99.99999999998921396 ) ) ;
#10509=CARTESIAN_POINT ( 'NONE',  ( 101.0134428126900303, 235.9903891613491282, 23.57075532798359419 ) ) ;
#10511=CARTESIAN_POINT ( 'NONE',  ( -199.1255185106215322, 96.44980846386927453, -30.47972463551135647 ) ) ;
#10514=CARTESIAN_POINT ( 'NONE',  ( -232.1897660433613453, 90.99944575719695194, 14.99999999999994849 ) ) ;
#10515=EDGE_LOOP ( 'NONE', ( #20307, #13856, #23400, #20670, #19689, #5700 ) ) ;
#10518=AXIS2_PLACEMENT_3D ( 'NONE', #22114, #23993, #24412 ) ;
#10519=EDGE_CURVE ( 'NONE', #11930, #1493, #12966, .T. ) ;
#10520=CARTESIAN_POINT ( 'NONE',  ( 0.000000000000000000, -18.01420295945611727, 95.00000000000000000 ) ) ;
#10522=EDGE_CURVE ( 'NONE', #16893, #1460, #28291, .T. ) ;
#10524=VERTEX_POINT ( 'NONE', #6897 ) ;
#10525=LINE ( 'NONE', #27465, #14608 ) ;
#10526=EDGE_CURVE ( 'NONE', #15707, #20254, #18000, .T. ) ;
#10531=CARTESIAN_POINT ( 'NONE',  ( 115.6411010564592061, 231.4666050640012998, 99.00000000000001421 ) ) ;
#10532=CIRCLE ( 'NONE', #17868, 16.07743405327025243 ) ;
#10534=CARTESIAN_POINT ( 'NONE',  ( -206.8817896583512095, 90.46732954276036764, 26.12578640336038660 ) ) ;
#10538=EDGE_LOOP ( 'NONE', ( #28293, #12680, #7389, #3776 ) ) ;
#10541=CARTESIAN_POINT ( 'NONE',  ( -162.3702703317349858, 119.5357951972386985, -23.00655219379951077 ) ) ;
#10544=AXIS2_PLACEMENT_3D ( 'NONE', #15801, #9178, #17935 ) ;
#10552=AXIS2_PLACEMENT_3D ( 'NONE', #17756, #10878, #15620 ) ;
#10553=PLANE ( 'NONE',  #2533 ) ;
#10554=DIRECTION ( 'NONE',  ( 1.000000000000000000, 0.000000000000000000, 0.000000000000000000 ) ) ;
#10556=CARTESIAN_POINT ( 'NONE',  ( 118.3276951936840078, 204.8474345110799959, -99.88760442621965296 ) ) ;
#10558=DIRECTION ( 'NONE',  ( 1.850371707708594316E-16, -1.000000000000000000, 0.000000000000000000 ) ) ;
#10559=CARTESIAN_POINT ( 'NONE',  ( -236.2622743973891772, 68.21227378728583801, -5.744226217427297776 ) ) ;
#10562=DIRECTION ( 'NONE',  ( 1.000000000000000000, 0.000000000000000000, 0.000000000000000000 ) ) ;
#10564=CARTESIAN_POINT ( 'NONE',  ( 113.9142275403307565, 227.9126300401528908, -97.94883453769639914 ) ) ;
#10565=ORIENTED_EDGE ( 'NONE', *, *, #4122, .F. ) ;
#10567=EDGE_CURVE ( 'NONE', #10408, #6088, #25448, .T. ) ;
#10570=DIRECTION ( 'NONE',  ( -0.2458199939946738577, -0.9693154958796741383, 0.000000000000000000 ) ) ;
#10575=DIRECTION ( 'NONE',  ( -1.000000000000000000, 0.000000000000000000, 0.000000000000000000 ) ) ;
#10577=CARTESIAN_POINT ( 'NONE',  ( -71.37541315349507443, 240.0000000000000000, 5.000000000000002665 ) ) ;
#10579=EDGE_CURVE ( 'NONE', #11112, #18951, #24282, .T. ) ;
#10580=ORIENTED_EDGE ( 'NONE', *, *, #7231, .F. ) ;
#10586=CARTESIAN_POINT ( 'NONE',  ( 112.5004877479093324, 218.9596622748219090, 96.61493133138614553 ) ) ;
#10587=CARTESIAN_POINT ( 'NONE',  ( -67.63633724927728963, 133.9262831905602127, -15.61889904559025943 ) ) ;
#10589=ADVANCED_FACE ( 'NONE', ( #11662, #18252 ), #7478, .F. ) ;
#10590=CARTESIAN_POINT ( 'NONE',  ( -148.2611599703591878, 125.4274327989001137, -17.54707401466952632 ) ) ;
#10593=CARTESIAN_POINT ( 'NONE',  ( -226.3292334817031985, 89.73541284941354945, -15.87801632005360553 ) ) ;
#10598=DIRECTION ( 'NONE',  ( 0.000000000000000000, 0.000000000000000000, 1.000000000000000000 ) ) ;
#10602=CIRCLE ( 'NONE', #9228, 89.71075545852265520 ) ;
#10607=ORIENTED_EDGE ( 'NONE', *, *, #18351, .T. ) ;
#10609=CARTESIAN_POINT ( 'NONE',  ( 100.2919976486446387, 242.8371140005963866, -14.10862752715507540 ) ) ;
#10611=ORIENTED_EDGE ( 'NONE', *, *, #6465, .F. ) ;
#10619=DIRECTION ( 'NONE',  ( 1.000000000000000000, 0.000000000000000000, 0.000000000000000000 ) ) ;
#10621=VECTOR ( 'NONE', #20921, 1000.000000000000000 ) ;
#10622=DIRECTION ( 'NONE',  ( 4.163336342344337027E-16, -1.000000000000000000, 1.387778780781445429E-16 ) ) ;
#10629=VECTOR ( 'NONE', #13429, 1000.000000000000000 ) ;
#10630=DIRECTION ( 'NONE',  ( 1.000000000000000000, 0.000000000000000000, 0.000000000000000000 ) ) ;
#10631=DIRECTION ( 'NONE',  ( 0.000000000000000000, 0.000000000000000000, 1.000000000000000000 ) ) ;
#10632=ADVANCED_FACE ( 'NONE', ( #7336 ), #446, .T. ) ;
#10636=ORIENTED_EDGE ( 'NONE', *, *, #12021, .T. ) ;
#10637=AXIS2_PLACEMENT_3D ( 'NONE', #25065, #2320, #14860 ) ;
#10638=CARTESIAN_POINT ( 'NONE',  ( -188.7674184428050239, 104.2604349191509101, 32.38797585049563565 ) ) ;
#10640=CARTESIAN_POINT ( 'NONE',  ( -140.1213116003368668, 122.5384136796733827, 15.00000000000000000 ) ) ;
#10641=ORIENTED_EDGE ( 'NONE', *, *, #22979, .T. ) ;
#10644=ORIENTED_EDGE ( 'NONE', *, *, #2436, .T. ) ;
#10650=CARTESIAN_POINT ( 'NONE',  ( 82.91040908012101340, 80.00000000661717081, -100.0000000000000142 ) ) ;
#10654=CARTESIAN_POINT ( 'NONE',  ( -164.5329923790834528, 118.5024393687872504, -22.94354786372609212 ) ) ;
#10656=CARTESIAN_POINT ( 'NONE',  ( -220.0435420340362214, 87.92826792072207809, 18.32348305083313278 ) ) ;
#10664=ORIENTED_EDGE ( 'NONE', *, *, #4761, .F. ) ;
#10667=DIRECTION ( 'NONE',  ( 1.000000000000000000, 4.163336342344337027E-16, -0.000000000000000000 ) ) ;
#10675=CARTESIAN_POINT ( 'NONE',  ( -181.6509543635144439, 108.9824211742952116, 30.31695520427327750 ) ) ;
#10678=VERTEX_POINT ( 'NONE', #15770 ) ;
#10682=VECTOR ( 'NONE', #23046, 1000.000000000000000 ) ;
#10684=CARTESIAN_POINT ( 'NONE',  ( -182.9507880900968360, 107.8942440073746951, -31.71834794605663532 ) ) ;
#10685=VERTEX_POINT ( 'NONE', #26952 ) ;
#10686=ADVANCED_FACE ( 'NONE', ( #4824 ), #11607, .F. ) ;
#10687=ORIENTED_EDGE ( 'NONE', *, *, #21180, .T. ) ;
#10688=ADVANCED_FACE ( 'NONE', ( #4679 ), #2381, .T. ) ;
#10702=FACE_OUTER_BOUND ( 'NONE', #10055, .T. ) ;
#10703=CARTESIAN_POINT ( 'NONE',  ( -143.6428522700808230, 68.51688903468615877, 83.00000000000001421 ) ) ;
#10704=CARTESIAN_POINT ( 'NONE',  ( -227.4113622183683106, 63.29489605847815881, -7.985794955240778314 ) ) ;
#10709=DIRECTION ( 'NONE',  ( 0.000000000000000000, 1.000000000000000000, -1.224646799147353207E-16 ) ) ;
#10711=ORIENTED_EDGE ( 'NONE', *, *, #19631, .T. ) ;
#10715=DIRECTION ( 'NONE',  ( 1.000000000000000000, 0.000000000000000000, 0.000000000000000000 ) ) ;
#10716=CARTESIAN_POINT ( 'NONE',  ( 139.9999999999999147, 4.857225732735056078E-14, -100.0000000000000142 ) ) ;
#10718=ORIENTED_EDGE ( 'NONE', *, *, #16901, .F. ) ;
#10720=ADVANCED_FACE ( 'NONE', ( #8860 ), #22137, .T. ) ;
#10721=CIRCLE ( 'NONE', #171, 30.49120955644046660 ) ;
#10726=ORIENTED_EDGE ( 'NONE', *, *, #259, .T. ) ;
#10730=ADVANCED_FACE ( 'NONE', ( #6985 ), #6841, .T. ) ;
#10731=EDGE_LOOP ( 'NONE', ( #28051, #16442, #19686, #4877 ) ) ;
#10732=ORIENTED_EDGE ( 'NONE', *, *, #2120, .T. ) ;
#10733=DIRECTION ( 'NONE',  ( -1.000000000000000000, 0.000000000000000000, 0.000000000000000000 ) ) ;
#10739=CIRCLE ( 'NONE', #6608, 21.49999999999997868 ) ;
#10741=CARTESIAN_POINT ( 'NONE',  ( -196.7918453702777128, 20.24192588826927164, 93.88690167569080813 ) ) ;
#10742=CARTESIAN_POINT ( 'NONE',  ( -233.2943309833543140, 92.06151970357154823, -14.99999999999999645 ) ) ;
#10743=CARTESIAN_POINT ( 'NONE',  ( 89.99999999999988631, 240.0000000000000284, -6.270166537926030514 ) ) ;
#10744=CARTESIAN_POINT ( 'NONE',  ( -112.3221550338875687, 74.54464929955099706, 80.00000000000001421 ) ) ;
#10749=VERTEX_POINT ( 'NONE', #17906 ) ;
#10755=CARTESIAN_POINT ( 'NONE',  ( 96.18084660807248554, 232.2996298045119943, -19.72083291508440794 ) ) ;
#10757=DIRECTION ( 'NONE',  ( 0.000000000000000000, 0.000000000000000000, -1.000000000000000000 ) ) ;
#10759=ORIENTED_EDGE ( 'NONE', *, *, #17388, .F. ) ;
#10760=VERTEX_POINT ( 'NONE', #6699 ) ;
#10763=ORIENTED_EDGE ( 'NONE', *, *, #18926, .F. ) ;
#10765=ADVANCED_FACE ( 'NONE', ( #15623 ), #528, .F. ) ;
#10769=DIRECTION ( 'NONE',  ( 1.000000000000000000, 1.541976423090495880E-16, 0.000000000000000000 ) ) ;
#10771=CARTESIAN_POINT ( 'NONE',  ( -63.57415822541634043, -18.01420295945611727, 95.00000000000000000 ) ) ;
#10773=DIRECTION ( 'NONE',  ( 0.000000000000000000, 0.000000000000000000, 1.000000000000000000 ) ) ;
#10775=EDGE_CURVE ( 'NONE', #20507, #14873, #14338, .T. ) ;
#10776=ADVANCED_FACE ( 'NONE', ( #21930 ), #13464, .T. ) ;
#10777=LINE ( 'NONE', #6457, #20575 ) ;
#10783=ORIENTED_EDGE ( 'NONE', *, *, #19549, .T. ) ;
#10784=CARTESIAN_POINT ( 'NONE',  ( -180.6173853931124711, 109.6284025331804628, 30.49881833197462910 ) ) ;
#10786=ORIENTED_EDGE ( 'NONE', *, *, #4671, .F. ) ;
#10788=ADVANCED_FACE ( 'NONE', ( #677 ), #13324, .T. ) ;
#10791=CYLINDRICAL_SURFACE ( 'NONE', #3779, 5.000000000000004441 ) ;
#10796=CARTESIAN_POINT ( 'NONE',  ( 93.07270601803662657, 112.9533406971499971, -74.06249999970600584 ) ) ;
#10797=AXIS2_PLACEMENT_3D ( 'NONE', #5500, #22758, #1053 ) ;
#10799=CARTESIAN_POINT ( 'NONE',  ( -173.5285038084994085, 113.8115965281807576, -27.00126897022071404 ) ) ;
#10800=ORIENTED_EDGE ( 'NONE', *, *, #2567, .T. ) ;
#10801=CARTESIAN_POINT ( 'NONE',  ( -222.5854910735133387, 88.44175340957714582, 17.19091714286218320 ) ) ;
#10803=VECTOR ( 'NONE', #10958, 1000.000000000000000 ) ;
#10805=DIRECTION ( 'NONE',  ( 1.000000000000000000, -0.000000000000000000, -0.000000000000000000 ) ) ;
#10809=CARTESIAN_POINT ( 'NONE',  ( 116.2405502098311558, 207.5638714341443176, 99.27293966533068215 ) ) ;
#10810=AXIS2_PLACEMENT_3D ( 'NONE', #19730, #26333, #55 ) ;
#10812=DIRECTION ( 'NONE',  ( 0.000000000000000000, 0.000000000000000000, 1.000000000000000000 ) ) ;
#10815=VERTEX_POINT ( 'NONE', #7134 ) ;
#10818=LINE ( 'NONE', #24307, #17598 ) ;
#10820=DIRECTION ( 'NONE',  ( 1.000000000000000000, 1.321694076934710155E-16, -0.000000000000000000 ) ) ;
#10825=CARTESIAN_POINT ( 'NONE',  ( -185.9585935723647765, 106.1799384177000718, -31.51628191568552140 ) ) ;
#10831=ORIENTED_EDGE ( 'NONE', *, *, #24014, .F. ) ;
#10834=PLANE ( 'NONE',  #24451 ) ;
#10840=LINE ( 'NONE', #11272, #1402 ) ;
#10842=CARTESIAN_POINT ( 'NONE',  ( -226.0190876347137419, 72.67478414372106954, -17.85134081709557563 ) ) ;
#10844=DIRECTION ( 'NONE',  ( 0.8018642810807398158, 0.5975062131282554700, -0.000000000000000000 ) ) ;
#10846=CARTESIAN_POINT ( 'NONE',  ( -63.57415822541634043, 80.97823757117562593, 80.00000000000001421 ) ) ;
#10847=DIRECTION ( 'NONE',  ( -0.000000000000000000, 0.000000000000000000, 1.000000000000000000 ) ) ;
#10848=CARTESIAN_POINT ( 'NONE',  ( 112.7775258882242468, 223.5591602065040036, -96.91707758366551673 ) ) ;
#10852=ADVANCED_FACE ( 'NONE', ( #5397 ), #20767, .F. ) ;
#10855=CARTESIAN_POINT ( 'NONE',  ( -76.25760768171835480, 221.6666220619077876, 15.00000000000000000 ) ) ;
#10858=DIRECTION ( 'NONE',  ( 0.8314772792026874360, -0.5555587585212711232, 0.000000000000000000 ) ) ;
#10861=LINE ( 'NONE', #9274, #21688 ) ;
#10865=VECTOR ( 'NONE', #5259, 1000.000000000000000 ) ;
#10866=VERTEX_POINT ( 'NONE', #23071 ) ;
#10868=ORIENTED_EDGE ( 'NONE', *, *, #6390, .T. ) ;
#10871=CARTESIAN_POINT ( 'NONE',  ( -52.82542805791850782, 131.8416355074880073, -16.11994505319805526 ) ) ;
#10875=CONICAL_SURFACE ( 'NONE', #16838, 6.025000000000002132, 0.7853981633974482790 ) ;
#10878=DIRECTION ( 'NONE',  ( -0.000000000000000000, -0.000000000000000000, 1.000000000000000000 ) ) ;
#10881=CARTESIAN_POINT ( 'NONE',  ( -211.8454146708414498, 88.46767467987882583, -21.92683318774069079 ) ) ;
#10887=ORIENTED_EDGE ( 'NONE', *, *, #16934, .F. ) ;
#10891=DIRECTION ( 'NONE',  ( 1.850371707708594316E-16, -1.000000000000000000, 0.000000000000000000 ) ) ;
#10892=CARTESIAN_POINT ( 'NONE',  ( 33.10302365956999182, 203.2034914284457159, 12.99999999999999822 ) ) ;
#10894=EDGE_CURVE ( 'NONE', #20219, #14406, #22621, .T. ) ;
#10895=CARTESIAN_POINT ( 'NONE',  ( 91.17299970895513184, 230.3777436784973816, -17.14176051628210828 ) ) ;
#10897=CARTESIAN_POINT ( 'NONE',  ( -13.80176969007178478, 130.8724268707720171, -14.97137485413120395 ) ) ;
#10901=ORIENTED_EDGE ( 'NONE', *, *, #4585, .F. ) ;
#10905=FACE_OUTER_BOUND ( 'NONE', #16484, .T. ) ;
#10907=CARTESIAN_POINT ( 'NONE',  ( -206.2579005266799186, 60.21847207785817346, 20.52143262683453528 ) ) ;
#10910=EDGE_CURVE ( 'NONE', #5551, #14300, #15285, .T. ) ;
#10912=DIRECTION ( 'NONE',  ( 2.602085213965210642E-16, -1.000000000000000000, 0.000000000000000000 ) ) ;
#10915=DIRECTION ( 'NONE',  ( -0.000000000000000000, 0.000000000000000000, 1.000000000000000000 ) ) ;
#10916=CARTESIAN_POINT ( 'NONE',  ( -209.0137874940113818, 69.92142720080950369, 37.51845061662766057 ) ) ;
#10917=CARTESIAN_POINT ( 'NONE',  ( -71.37541315349507443, 150.2892445414773590, -5.000000000000004441 ) ) ;
#10918=FACE_OUTER_BOUND ( 'NONE', #20753, .T. ) ;
#10921=CARTESIAN_POINT ( 'NONE',  ( -184.2222344732742556, 107.3439714424985993, 31.61955583114170309 ) ) ;
#10925=ORIENTED_EDGE ( 'NONE', *, *, #2663, .T. ) ;
#10927=EDGE_CURVE ( 'NONE', #7126, #15348, #15735, .T. ) ;
#10928=ORIENTED_EDGE ( 'NONE', *, *, #8545, .F. ) ;
#10932=DIRECTION ( 'NONE',  ( 1.000000000000000000, -0.000000000000000000, -0.000000000000000000 ) ) ;
#10936=CARTESIAN_POINT ( 'NONE',  ( 109.9999999999999147, 137.0808454112663810, -89.99999999930710715 ) ) ;
#10939=CARTESIAN_POINT ( 'NONE',  ( 109.9999999999999147, 140.0000000000000000, 100.0000000000000142 ) ) ;
#10941=CARTESIAN_POINT ( 'NONE',  ( -211.3652297710211201, 88.58433376602883413, 23.76089942878013161 ) ) ;
#10946=CARTESIAN_POINT ( 'NONE',  ( 109.9999999999999289, -90.00000000000001421, -70.00000000000001421 ) ) ;
#10947=ORIENTED_EDGE ( 'NONE', *, *, #17974, .T. ) ;
#10950=CARTESIAN_POINT ( 'NONE',  ( 139.9999999999999716, -100.0000000000000000, 100.0000000000000142 ) ) ;
#10953=ORIENTED_EDGE ( 'NONE', *, *, #7052, .F. ) ;
#10958=DIRECTION ( 'NONE',  ( 1.000000000000000000, 1.530283246943720875E-16, -0.000000000000000000 ) ) ;
#10961=VERTEX_POINT ( 'NONE', #5959 ) ;
#10964=CARTESIAN_POINT ( 'NONE',  ( -191.3994286864096637, 102.3862160203461400, -32.47203723438894940 ) ) ;
#10965=EDGE_LOOP ( 'NONE', ( #20710, #11573, #8111, #14319 ) ) ;
#10966=ADVANCED_FACE ( 'NONE', ( #10280 ), #8086, .T. ) ;
#10968=CARTESIAN_POINT ( 'NONE',  ( -524.0002167759885197, -169.4627935898112696, 0.000000000000000000 ) ) ;
#10969=CONICAL_SURFACE ( 'NONE', #14182, 6.025000000000002132, 0.7853981633974482790 ) ;
#10972=EDGE_LOOP ( 'NONE', ( #26833, #657, #17286, #2358 ) ) ;
#10973=ORIENTED_EDGE ( 'NONE', *, *, #14841, .T. ) ;
#10974=EDGE_CURVE ( 'NONE', #20823, #9382, #21685, .T. ) ;
#10975=CARTESIAN_POINT ( 'NONE',  ( -43.02437977270766822, 129.7200458115292747, 16.81627168235289815 ) ) ;
#10978=CARTESIAN_POINT ( 'NONE',  ( -200.0000000000000284, -91.18033988749901653, -21.20097097723064294 ) ) ;
#10998=CARTESIAN_POINT ( 'NONE',  ( 157.4999999999998579, 220.0000000000000284, 99.00000000000001421 ) ) ;
#11001=EDGE_CURVE ( 'NONE', #25311, #24933, #21114, .T. ) ;
#11004=CARTESIAN_POINT ( 'NONE',  ( 79.99999999999991473, 80.00000000000001421, -100.0000000000000142 ) ) ;
#11011=ORIENTED_EDGE ( 'NONE', *, *, #6899, .T. ) ;
#11012=VERTEX_POINT ( 'NONE', #10207 ) ;
#11013=CARTESIAN_POINT ( 'NONE',  ( -279.3160071107327553, -512.7211954420570237, -9.184850993605147944E-16 ) ) ;
#11014=CARTESIAN_POINT ( 'NONE',  ( 104.4928295061213248, 246.1605864358052713, 20.56267333364200667 ) ) ;
#11016=AXIS2_PLACEMENT_3D ( 'NONE', #4975, #6994, #13912 ) ;
#11019=DIRECTION ( 'NONE',  ( 1.000000000000000000, 0.000000000000000000, 0.000000000000000000 ) ) ;
#11024=DIRECTION ( 'NONE',  ( 0.000000000000000000, 0.000000000000000000, -1.000000000000000000 ) ) ;
#11026=CARTESIAN_POINT ( 'NONE',  ( -71.37541315349507443, 240.0000000000000000, 15.00000000000000000 ) ) ;
#11028=EDGE_LOOP ( 'NONE', ( #22305, #3249, #8174, #16239 ) ) ;
#11031=DIRECTION ( 'NONE',  ( 1.000000000000000000, 0.000000000000000000, 0.000000000000000000 ) ) ;
#11034=ORIENTED_EDGE ( 'NONE', *, *, #17136, .F. ) ;
#11037=EDGE_LOOP ( 'NONE', ( #5083, #2758, #8207, #26384 ) ) ;
#11038=CARTESIAN_POINT ( 'NONE',  ( -5.362417151017317529, 133.6996939015124326, -14.05114881981127972 ) ) ;
#11041=ORIENTED_EDGE ( 'NONE', *, *, #24397, .T. ) ;
#11042=VERTEX_POINT ( 'NONE', #7631 ) ;
#11044=DIRECTION ( 'NONE',  ( 1.000000000000000000, 0.000000000000000000, 0.000000000000000000 ) ) ;
#11046=CIRCLE ( 'NONE', #7380, 5.000000000000004441 ) ;
#11047=EDGE_CURVE ( 'NONE', #21857, #12635, #2884, .T. ) ;
#11049=CARTESIAN_POINT ( 'NONE',  ( 134.9999999999998579, 220.0000000000000284, -99.00000000000001421 ) ) ;
#11050=CIRCLE ( 'NONE', #27104, 58.59270260175150469 ) ;
#11051=CARTESIAN_POINT ( 'NONE',  ( -203.1048999768048589, 60.64878749907337152, 23.79654850876809036 ) ) ;
#11054=CARTESIAN_POINT ( 'NONE',  ( -210.7172313291012529, 103.7585653882801182, -5.000000000000004441 ) ) ;
#11057=CARTESIAN_POINT ( 'NONE',  ( -235.6744655116503964, 80.57819178535525850, -15.03015451089642873 ) ) ;
#11058=CARTESIAN_POINT ( 'NONE',  ( -26.97244491501115604, 127.9665432412413537, 17.51913689374569927 ) ) ;
#11065=CARTESIAN_POINT ( 'NONE',  ( -186.0333716493514089, 106.1453078209526950, 32.04635124596575224 ) ) ;
#11067=CARTESIAN_POINT ( 'NONE',  ( -204.2386885291766134, 92.18108640773468210, -28.15472916265547809 ) ) ;
#11069=EDGE_CURVE ( 'NONE', #14725, #5248, #6629, .T. ) ;
#11071=ORIENTED_EDGE ( 'NONE', *, *, #6593, .F. ) ;
#11073=EDGE_CURVE ( 'NONE', #25416, #223, #15380, .T. ) ;
#11075=CARTESIAN_POINT ( 'NONE',  ( -144.2277858775206028, 125.7111241703296969, 18.60581271085799315 ) ) ;
#11077=CARTESIAN_POINT ( 'NONE',  ( 85.37729192593057803, 80.27798593821322015, -100.0000000000000142 ) ) ;
#11078=ADVANCED_FACE ( 'NONE', ( #23846 ), #27991, .F. ) ;
#11080=ORIENTED_EDGE ( 'NONE', *, *, #2331, .T. ) ;
#11081=CARTESIAN_POINT ( 'NONE',  ( -226.4313904733368474, 87.63842543593344203, 16.09009735459598645 ) ) ;
#11091=CARTESIAN_POINT ( 'NONE',  ( -219.9082363642798441, 137.1815813412079308, -12.98324324887284043 ) ) ;
#11100=VERTEX_POINT ( 'NONE', #24135 ) ;
#11101=EDGE_CURVE ( 'NONE', #6472, #20401, #26132, .T. ) ;
#11104=CARTESIAN_POINT ( 'NONE',  ( -161.8838264660121808, 118.9755829189611802, -23.57291196158939073 ) ) ;
#11109=AXIS2_PLACEMENT_3D ( 'NONE', #26071, #6816, #15175 ) ;
#11112=VERTEX_POINT ( 'NONE', #2278 ) ;
#11115=EDGE_CURVE ( 'NONE', #11368, #28220, #135, .T. ) ;
#11119=DIRECTION ( 'NONE',  ( 0.000000000000000000, 0.000000000000000000, -1.000000000000000000 ) ) ;
#11120=AXIS2_PLACEMENT_3D ( 'NONE', #11740, #25353, #27084 ) ;
#11121=CARTESIAN_POINT ( 'NONE',  ( -209.9947861493998857, 60.75004723859214550, -22.65375933340435921 ) ) ;
#11122=FACE_OUTER_BOUND ( 'NONE', #15887, .T. ) ;
#11128=CARTESIAN_POINT ( 'NONE',  ( -119.0030847931093518, 214.2064521616283059, -5.000000000000002665 ) ) ;
#11129=DIRECTION ( 'NONE',  ( 1.000000000000000000, 0.000000000000000000, 0.000000000000000000 ) ) ;
#11131=ADVANCED_FACE ( 'NONE', ( #19535 ), #12660, .F. ) ;
#11136=CARTESIAN_POINT ( 'NONE',  ( -231.1953787138147050, 65.04295872140689028, -6.836033801457077175 ) ) ;
#11141=EDGE_CURVE ( 'NONE', #17245, #15024, #26275, .T. ) ;
#11142=CARTESIAN_POINT ( 'NONE',  ( -207.8817926630784712, 75.32300084315906474, 40.82685150828277898 ) ) ;
#11145=ORIENTED_EDGE ( 'NONE', *, *, #2436, .F. ) ;
#11146=EDGE_CURVE ( 'NONE', #3920, #7087, #25826, .T. ) ;
#11147=AXIS2_PLACEMENT_3D ( 'NONE', #3542, #1396, #3403 ) ;
#11149=DIRECTION ( 'NONE',  ( 1.000000000000000000, 0.000000000000000000, -0.000000000000000000 ) ) ;
#11150=CIRCLE ( 'NONE', #13918, 58.90601976618767566 ) ;
#11151=ORIENTED_EDGE ( 'NONE', *, *, #21347, .F. ) ;
#11154=CARTESIAN_POINT ( 'NONE',  ( -225.3736415174481351, 135.7651958811099178, 14.97905406095859249 ) ) ;
#11155=CARTESIAN_POINT ( 'NONE',  ( 96.03789414443664896, 240.4739163874647261, 19.46186845664385601 ) ) ;
#11156=AXIS2_PLACEMENT_3D ( 'NONE', #23932, #1939, #21777 ) ;
#11161=DIRECTION ( 'NONE',  ( -1.000000000000000000, 0.000000000000000000, 0.000000000000000000 ) ) ;
#11163=DIRECTION ( 'NONE',  ( 0.000000000000000000, 0.000000000000000000, 1.000000000000000000 ) ) ;
#11165=DIRECTION ( 'NONE',  ( 1.321694076934710155E-16, -1.000000000000000000, 0.000000000000000000 ) ) ;
#11166=CARTESIAN_POINT ( 'NONE',  ( 124.9999999999998579, 220.0000000000000284, -90.00000000000002842 ) ) ;
#11168=AXIS2_PLACEMENT_3D ( 'NONE', #18574, #7236, #13858 ) ;
#11169=DIRECTION ( 'NONE',  ( -0.000000000000000000, -0.000000000000000000, 1.000000000000000000 ) ) ;
#11174=AXIS2_PLACEMENT_3D ( 'NONE', #2674, #9153, #683 ) ;
#11178=CARTESIAN_POINT ( 'NONE',  ( 109.4601507141043157, 253.2495769758999415, -39.14599534725524421 ) ) ;
#11179=VERTEX_POINT ( 'NONE', #20385 ) ;
#11180=CARTESIAN_POINT ( 'NONE',  ( -18.15202183006797299, 129.9612872840096145, -15.33564462930252681 ) ) ;
#11181=ORIENTED_EDGE ( 'NONE', *, *, #13688, .F. ) ;
#11184=ORIENTED_EDGE ( 'NONE', *, *, #26759, .F. ) ;
#11185=EDGE_LOOP ( 'NONE', ( #4698, #10292, #20258, #25872 ) ) ;
#11186=EDGE_LOOP ( 'NONE', ( #9663, #9056, #6365, #6011 ) ) ;
#11187=CIRCLE ( 'NONE', #23566, 21.49999999999999289 ) ;
#11188=CARTESIAN_POINT ( 'NONE',  ( -141.6428522700808230, 22.24192588826928585, 80.00000000000001421 ) ) ;
#11190=DIRECTION ( 'NONE',  ( 1.000000000000000000, 1.541976423090495387E-16, -0.000000000000000000 ) ) ;
#11194=CARTESIAN_POINT ( 'NONE',  ( -217.0794644928064088, 71.41167302539513173, 24.35665452625131522 ) ) ;
#11198=CYLINDRICAL_SURFACE ( 'NONE', #16353, 30.00000000000000000 ) ;
#11199=CARTESIAN_POINT ( 'NONE',  ( -123.8208147886770121, 198.8605305197760913, -13.00000000000000000 ) ) ;
#11200=( BOUNDED_SURFACE ( )  B_SPLINE_SURFACE ( 3, 2, ( 
 ( #3218, #24041, #21740 ),
 ( #11104, #10541, #4203 ),
 ( #8530, #23897, #17423 ),
 ( #3924, #26041, #23752 ),
 ( #21592, #19582, #17144 ),
 ( #28185, #1764, #12994 ),
 ( #28040, #17564, #6361 ),
 ( #15428, #19297, #4060 ),
 ( #4478, #17705, #8390 ),
 ( #10684, #12849, #15002 ),
 ( #19442, #4344, #25900 ),
 ( #22017, #6223, #8948 ),
 ( #21877, #2050, #10825 ),
 ( #28321, #19720, #8668 ),
 ( #2325, #15142, #26181 ),
 ( #1904, #6505, #24180 ),
 ( #15289, #13138, #12711 ),
 ( #2184, #10964, #17281 ),
 ( #43, #8802, #26322 ),
 ( #6648, #21448, #13269 ),
 ( #19861, #188, #26452 ),
 ( #14864, #23611, #15710 ),
 ( #13554, #11550, #9089 ),
 ( #20144, #22161, #15859 ),
 ( #20002, #9525, #26755 ),
 ( #7368, #2467, #24463 ) ),
 .UNSPECIFIED., .F., .F., .T. ) 
 B_SPLINE_SURFACE_WITH_KNOTS ( ( 4, 2, 2, 2, 2, 2, 2, 2, 2, 2, 2, 2, 4 ),
 ( 3, 3 ),
 ( 0.000000000000000000, 0.006475292796905446693, 0.01295058559381089339, 0.01942587839071634181, 0.02590117118762178677, 0.02913881758607450925, 0.03075764078530086876, 0.03237646398452723173, 0.03561411038297995768, 0.03885175678143268363, 0.04532704957833812859, 0.04856469597679084760, 0.05180234237524357355 ),
 ( 0.000000000000000000, 1.000000000000000000 ),
 .UNSPECIFIED. ) 
 GEOMETRIC_REPRESENTATION_ITEM ( )  RATIONAL_B_SPLINE_SURFACE ( (
 ( 1.000000000000000000, 0.8981184559478653240, 1.000000000000000000),
 ( 1.000000000000000000, 0.9063539217822286220, 1.000000000000000000),
 ( 1.000000000000000000, 0.9141583029243198766, 1.000000000000000000),
 ( 1.000000000000000000, 0.9287421046155968085, 1.000000000000000000),
 ( 1.000000000000000000, 0.9355219901798119686, 1.000000000000000000),
 ( 1.000000000000000000, 0.9478609921803489158, 1.000000000000000000),
 ( 1.000000000000000000, 0.9534203654370090320, 1.000000000000000000),
 ( 1.000000000000000000, 0.9630842474809748754, 1.000000000000000000),
 ( 1.000000000000000000, 0.9671903355926384505, 1.000000000000000000),
 ( 1.000000000000000000, 0.9720373127047674533, 1.000000000000000000),
 ( 1.000000000000000000, 0.9734336496369194736, 1.000000000000000000),
 ( 1.000000000000000000, 0.9751626172152862981, 1.000000000000000000),
 ( 1.000000000000000000, 0.9756779393314085613, 1.000000000000000000),
 ( 1.000000000000000000, 0.9765794559351392845, 1.000000000000000000),
 ( 1.000000000000000000, 0.9769664380131323211, 1.000000000000000000),
 ( 1.000000000000000000, 0.9779163903307834804, 1.000000000000000000),
 ( 1.000000000000000000, 0.9782631544368628473, 1.000000000000000000),
 ( 1.000000000000000000, 0.9783930851710932464, 1.000000000000000000),
 ( 1.000000000000000000, 0.9781763639274896338, 1.000000000000000000),
 ( 1.000000000000000000, 0.9767097374471905846, 1.000000000000000000),
 ( 1.000000000000000000, 0.9746417070090728219, 1.000000000000000000),
 ( 1.000000000000000000, 0.9700692524430989394, 1.000000000000000000),
 ( 1.000000000000000000, 0.9683033234255177257, 1.000000000000000000),
 ( 1.000000000000000000, 0.9643524362418313123, 1.000000000000000000),
 ( 1.000000000000000000, 0.9621641871898499732, 1.000000000000000000),
 ( 1.000000000000000000, 0.9597817246759324794, 1.000000000000000000) ) ) 
 REPRESENTATION_ITEM ( '' )  SURFACE ( )  );
#11202=CARTESIAN_POINT ( 'NONE',  ( 81.45493510940914916, 110.0000000000000142, 70.00000000030220804 ) ) ;
#11204=CARTESIAN_POINT ( 'NONE',  ( -208.4180970336325913, 72.50582114360651076, 40.62062832311974603 ) ) ;
#11206=EDGE_CURVE ( 'NONE', #20401, #5762, #3797, .T. ) ;
#11208=ORIENTED_EDGE ( 'NONE', *, *, #26721, .F. ) ;
#11209=CIRCLE ( 'NONE', #23588, 21.59849023212046149 ) ;
#11210=CARTESIAN_POINT ( 'NONE',  ( -180.7514521273787125, 109.5450234118598161, 29.99853612640514200 ) ) ;
#11215=EDGE_CURVE ( 'NONE', #28035, #21416, #26161, .T. ) ;
#11217=VERTEX_POINT ( 'NONE', #7177 ) ;
#11221=CARTESIAN_POINT ( 'NONE',  ( -42.99650729631200363, 36.92584315232891612, 99.00000000000000000 ) ) ;
#11222=CARTESIAN_POINT ( 'NONE',  ( -138.8964747619121454, 128.5890830931904816, 15.90235027539833901 ) ) ;
#11223=ORIENTED_EDGE ( 'NONE', *, *, #27279, .F. ) ;
#11227=ORIENTED_EDGE ( 'NONE', *, *, #13007, .F. ) ;
#11229=CARTESIAN_POINT ( 'NONE',  ( -216.3450931143857758, 86.38378630374840839, 20.83050718481806030 ) ) ;
#11240=CARTESIAN_POINT ( 'NONE',  ( -223.0199379110806319, 134.9200334684691143, -15.12837422688741462 ) ) ;
#11243=ORIENTED_EDGE ( 'NONE', *, *, #13307, .T. ) ;
#11246=CARTESIAN_POINT ( 'NONE',  ( 109.9999999999999289, -90.00000000000001421, -100.0000000000000142 ) ) ;
#11247=CARTESIAN_POINT ( 'NONE',  ( -142.7917509638491254, 69.37713474640312938, 82.93960292326050876 ) ) ;
#11248=ORIENTED_EDGE ( 'NONE', *, *, #5631, .T. ) ;
#11250=CIRCLE ( 'NONE', #24550, 14.94182580522077330 ) ;
#11252=AXIS2_PLACEMENT_3D ( 'NONE', #24515, #384, #6984 ) ;
#11253=AXIS2_PLACEMENT_3D ( 'NONE', #9924, #23133, #7205 ) ;
#11258=AXIS2_PLACEMENT_3D ( 'NONE', #27207, #27476, #16723 ) ;
#11259=EDGE_LOOP ( 'NONE', ( #21802, #17183, #27767, #21812 ) ) ;
#11260=CARTESIAN_POINT ( 'NONE',  ( -125.2895325436294058, 200.2180533211638362, -13.00000000000000000 ) ) ;
#11263=ORIENTED_EDGE ( 'NONE', *, *, #4944, .F. ) ;
#11264=CARTESIAN_POINT ( 'NONE',  ( -7.915935011954262635, 131.1680411804064477, 16.32730855510867585 ) ) ;
#11268=CARTESIAN_POINT ( 'NONE',  ( -11.50561076655487014, 131.4941894630789250, -16.18874966886875200 ) ) ;
#11272=CARTESIAN_POINT ( 'NONE',  ( -180.0000000000000284, -70.00000000000004263, 70.00000000000001421 ) ) ;
#11278=AXIS2_PLACEMENT_3D ( 'NONE', #1443, #23423, #3732 ) ;
#11284=ORIENTED_EDGE ( 'NONE', *, *, #8028, .T. ) ;
#11288=ORIENTED_EDGE ( 'NONE', *, *, #24736, .T. ) ;
#11296=ORIENTED_EDGE ( 'NONE', *, *, #9503, .T. ) ;
#11298=AXIS2_PLACEMENT_3D ( 'NONE', #332, #6785, #20432 ) ;
#11299=ORIENTED_EDGE ( 'NONE', *, *, #24127, .T. ) ;
#11303=AXIS2_PLACEMENT_3D ( 'NONE', #4298, #19807, #565 ) ;
#11306=CARTESIAN_POINT ( 'NONE',  ( 96.65725945967196253, 241.1367295422483608, 10.34535073431436025 ) ) ;
#11307=EDGE_CURVE ( 'NONE', #19138, #12493, #14360, .T. ) ;
#11310=DIRECTION ( 'NONE',  ( -1.000000000000000000, -4.625929269271485914E-16, 0.000000000000000000 ) ) ;
#11312=DIRECTION ( 'NONE',  ( -1.000000000000000000, 8.673617379884073683E-17, 0.000000000000000000 ) ) ;
#11316=CARTESIAN_POINT ( 'NONE',  ( 46.79174272583949090, 194.0572550123460474, -13.00000000000000000 ) ) ;
#11319=ORIENTED_EDGE ( 'NONE', *, *, #5398, .T. ) ;
#11320=CARTESIAN_POINT ( 'NONE',  ( -37.82257053376181233, 71.03850157808263077, 99.00000000000000000 ) ) ;
#11321=CARTESIAN_POINT ( 'NONE',  ( 79.99999999999992895, 230.0000000000000284, 15.00000000000000000 ) ) ;
#11322=DIRECTION ( 'NONE',  ( 1.000000000000000000, 2.602085213965211135E-16, 0.000000000000000000 ) ) ;
#11327=LINE ( 'NONE', #20069, #15764 ) ;
#11329=CARTESIAN_POINT ( 'NONE',  ( -28.20602204321357576, 129.1555197674190083, -15.69110966610875657 ) ) ;
#11333=VERTEX_POINT ( 'NONE', #7604 ) ;
#11338=LINE ( 'NONE', #19412, #17083 ) ;
#11341=CARTESIAN_POINT ( 'NONE',  ( -20.30609983892121306, 129.6347424868099267, 15.47798682350772559 ) ) ;
#11342=ADVANCED_FACE ( 'NONE', ( #5578 ), #5434, .F. ) ;
#11343=CARTESIAN_POINT ( 'NONE',  ( -211.4394172367905185, 73.16162223722160718, 31.69164223700430938 ) ) ;
#11345=CARTESIAN_POINT ( 'NONE',  ( -160.0000000000000284, 59.99999999999994316, -45.00000000000000000 ) ) ;
#11347=DIRECTION ( 'NONE',  ( -1.000000000000000000, 0.000000000000000000, 0.000000000000000000 ) ) ;
#11348=EDGE_CURVE ( 'NONE', #22419, #12991, #18047, .T. ) ;
#11357=ORIENTED_EDGE ( 'NONE', *, *, #25525, .F. ) ;
#11360=DIRECTION ( 'NONE',  ( -0.000000000000000000, -0.000000000000000000, -1.000000000000000000 ) ) ;
#11361=CARTESIAN_POINT ( 'NONE',  ( -207.4088226029311102, 90.18755115757591057, -25.68075420788710161 ) ) ;
#11366=DIRECTION ( 'NONE',  ( 1.000000000000000000, 0.000000000000000000, 0.000000000000000000 ) ) ;
#11367=CARTESIAN_POINT ( 'NONE',  ( -156.1148230221487552, 122.3320249483163877, 20.71187466365067564 ) ) ;
#11368=VERTEX_POINT ( 'NONE', #22831 ) ;
#11369=VERTEX_POINT ( 'NONE', #1266 ) ;
#11371=TOROIDAL_SURFACE ( 'NONE', #28313, 14.95564396479129243, 3.532530335305412716 ) ;
#11376=CIRCLE ( 'NONE', #26037, 5.000000000000004441 ) ;
#11377=FACE_OUTER_BOUND ( 'NONE', #6260, .T. ) ;
#11380=LINE ( 'NONE', #22429, #7081 ) ;
#11382=CARTESIAN_POINT ( 'NONE',  ( -197.4451421692467079, 62.05060586452424332, -32.13681025546651426 ) ) ;
#11385=CARTESIAN_POINT ( 'NONE',  ( -236.8667578982872044, 138.8517089611673043, -5.000000000000004441 ) ) ;
#11392=CIRCLE ( 'NONE', #377, 6.025000000000002132 ) ;
#11396=EDGE_LOOP ( 'NONE', ( #8034, #18349, #11248, #5613, #10901, #9100, #5942, #7327, #17773 ) ) ;
#11401=DIRECTION ( 'NONE',  ( -0.000000000000000000, -0.000000000000000000, 1.000000000000000000 ) ) ;
#11406=EDGE_LOOP ( 'NONE', ( #16281, #10187, #23921, #14739 ) ) ;
#11407=CARTESIAN_POINT ( 'NONE',  ( 85.37729192592163940, 80.27798593822440409, 100.0000000000000142 ) ) ;
#11408=EDGE_LOOP ( 'NONE', ( #15711, #6010, #17746, #9532, #19559, #7924 ) ) ;
#11409=LINE ( 'NONE', #13146, #25820 ) ;
#11410=EDGE_CURVE ( 'NONE', #8764, #23283, #16232, .T. ) ;
#11416=CARTESIAN_POINT ( 'NONE',  ( -31.58116565127622621, 129.2285914189400557, -16.96974868353508370 ) ) ;
#11423=CARTESIAN_POINT ( 'NONE',  ( -40.40953891503691153, 0.000000000000000000, 100.0000000000000000 ) ) ;
#11426=ORIENTED_EDGE ( 'NONE', *, *, #28314, .T. ) ;
#11427=CARTESIAN_POINT ( 'NONE',  ( -221.9128906662286909, 61.41899577391679088, 10.11264670733106996 ) ) ;
#11431=FACE_OUTER_BOUND ( 'NONE', #6930, .T. ) ;
#11432=DIRECTION ( 'NONE',  ( 1.000000000000000000, 0.000000000000000000, 0.000000000000000000 ) ) ;
#11434=PLANE ( 'NONE',  #19798 ) ;
#11438=CARTESIAN_POINT ( 'NONE',  ( -216.5232992714898046, 71.44138874852887966, 24.86461342636829386 ) ) ;
#11439=VERTEX_POINT ( 'NONE', #13056 ) ;
#11441=AXIS2_PLACEMENT_3D ( 'NONE', #18125, #2596, #11532 ) ;
#11444=EDGE_LOOP ( 'NONE', ( #15862, #24534, #12312, #23658 ) ) ;
#11448=ADVANCED_FACE ( 'NONE', ( #21801 ), #21250, .T. ) ;
#11451=CARTESIAN_POINT ( 'NONE',  ( 105.2802062291979723, 246.7841820210157380, 28.66020632212674002 ) ) ;
#11452=AXIS2_PLACEMENT_3D ( 'NONE', #18311, #5084, #16441 ) ;
#11453=ADVANCED_FACE ( 'NONE', ( #28246 ), #5999, .F. ) ;
#11460=DIRECTION ( 'NONE',  ( 1.000000000000000000, -1.850371707708594366E-15, 0.000000000000000000 ) ) ;
#11463=LINE ( 'NONE', #24662, #23181 ) ;
#11465=LINE ( 'NONE', #26818, #3589 ) ;
#11466=CARTESIAN_POINT ( 'NONE',  ( 87.49999999999990052, 230.0000000000000284, 15.95262490344436657 ) ) ;
#11472=ORIENTED_EDGE ( 'NONE', *, *, #10974, .F. ) ;
#11475=CARTESIAN_POINT ( 'NONE',  ( 109.8651760759819354, 256.6126121034981225, -42.06544492442053240 ) ) ;
#11479=VECTOR ( 'NONE', #17631, 1000.000000000000000 ) ;
#11480=EDGE_CURVE ( 'NONE', #14873, #7514, #22177, .T. ) ;
#11481=VERTEX_POINT ( 'NONE', #17479 ) ;
#11482=ORIENTED_EDGE ( 'NONE', *, *, #16464, .T. ) ;
#11487=CARTESIAN_POINT ( 'NONE',  ( 0.000000000000000000, 0.000000000000000000, 83.00000000000001421 ) ) ;
#11490=CARTESIAN_POINT ( 'NONE',  ( -219.3331038875187176, 71.26739478976685405, 22.27060053768792258 ) ) ;
#11494=TOROIDAL_SURFACE ( 'NONE', #27080, 20.00000000000000355, 30.00000000000000000 ) ;
#11496=CARTESIAN_POINT ( 'NONE',  ( -228.9609126401460344, 91.22585804526202935, -13.24624710532488514 ) ) ;
#11498=CARTESIAN_POINT ( 'NONE',  ( -110.3221550338875687, 80.49308115506423178, 248.5795775865965993 ) ) ;
#11500=AXIS2_PLACEMENT_3D ( 'NONE', #14567, #23322, #3630 ) ;
#11502=CARTESIAN_POINT ( 'NONE',  ( -143.6428522700808230, 20.24192588826928585, 83.00000000000001421 ) ) ;
#11503=DIRECTION ( 'NONE',  ( 2.602085213965211135E-16, -1.000000000000000000, 0.000000000000000000 ) ) ;
#11506=ORIENTED_EDGE ( 'NONE', *, *, #17685, .T. ) ;
#11510=DIRECTION ( 'NONE',  ( 0.000000000000000000, 0.000000000000000000, 1.000000000000000000 ) ) ;
#11514=ORIENTED_EDGE ( 'NONE', *, *, #3474, .T. ) ;
#11517=AXIS2_PLACEMENT_3D ( 'NONE', #15194, #4677, #11310 ) ;
#11521=ORIENTED_EDGE ( 'NONE', *, *, #12776, .T. ) ;
#11524=AXIS2_PLACEMENT_3D ( 'NONE', #11320, #23961, #8592 ) ;
#11525=CARTESIAN_POINT ( 'NONE',  ( 20.92655468430566756, 155.3461090732848220, -13.00000000000000000 ) ) ;
#11527=CARTESIAN_POINT ( 'NONE',  ( -205.8198834057387785, 91.09083988932387399, 26.98970021333139613 ) ) ;
#11532=DIRECTION ( 'NONE',  ( -1.000000000000000000, -1.850371707708595056E-16, 0.000000000000000000 ) ) ;
#11533=CARTESIAN_POINT ( 'NONE',  ( -216.3679220181670360, 71.52319660855025063, -25.09443459582657709 ) ) ;
#11535=CIRCLE ( 'NONE', #27549, 1.999999999999993339 ) ;
#11539=DIRECTION ( 'NONE',  ( -1.000000000000000000, 0.000000000000000000, -0.000000000000000000 ) ) ;
#11543=CARTESIAN_POINT ( 'NONE',  ( -238.3574390336322040, 69.78222348740347059, 5.410870504207573539 ) ) ;
#11545=VERTEX_POINT ( 'NONE', #9447 ) ;
#11549=CARTESIAN_POINT ( 'NONE',  ( 100.5794065449870942, 118.1137289701970872, 81.24999999968734699 ) ) ;
#11550=CARTESIAN_POINT ( 'NONE',  ( -200.0701886854841689, 95.67681652162154649, -30.66283971992370638 ) ) ;
#11553=CARTESIAN_POINT ( 'NONE',  ( -189.8086322075389774, 92.49158130768422836, -13.00000000000000000 ) ) ;
#11560=CYLINDRICAL_SURFACE ( 'NONE', #2434, 5.000000000000004441 ) ;
#11565=CARTESIAN_POINT ( 'NONE',  ( 48.45469728424487244, 192.9461374953035033, -13.00000000000000000 ) ) ;
#11573=ORIENTED_EDGE ( 'NONE', *, *, #6331, .T. ) ;
#11574=CARTESIAN_POINT ( 'NONE',  ( -244.5479615644635487, 75.99513337129094737, 5.000000000000002665 ) ) ;
#11576=AXIS2_PLACEMENT_3D ( 'NONE', #4930, #5225, #5080 ) ;
#11578=CARTESIAN_POINT ( 'NONE',  ( -225.0350560533458690, 62.39407306348317661, -8.837833373942165949 ) ) ;
#11581=( NAMED_UNIT ( * ) SI_UNIT ( $, .STERADIAN. ) SOLID_ANGLE_UNIT ( ) );
#11583=ADVANCED_FACE ( 'NONE', ( #24373 ), #2905, .F. ) ;
#11584=AXIS2_PLACEMENT_3D ( 'NONE', #28039, #14863, #1903 ) ;
#11588=VECTOR ( 'NONE', #24785, 1000.000000000000000 ) ;
#11589=CARTESIAN_POINT ( 'NONE',  ( -92.70792463290142393, 134.7647503918266239, 15.46030987956200420 ) ) ;
#11591=EDGE_CURVE ( 'NONE', #26681, #4224, #5118, .T. ) ;
#11595=DIRECTION ( 'NONE',  ( 0.000000000000000000, -2.498359269027536814E-16, 1.000000000000000000 ) ) ;
#11599=CARTESIAN_POINT ( 'NONE',  ( 92.84236432024050600, 239.7913859916842227, 17.77233924293420841 ) ) ;
#11600=AXIS2_PLACEMENT_3D ( 'NONE', #16819, #3875, #21261 ) ;
#11601=CARTESIAN_POINT ( 'NONE',  ( 6.071532165918828775E-15, -70.00000000000002842, 100.0000000000000142 ) ) ;
#11607=CYLINDRICAL_SURFACE ( 'NONE', #4229, 30.00000000000000000 ) ;
#11609=CARTESIAN_POINT ( 'NONE',  ( 79.99999999999990052, 230.0000000000000284, -45.00000000000000000 ) ) ;
#11610=DIRECTION ( 'NONE',  ( 1.224646799147353207E-16, 1.000000000000000000, -0.000000000000000000 ) ) ;
#11616=DIRECTION ( 'NONE',  ( -0.000000000000000000, -0.000000000000000000, -1.000000000000000000 ) ) ;
#11622=CARTESIAN_POINT ( 'NONE',  ( 109.2808348379079462, 254.3902513977343176, -38.18180188067670855 ) ) ;
#11623=ORIENTED_EDGE ( 'NONE', *, *, #16944, .T. ) ;
#11629=ORIENTED_EDGE ( 'NONE', *, *, #11746, .F. ) ;
#11631=ORIENTED_EDGE ( 'NONE', *, *, #16555, .F. ) ;
#11632=CARTESIAN_POINT ( 'NONE',  ( 109.9999999999999432, 2.035408878479452500E-14, 45.00000000000000000 ) ) ;
#11637=VECTOR ( 'NONE', #13278, 1000.000000000000114 ) ;
#11640=CARTESIAN_POINT ( 'NONE',  ( -67.45133076571056563, 135.5141271316668394, -13.65948042911834470 ) ) ;
#11641=AXIS2_PLACEMENT_3D ( 'NONE', #28347, #15316, #4372 ) ;
#11642=CARTESIAN_POINT ( 'NONE',  ( 134.9999999999998579, 220.0000000000000284, -105.0000000000000284 ) ) ;
#11643=CARTESIAN_POINT ( 'NONE',  ( -203.1779787704217313, 93.05164332230201296, -28.77272332722132475 ) ) ;
#11645=CARTESIAN_POINT ( 'NONE',  ( -217.0264852877946566, -91.18033988749901653, 19.68410787789781580 ) ) ;
#11649=CARTESIAN_POINT ( 'NONE',  ( -8.429728459452139333, 132.5274614703484133, 14.39831780793436522 ) ) ;
#11653=VERTEX_POINT ( 'NONE', #11466 ) ;
#11654=ORIENTED_EDGE ( 'NONE', *, *, #13325, .T. ) ;
#11655=CARTESIAN_POINT ( 'NONE',  ( -203.2481855153402250, 92.57460631283319685, -29.78692811926998729 ) ) ;
#11657=ORIENTED_EDGE ( 'NONE', *, *, #16813, .T. ) ;
#11662=FACE_BOUND ( 'NONE', #28112, .T. ) ;
#11663=EDGE_CURVE ( 'NONE', #26863, #2835, #14377, .T. ) ;
#11664=CARTESIAN_POINT ( 'NONE',  ( -137.6856056883401322, 128.9562719326160334, 15.73927209086268064 ) ) ;
#11667=ORIENTED_EDGE ( 'NONE', *, *, #14879, .T. ) ;
#11672=CARTESIAN_POINT ( 'NONE',  ( -203.8967259421660572, 92.43987101052316291, 29.06044879621326160 ) ) ;
#11674=EDGE_CURVE ( 'NONE', #23784, #13456, #2385, .T. ) ;
#11676=FACE_OUTER_BOUND ( 'NONE', #11186, .T. ) ;
#11678=CARTESIAN_POINT ( 'NONE',  ( -195.0250397031994112, 62.90385929084195737, -38.63509848415888115 ) ) ;
#11680=EDGE_CURVE ( 'NONE', #11684, #21857, #23553, .T. ) ;
#11683=CARTESIAN_POINT ( 'NONE',  ( -160.0000000000000284, 59.99999999999994316, 15.00000000000000000 ) ) ;
#11684=VERTEX_POINT ( 'NONE', #26661 ) ;
#11686=CARTESIAN_POINT ( 'NONE',  ( -239.3181950532627980, 70.57797675262781922, 14.71337737012095559 ) ) ;
#11687=PLANE ( 'NONE',  #12658 ) ;
#11690=CARTESIAN_POINT ( 'NONE',  ( -119.0030847931093518, 214.2064521616283059, 5.000000000000002665 ) ) ;
#11691=DIRECTION ( 'NONE',  ( 0.000000000000000000, 0.000000000000000000, 1.000000000000000000 ) ) ;
#11696=CARTESIAN_POINT ( 'NONE',  ( 134.9999999999998579, 220.0000000000000284, 99.00000000000001421 ) ) ;
#11697=CARTESIAN_POINT ( 'NONE',  ( -215.4886702565631538, 139.8420026707765942, 14.99999999999998579 ) ) ;
#11700=EDGE_LOOP ( 'NONE', ( #8191, #10146, #471, #19586 ) ) ;
#11701=AXIS2_PLACEMENT_3D ( 'NONE', #15782, #11322, #9016 ) ;
#11702=LINE ( 'NONE', #20580, #13004 ) ;
#11705=CARTESIAN_POINT ( 'NONE',  ( -24.85022236748708124, 129.2502597746190816, -15.64835883620313517 ) ) ;
#11712=AXIS2_PLACEMENT_3D ( 'NONE', #13899, #22786, #7564 ) ;
#11713=EDGE_CURVE ( 'NONE', #7659, #25070, #24457, .T. ) ;
#11722=PLANE ( 'NONE',  #17877 ) ;
#11724=EDGE_LOOP ( 'NONE', ( #26453, #1731, #19590, #26644, #24315, #27182, #5727, #6893 ) ) ;
#11727=CIRCLE ( 'NONE', #7589, 14.94182580522077330 ) ;
#11728=EDGE_LOOP ( 'NONE', ( #13743, #10193, #16324, #22801 ) ) ;
#11732=ORIENTED_EDGE ( 'NONE', *, *, #13007, .T. ) ;
#11733=CARTESIAN_POINT ( 'NONE',  ( -17.24491960465746132, 80.97823757117562593, 95.00000000000000000 ) ) ;
#11734=ORIENTED_EDGE ( 'NONE', *, *, #22462, .F. ) ;
#11736=CIRCLE ( 'NONE', #10810, 50.00000000000000000 ) ;
#11740=CARTESIAN_POINT ( 'NONE',  ( -160.0000000000000284, 59.99999999999994316, 80.00000000000001421 ) ) ;
#11741=PLANE ( 'NONE',  #20427 ) ;
#11743=CARTESIAN_POINT ( 'NONE',  ( -210.7172313291012529, 103.7585653882801182, -5.000000000000004441 ) ) ;
#11746=EDGE_CURVE ( 'NONE', #23197, #1515, #2442, .T. ) ;
#11749=DIRECTION ( 'NONE',  ( -1.000000000000000000, 0.000000000000000000, -0.000000000000000000 ) ) ;
#11750=EDGE_CURVE ( 'NONE', #27752, #5346, #18484, .T. ) ;
#11751=DIRECTION ( 'NONE',  ( 1.000000000000000000, 0.000000000000000000, 0.000000000000000000 ) ) ;
#11756=ORIENTED_EDGE ( 'NONE', *, *, #17413, .T. ) ;
#11760=DIRECTION ( 'NONE',  ( 1.000000000000000000, -0.000000000000000000, -0.000000000000000000 ) ) ;
#11766=ORIENTED_EDGE ( 'NONE', *, *, #10775, .F. ) ;
#11768=ORIENTED_EDGE ( 'NONE', *, *, #24362, .F. ) ;
#11769=EDGE_LOOP ( 'NONE', ( #8942, #12646, #14166, #6792 ) ) ;
#11770=CARTESIAN_POINT ( 'NONE',  ( -158.6438865070083750, 121.2377615292502782, 20.46887661539795644 ) ) ;
#11771=DIRECTION ( 'NONE',  ( -0.000000000000000000, -0.000000000000000000, -1.000000000000000000 ) ) ;
#11773=EDGE_CURVE ( 'NONE', #4407, #2835, #27507, .T. ) ;
#11775=CARTESIAN_POINT ( 'NONE',  ( -97.72577305530073488, 134.4685796935967801, -15.51422881674326604 ) ) ;
#11778=CARTESIAN_POINT ( 'NONE',  ( -40.35425475217338942, 130.4208791593096350, 15.14570953137466880 ) ) ;
#11781=CARTESIAN_POINT ( 'NONE',  ( -144.7131007173674107, 126.7073428816716785, -16.81478254977324127 ) ) ;
#11782=EDGE_CURVE ( 'NONE', #10524, #12184, #27365, .T. ) ;
#11783=CARTESIAN_POINT ( 'NONE',  ( 79.99999999999995737, 93.29453619103988160, -96.96498881298317940 ) ) ;
#11784=DIRECTION ( 'NONE',  ( 1.000000000000000000, 0.000000000000000000, 0.000000000000000000 ) ) ;
#11788=CARTESIAN_POINT ( 'NONE',  ( 93.07270601802888166, 112.9533406971467429, 74.06249999970600584 ) ) ;
#11790=FACE_OUTER_BOUND ( 'NONE', #10180, .T. ) ;
#11791=CARTESIAN_POINT ( 'NONE',  ( -184.2178799556576791, 107.1030787669916435, 32.07408992895755517 ) ) ;
#11795=CARTESIAN_POINT ( 'NONE',  ( -218.6521670693695683, 86.22552751504353807, -19.45793375878209375 ) ) ;
#11796=DIRECTION ( 'NONE',  ( 0.000000000000000000, 0.000000000000000000, -1.000000000000000000 ) ) ;
#11797=ORIENTED_EDGE ( 'NONE', *, *, #13584, .F. ) ;
#11798=CIRCLE ( 'NONE', #21405, 89.71075545852265520 ) ;
#11803=VERTEX_POINT ( 'NONE', #3238 ) ;
#11805=FACE_OUTER_BOUND ( 'NONE', #15965, .T. ) ;
#11808=CARTESIAN_POINT ( 'NONE',  ( 134.9999999999998579, 220.0000000000000284, 100.0000000000000142 ) ) ;
#11810=CYLINDRICAL_SURFACE ( 'NONE', #415, 30.00000000000000000 ) ;
#11811=AXIS2_PLACEMENT_3D ( 'NONE', #18116, #13966, #22279 ) ;
#11812=CARTESIAN_POINT ( 'NONE',  ( -214.2313421017086341, 58.42887478691789482, -32.84133050939110632 ) ) ;
#11816=CARTESIAN_POINT ( 'NONE',  ( -180.0000000000000284, -40.00000000000004974, -25.00000000000000711 ) ) ;
#11821=CARTESIAN_POINT ( 'NONE',  ( -234.0991496467403579, 66.75367139654557036, 6.159314286176283737 ) ) ;
#11822=CARTESIAN_POINT ( 'NONE',  ( 124.9999999999998579, 220.0000000000000284, 90.00000000000002842 ) ) ;
#11823=ORIENTED_EDGE ( 'NONE', *, *, #4349, .F. ) ;
#11827=EDGE_CURVE ( 'NONE', #22340, #7786, #22204, .T. ) ;
#11828=CARTESIAN_POINT ( 'NONE',  ( 108.2273028572102760, 129.5338070841179672, 88.59375000028596503 ) ) ;
#11829=CARTESIAN_POINT ( 'NONE',  ( -210.0000000000000284, 59.99999999999994316, 15.00000000000000000 ) ) ;
#11831=AXIS2_PLACEMENT_3D ( 'NONE', #270, #15937, #13492 ) ;
#11833=CARTESIAN_POINT ( 'NONE',  ( -76.25760768171835480, 219.6666220619077876, -15.00000000000000000 ) ) ;
#11842=CARTESIAN_POINT ( 'NONE',  ( -28.20614712894950316, 129.1555222404294909, -15.69110854779580322 ) ) ;
#11844=EDGE_CURVE ( 'NONE', #18495, #21449, #18533, .T. ) ;
#11847=VECTOR ( 'NONE', #12629, 1000.000000000000000 ) ;
#11851=CARTESIAN_POINT ( 'NONE',  ( -218.8273392347297488, 140.3457761587515336, 14.99191580167116911 ) ) ;
#11855=EDGE_LOOP ( 'NONE', ( #17258, #4684, #14904, #2493 ) ) ;
#11856=DIRECTION ( 'NONE',  ( -0.000000000000000000, -0.000000000000000000, -1.000000000000000000 ) ) ;
#11862=ORIENTED_EDGE ( 'NONE', *, *, #14327, .T. ) ;
#11863=EDGE_CURVE ( 'NONE', #12495, #18743, #22355, .T. ) ;
#11864=CARTESIAN_POINT ( 'NONE',  ( -75.15023727777021634, 134.4794526767016691, 15.51172362355055867 ) ) ;
#11872=ORIENTED_EDGE ( 'NONE', *, *, #22390, .T. ) ;
#11878=CARTESIAN_POINT ( 'NONE',  ( 108.8501248000121109, 253.0299650810305536, 36.51570041463102001 ) ) ;
#11881=LINE ( 'NONE', #5254, #14237 ) ;
#11889=DIRECTION ( 'NONE',  ( 0.2759800118297804916, -0.9611633748070274041, 0.000000000000000000 ) ) ;
#11891=CARTESIAN_POINT ( 'NONE',  ( 113.9305603607155888, 212.0895489533244245, -97.95022080735121506 ) ) ;
#11893=VECTOR ( 'NONE', #2346, 1000.000000000000000 ) ;
#11894=AXIS2_PLACEMENT_3D ( 'NONE', #24766, #18301, #7385 ) ;
#11895=DIRECTION ( 'NONE',  ( 0.8516548651973804285, -0.5241030343220993704, 0.000000000000000000 ) ) ;
#11896=FACE_OUTER_BOUND ( 'NONE', #14933, .T. ) ;
#11897=FACE_OUTER_BOUND ( 'NONE', #2255, .T. ) ;
#11901=EDGE_LOOP ( 'NONE', ( #26393, #25660, #9603, #21159 ) ) ;
#11906=VECTOR ( 'NONE', #22766, 1000.000000000000000 ) ;
#11908=EDGE_LOOP ( 'NONE', ( #11667, #15745, #15033, #16073 ) ) ;
#11914=VECTOR ( 'NONE', #10040, 1000.000000000000000 ) ;
#11915=CARTESIAN_POINT ( 'NONE',  ( -248.1546605714623013, -91.18033988749901653, 0.000000000000000000 ) ) ;
#11919=CARTESIAN_POINT ( 'NONE',  ( -151.7715828776752574, 124.0909716950949644, -18.38260046643562617 ) ) ;
#11924=CIRCLE ( 'NONE', #17415, 1.999999999999997335 ) ;
#11927=CARTESIAN_POINT ( 'NONE',  ( 104.4199312700659448, 89.58810137561040676, -100.0000000000000142 ) ) ;
#11929=B_SPLINE_CURVE_WITH_KNOTS ( 'NONE', 3,
 ( #20172, #4504, #22043, #8974, #17305, #17731, #22332, #2641, #11427, #8557, #26478, #26065, #6808, #24631, #5229, #11993, #14288, #13872, #7674, #16304, #24777, #14149, #9412, #11574 ),
 .UNSPECIFIED., .F., .F.,
 ( 4, 2, 2, 2, 2, 2, 2, 2, 2, 2, 2, 4 ),
 ( 0.000000000000000000, 0.005275168248736577560, 0.007912752373104866774, 0.01055033649747315512, 0.01582550474620979947, 0.01846308887057816067, 0.02110067299494652188, 0.02637584124368318184, 0.02901342536805146324, 0.03165100949241975159, 0.03692617774115627971, 0.04220134598989280783 ),
 .UNSPECIFIED. ) ;
#11930=VERTEX_POINT ( 'NONE', #6107 ) ;
#11931=ORIENTED_EDGE ( 'NONE', *, *, #2793, .F. ) ;
#11935=AXIS2_PLACEMENT_3D ( 'NONE', #5711, #14484, #5989 ) ;
#11936=ORIENTED_EDGE ( 'NONE', *, *, #8822, .T. ) ;
#11941=ORIENTED_EDGE ( 'NONE', *, *, #5398, .F. ) ;
#11943=DIRECTION ( 'NONE',  ( 1.000000000000000000, 0.000000000000000000, 0.000000000000000000 ) ) ;
#11944=AXIS2_PLACEMENT_3D ( 'NONE', #16742, #21462, #21181 ) ;
#11945=DIRECTION ( 'NONE',  ( 1.000000000000000000, 0.000000000000000000, 0.000000000000000000 ) ) ;
#11946=CARTESIAN_POINT ( 'NONE',  ( 95.56988606615753667, 231.9897823149801752, -19.35215035236615932 ) ) ;
#11947=CIRCLE ( 'NONE', #7366, 79.71075545852265520 ) ;
#11949=CARTESIAN_POINT ( 'NONE',  ( 113.4999999999998863, 220.0000000000000284, -99.00000000000001421 ) ) ;
#11950=CARTESIAN_POINT ( 'NONE',  ( -217.0794644928006392, 71.41167302539398065, -24.35665452625710259 ) ) ;
#11959=CARTESIAN_POINT ( 'NONE',  ( -235.2766700735673169, 67.45978041260606517, 15.24953891110985182 ) ) ;
#11965=VECTOR ( 'NONE', #2603, 1000.000000000000000 ) ;
#11966=CARTESIAN_POINT ( 'NONE',  ( 101.7779539752123981, 119.2876405402088835, 100.0000000000000142 ) ) ;
#11978=LINE ( 'NONE', #24901, #25376 ) ;
#11979=VECTOR ( 'NONE', #26164, 1000.000000000000000 ) ;
#11982=CARTESIAN_POINT ( 'NONE',  ( -38.26643717395023003, 130.0143911579998530, -16.67725966943145366 ) ) ;
#11985=CARTESIAN_POINT ( 'NONE',  ( -207.5617036789550980, 75.42459176675926358, -44.71595801440848561 ) ) ;
#11991=DIRECTION ( 'NONE',  ( -0.000000000000000000, -0.000000000000000000, 1.000000000000000000 ) ) ;
#11993=CARTESIAN_POINT ( 'NONE',  ( -233.4149848405407681, 66.33036726544320061, 6.308275885109302372 ) ) ;
#11994=ORIENTED_EDGE ( 'NONE', *, *, #11844, .F. ) ;
#11995=EDGE_CURVE ( 'NONE', #23684, #8916, #8828, .T. ) ;
#11996=FACE_OUTER_BOUND ( 'NONE', #25506, .T. ) ;
#11997=LINE ( 'NONE', #20885, #943 ) ;
#12003=CARTESIAN_POINT ( 'NONE',  ( -86.44332993818018451, 134.8061491223789972, 15.45302073408354993 ) ) ;
#12004=CARTESIAN_POINT ( 'NONE',  ( 108.2138036696523642, 251.6610875895352137, 30.47597920753440803 ) ) ;
#12007=CARTESIAN_POINT ( 'NONE',  ( -143.6428522700808230, 20.24192588826928585, 80.00000000000001421 ) ) ;
#12012=ORIENTED_EDGE ( 'NONE', *, *, #26997, .F. ) ;
#12013=VERTEX_POINT ( 'NONE', #26475 ) ;
#12016=CARTESIAN_POINT ( 'NONE',  ( -229.2498027451139251, 132.0565166830976693, 15.00000000000000000 ) ) ;
#12018=CARTESIAN_POINT ( 'NONE',  ( 94.38583646783695258, 113.6320904521875548, -75.15625000023771918 ) ) ;
#12021=EDGE_CURVE ( 'NONE', #230, #22407, #6590, .T. ) ;
#12023=CARTESIAN_POINT ( 'NONE',  ( 109.9999999999999432, -100.0000000000000142, 70.00000000000001421 ) ) ;
#12025=CIRCLE ( 'NONE', #16171, 10.00000000000000888 ) ;
#12028=MECHANICAL_DESIGN_GEOMETRIC_PRESENTATION_REPRESENTATION('',(#7428),#15222);
#12038=CARTESIAN_POINT ( 'NONE',  ( 134.9999999999998579, 220.0000000000000284, 90.00000000000002842 ) ) ;
#12042=B_SPLINE_CURVE_WITH_KNOTS ( 'NONE', 3,
 ( #8627, #6609, #17377, #17099, #2427, #24275, #4445, #13230, #26140, #6464, #8912, #295, #13660, #5165, #20394, #11795, #26996, #5016, #6890, #9198, #24419, #20533, #15820, #22700, #724, #7038, #2865, #2574, #16101, #11655 ),
 .UNSPECIFIED., .F., .F.,
 ( 4, 2, 2, 2, 2, 2, 2, 2, 2, 2, 2, 2, 2, 2, 4 ),
 ( 1.076317285288624681E-15, 0.002329614659891489793, 0.003494421989836663748, 0.004659229319781837270, 0.009318458639562503601, 0.01164807329945279947, 0.01397768795934309534, 0.01630730261923338947, 0.01863691727912368534, 0.02329614659890428055, 0.02795537591868487923, 0.03028499057857521326, 0.03261460523846554382, 0.03494421989835588827, 0.03727383455824621883 ),
 .UNSPECIFIED. ) ;
#12043=ORIENTED_EDGE ( 'NONE', *, *, #9629, .F. ) ;
#12044=AXIS2_PLACEMENT_3D ( 'NONE', #3164, #20131, #2893 ) ;
#12046=ORIENTED_EDGE ( 'NONE', *, *, #12188, .F. ) ;
#12047=ORIENTED_EDGE ( 'NONE', *, *, #23294, .F. ) ;
#12049=DIRECTION ( 'NONE',  ( 1.000000000000000000, 0.000000000000000000, 0.000000000000000000 ) ) ;
#12052=AXIS2_PLACEMENT_3D ( 'NONE', #13302, #20180, #10858 ) ;
#12054=LINE ( 'NONE', #18646, #16703 ) ;
#12059=CARTESIAN_POINT ( 'NONE',  ( -219.0853371859187746, 87.86960372567372701, -16.90895988174265696 ) ) ;
#12067=TOROIDAL_SURFACE ( 'NONE', #24410, 68.83858790703926900, 2.000000000000000000 ) ;
#12078=ORIENTED_EDGE ( 'NONE', *, *, #7288, .T. ) ;
#12079=ORIENTED_EDGE ( 'NONE', *, *, #11069, .T. ) ;
#12085=CARTESIAN_POINT ( 'NONE',  ( -189.8086322075389774, 92.49158130768422836, -13.00000000000000000 ) ) ;
#12088=VECTOR ( 'NONE', #20501, 1000.000000000000000 ) ;
#12093=DIRECTION ( 'NONE',  ( 0.9960550913260673989, 0.000000000000000000, -0.08873699929240025375 ) ) ;
#12098=CARTESIAN_POINT ( 'NONE',  ( 179.9999999999999147, 0.000000000000000000, 100.0000000000000142 ) ) ;
#12103=CARTESIAN_POINT ( 'NONE',  ( -192.3996610505091951, 101.6547306301078493, 31.99652495868150837 ) ) ;
#12107=CIRCLE ( 'NONE', #7049, 30.00000000000000000 ) ;
#12109=ORIENTED_EDGE ( 'NONE', *, *, #18044, .T. ) ;
#12112=ORIENTED_EDGE ( 'NONE', *, *, #22353, .F. ) ;
#12118=CARTESIAN_POINT ( 'NONE',  ( -229.8316118350242334, 91.76664267010038145, 15.14942932049869917 ) ) ;
#12119=EDGE_LOOP ( 'NONE', ( #25853, #23053, #28182, #1766 ) ) ;
#12121=DIRECTION ( 'NONE',  ( -0.000000000000000000, -0.000000000000000000, 1.000000000000000000 ) ) ;
#12122=EDGE_CURVE ( 'NONE', #4186, #21416, #20313, .T. ) ;
#12123=ADVANCED_FACE ( 'NONE', ( #18171 ), #4791, .T. ) ;
#12128=DIRECTION ( 'NONE',  ( 0.000000000000000000, 0.000000000000000000, 1.000000000000000000 ) ) ;
#12129=CARTESIAN_POINT ( 'NONE',  ( -17.24491960465747553, 29.64876300893806516, 100.0000000000000000 ) ) ;
#12130=CARTESIAN_POINT ( 'NONE',  ( -199.1824292897938449, 96.09958175297150262, -31.38469581239659334 ) ) ;
#12131=VERTEX_POINT ( 'NONE', #2347 ) ;
#12133=EDGE_CURVE ( 'NONE', #21744, #14063, #2922, .T. ) ;
#12136=CARTESIAN_POINT ( 'NONE',  ( -217.6530433929989101, 140.9974892713794929, 15.00000000000000000 ) ) ;
#12139=FACE_OUTER_BOUND ( 'NONE', #16105, .T. ) ;
#12145=ORIENTED_EDGE ( 'NONE', *, *, #2049, .T. ) ;
#12147=CARTESIAN_POINT ( 'NONE',  ( 144.9999999999998863, 220.0000000000000284, 90.00000000000002842 ) ) ;
#12149=TOROIDAL_SURFACE ( 'NONE', #25898, 16.91094714394370158, 6.204828372381208546 ) ;
#12150=CARTESIAN_POINT ( 'NONE',  ( -248.1546605714623013, -91.18033988749901653, 16.91094714394370158 ) ) ;
#12154=ORIENTED_EDGE ( 'NONE', *, *, #13897, .T. ) ;
#12159=CARTESIAN_POINT ( 'NONE',  ( 109.9730600663563393, 258.3045051371393015, 43.53165882722885982 ) ) ;
#12161=CARTESIAN_POINT ( 'NONE',  ( 0.000000000000000000, 0.000000000000000000, -25.00000000000000000 ) ) ;
#12173=CARTESIAN_POINT ( 'NONE',  ( -11.05879453184508421, 130.1926234397373605, 16.63927220650600702 ) ) ;
#12176=CARTESIAN_POINT ( 'NONE',  ( 102.7211314862593099, 244.5532733014852909, -17.51403904043078441 ) ) ;
#12177=CARTESIAN_POINT ( 'NONE',  ( 25.96679874230557061, 85.42000967830594504, 99.51128369927819506 ) ) ;
#12181=DIRECTION ( 'NONE',  ( 0.000000000000000000, 0.000000000000000000, 1.000000000000000000 ) ) ;
#12182=ORIENTED_EDGE ( 'NONE', *, *, #27695, .T. ) ;
#12184=VERTEX_POINT ( 'NONE', #7394 ) ;
#12187=AXIS2_PLACEMENT_3D ( 'NONE', #27658, #1527, #16764 ) ;
#12188=EDGE_CURVE ( 'NONE', #4667, #13173, #22764, .T. ) ;
#12189=VERTEX_POINT ( 'NONE', #23179 ) ;
#12190=ADVANCED_FACE ( 'NONE', ( #5227 ), #27239, .F. ) ;
#12193=EDGE_LOOP ( 'NONE', ( #13987, #6161 ) ) ;
#12194=CARTESIAN_POINT ( 'NONE',  ( 115.1311745403714326, 209.3942962959461056, 98.75303131641565813 ) ) ;
#12195=LINE ( 'NONE', #24969, #15043 ) ;
#12197=CARTESIAN_POINT ( 'NONE',  ( -82.59029360989333668, 136.4857614611269412, -15.15915259372811619 ) ) ;
#12199=PLANE ( 'NONE',  #16009 ) ;
#12201=CARTESIAN_POINT ( 'NONE',  ( -107.3221550338875687, 22.24192588826928585, 83.00000000000001421 ) ) ;
#12202=CIRCLE ( 'NONE', #5758, 14.13483123440684253 ) ;
#12203=DIRECTION ( 'NONE',  ( -0.000000000000000000, -0.000000000000000000, 1.000000000000000000 ) ) ;
#12210=EDGE_CURVE ( 'NONE', #17211, #1493, #919, .T. ) ;
#12211=EDGE_CURVE ( 'NONE', #88, #17838, #12107, .T. ) ;
#12212=LINE ( 'NONE', #23389, #11914 ) ;
#12213=CARTESIAN_POINT ( 'NONE',  ( 109.6721745451464045, 96.60743919220468001, -100.0000000000000142 ) ) ;
#12217=VERTEX_POINT ( 'NONE', #23035 ) ;
#12221=VERTEX_POINT ( 'NONE', #14147 ) ;
#12224=ORIENTED_EDGE ( 'NONE', *, *, #13256, .F. ) ;
#12235=CARTESIAN_POINT ( 'NONE',  ( 79.99999999999991473, 140.0000000000000000, -15.00000000000000000 ) ) ;
#12236=CARTESIAN_POINT ( 'NONE',  ( 0.000000000000000000, 330.0000000000000000, 100.0000000000000142 ) ) ;
#12237=CARTESIAN_POINT ( 'NONE',  ( -222.0767938393173893, 71.52268347900216838, -20.18230367956038407 ) ) ;
#12239=SPHERICAL_SURFACE ( 'NONE', #12804, 30.00000000000000000 ) ;
#12240=CARTESIAN_POINT ( 'NONE',  ( -68.57415822541635464, 80.97823757117562593, 80.00000000000001421 ) ) ;
#12243=CARTESIAN_POINT ( 'NONE',  ( -195.0176442371520693, 99.46973748894193079, 32.52229805665887596 ) ) ;
#12245=EDGE_LOOP ( 'NONE', ( #11936, #10013 ) ) ;
#12249=ORIENTED_EDGE ( 'NONE', *, *, #1654, .T. ) ;
#12250=CARTESIAN_POINT ( 'NONE',  ( 106.3487426207432804, 91.82653269718771583, 100.0000000000000142 ) ) ;
#12252=ORIENTED_EDGE ( 'NONE', *, *, #9191, .T. ) ;
#12254=ORIENTED_EDGE ( 'NONE', *, *, #16876, .T. ) ;
#12255=CARTESIAN_POINT ( 'NONE',  ( 90.17595424773269031, 111.7661400908363731, -72.22656249986501109 ) ) ;
#12257=CARTESIAN_POINT ( 'NONE',  ( 94.28021150171387887, 231.3879905774517454, 18.61204911420563590 ) ) ;
#12261=CARTESIAN_POINT ( 'NONE',  ( 100.8904249506254018, 86.57652225510716448, 100.0000000000000142 ) ) ;
#12263=TOROIDAL_SURFACE ( 'NONE', #22341, 21.49999999999998224, 1.000000000000000000 ) ;
#12264=FACE_OUTER_BOUND ( 'NONE', #19083, .T. ) ;
#12265=DIRECTION ( 'NONE',  ( 1.000000000000000000, 0.000000000000000000, 0.000000000000000000 ) ) ;
#12271=ORIENTED_EDGE ( 'NONE', *, *, #11101, .T. ) ;
#12273=DIRECTION ( 'NONE',  ( 1.000000000000000000, 0.000000000000000000, 0.000000000000000000 ) ) ;
#12275=CARTESIAN_POINT ( 'NONE',  ( -221.3650667873343139, -91.18033988749901653, 0.000000000000000000 ) ) ;
#12279=DIRECTION ( 'NONE',  ( 1.530283246943720875E-16, -1.000000000000000000, 0.000000000000000000 ) ) ;
#12281=CARTESIAN_POINT ( 'NONE',  ( -221.3650667873343139, -91.18033988749901653, 0.000000000000000000 ) ) ;
#12293=EDGE_CURVE ( 'NONE', #17838, #17982, #16716, .T. ) ;
#12295=ORIENTED_EDGE ( 'NONE', *, *, #26454, .T. ) ;
#12302=CARTESIAN_POINT ( 'NONE',  ( -226.9194690495523332, 131.5555540326517985, 13.00000000000000000 ) ) ;
#12307=DIRECTION ( 'NONE',  ( 1.321694076934710155E-16, -1.000000000000000000, 0.000000000000000000 ) ) ;
#12312=ORIENTED_EDGE ( 'NONE', *, *, #21657, .T. ) ;
#12314=CARTESIAN_POINT ( 'NONE',  ( 94.61298883701873308, 240.5205049088891371, -8.728139299124077155 ) ) ;
#12316=DIRECTION ( 'NONE',  ( 0.000000000000000000, 0.000000000000000000, -1.000000000000000000 ) ) ;
#12325=CIRCLE ( 'NONE', #1730, 22.49999999999999289 ) ;
#12328=CARTESIAN_POINT ( 'NONE',  ( -97.91344426061895945, 136.1593943688571926, 15.19680741217146824 ) ) ;
#12330=ORIENTED_EDGE ( 'NONE', *, *, #142, .F. ) ;
#12333=SPHERICAL_SURFACE ( 'NONE', #9143, 30.00000000000000000 ) ;
#12338=VECTOR ( 'NONE', #5117, 1000.000000000000000 ) ;
#12346=ORIENTED_EDGE ( 'NONE', *, *, #20942, .F. ) ;
#12347=ADVANCED_FACE ( 'NONE', ( #10386 ), #1476, .F. ) ;
#12348=CARTESIAN_POINT ( 'NONE',  ( -42.54774212103357200, -18.98692024693243852, 99.90775213666447030 ) ) ;
#12351=ORIENTED_EDGE ( 'NONE', *, *, #17845, .F. ) ;
#12353=CIRCLE ( 'NONE', #16910, 10.00000000000000888 ) ;
#12358=CIRCLE ( 'NONE', #13737, 24.07986109634097005 ) ;
#12359=AXIS2_PLACEMENT_3D ( 'NONE', #14805, #21398, #1711 ) ;
#12364=DIRECTION ( 'NONE',  ( -1.000000000000000000, -2.602085213965211135E-16, -0.000000000000000000 ) ) ;
#12381=DIRECTION ( 'NONE',  ( 0.000000000000000000, 0.000000000000000000, -1.000000000000000000 ) ) ;
#12384=VECTOR ( 'NONE', #6301, 1000.000000000000000 ) ;
#12387=EDGE_LOOP ( 'NONE', ( #11732, #12577, #21885, #5524 ) ) ;
#12392=CARTESIAN_POINT ( 'NONE',  ( 85.37729192592163940, 80.27798593822440409, 100.0000000000000142 ) ) ;
#12394=CARTESIAN_POINT ( 'NONE',  ( 65.00000000000000000, -120.0000000000000995, -75.99999999999998579 ) ) ;
#12401=VERTEX_POINT ( 'NONE', #28029 ) ;
#12402=CARTESIAN_POINT ( 'NONE',  ( 117.1152841538673073, 116.0550883417529207, 100.0000000000000142 ) ) ;
#12405=DIRECTION ( 'NONE',  ( 0.000000000000000000, 0.000000000000000000, 1.000000000000000000 ) ) ;
#12406=DIRECTION ( 'NONE',  ( -0.9654425086906591735, 0.2448377981135679837, 0.08930405941493638200 ) ) ;
#12414=DIRECTION ( 'NONE',  ( 0.000000000000000000, 0.000000000000000000, 1.000000000000000000 ) ) ;
#12423=CARTESIAN_POINT ( 'NONE',  ( -195.0245025301963722, 99.69673397905764034, 31.69035508706320670 ) ) ;
#12426=VERTEX_POINT ( 'NONE', #27889 ) ;
#12428=ORIENTED_EDGE ( 'NONE', *, *, #18408, .T. ) ;
#12433=DIRECTION ( 'NONE',  ( 1.000000000000000000, -0.000000000000000000, -0.000000000000000000 ) ) ;
#12443=CARTESIAN_POINT ( 'NONE',  ( 145.9999999999998863, 220.0000000000000284, -100.0000000000000142 ) ) ;
#12444=CARTESIAN_POINT ( 'NONE',  ( -225.7036482868739427, -91.18033988749901653, 0.000000000000000000 ) ) ;
#12446=CARTESIAN_POINT ( 'NONE',  ( -220.9458266506740927, 71.36862438102546946, -20.99673689147822486 ) ) ;
#12447=DIRECTION ( 'NONE',  ( -0.9586565047779720405, -0.2845658198851049314, -0.000000000000000000 ) ) ;
#12453=ADVANCED_FACE ( 'NONE', ( #22147 ), #22003, .F. ) ;
#12455=EDGE_CURVE ( 'NONE', #17982, #7779, #17549, .T. ) ;
#12467=CARTESIAN_POINT ( 'NONE',  ( -86.54597169974458382, 136.4599361015214072, 15.16231345941510433 ) ) ;
#12468=VERTEX_POINT ( 'NONE', #21867 ) ;
#12470=CARTESIAN_POINT ( 'NONE',  ( 112.8464227643159035, 224.0613302109408380, 96.99047740776141779 ) ) ;
#12476=EDGE_CURVE ( 'NONE', #2290, #2012, #13053, .T. ) ;
#12477=AXIS2_PLACEMENT_3D ( 'NONE', #17345, #19360, #8454 ) ;
#12481=DIRECTION ( 'NONE',  ( 1.000000000000000000, 0.000000000000000000, 0.000000000000000000 ) ) ;
#12482=CARTESIAN_POINT ( 'NONE',  ( -221.2010484699854089, 88.15128852653619163, -15.79399925067323451 ) ) ;
#12484=CARTESIAN_POINT ( 'NONE',  ( -224.8943620750042669, 87.10469160093204266, 16.59178732851365012 ) ) ;
#12490=DIRECTION ( 'NONE',  ( -0.6533458216954761699, 0.7570595995514904919, 0.000000000000000000 ) ) ;
#12491=DIRECTION ( 'NONE',  ( -1.000000000000000000, 0.000000000000000000, 0.000000000000000000 ) ) ;
#12493=VERTEX_POINT ( 'NONE', #17411 ) ;
#12494=CARTESIAN_POINT ( 'NONE',  ( 100.8286702512460664, 242.7181571222803882, -23.14229345413746231 ) ) ;
#12495=VERTEX_POINT ( 'NONE', #17695 ) ;
#12496=ORIENTED_EDGE ( 'NONE', *, *, #22723, .F. ) ;
#12500=EDGE_LOOP ( 'NONE', ( #16267, #28318, #22125, #13658 ) ) ;
#12504=DIRECTION ( 'NONE',  ( -1.000000000000000000, 0.000000000000000000, 0.000000000000000000 ) ) ;
#12505=CARTESIAN_POINT ( 'NONE',  ( 109.5123651676572933, 253.5802735191045656, -39.43351859324057784 ) ) ;
#12507=DIRECTION ( 'NONE',  ( 3.469446951953614189E-16, -1.000000000000000000, 0.000000000000000000 ) ) ;
#12508=EDGE_CURVE ( 'NONE', #22333, #7588, #2175, .T. ) ;
#12513=CARTESIAN_POINT ( 'NONE',  ( -209.1631124584775705, 74.45386818103241922, -36.43774469185622422 ) ) ;
#12514=VECTOR ( 'NONE', #1415, 1000.000000000000000 ) ;
#12516=DIRECTION ( 'NONE',  ( -0.000000000000000000, -0.000000000000000000, 1.000000000000000000 ) ) ;
#12520=CARTESIAN_POINT ( 'NONE',  ( -192.4212042216159944, 101.6389693173133253, 32.42120117541568192 ) ) ;
#12523=CARTESIAN_POINT ( 'NONE',  ( 134.9999999999998579, 220.0000000000000284, 99.00000000000001421 ) ) ;
#12529=TOROIDAL_SURFACE ( 'NONE', #22617, 19.29759039828519818, 4.355764593064427537 ) ;
#12530=CARTESIAN_POINT ( 'NONE',  ( 79.99999999999991473, 80.00000000000001421, 100.0000000000000142 ) ) ;
#12533=VECTOR ( 'NONE', #25989, 1000.000000000000000 ) ;
#12535=EDGE_CURVE ( 'NONE', #15146, #2640, #16265, .T. ) ;
#12540=CARTESIAN_POINT ( 'NONE',  ( -160.8326600028555902, 120.2355194873575073, -21.37420696376537776 ) ) ;
#12543=EDGE_LOOP ( 'NONE', ( #17147, #14335, #3925, #25683 ) ) ;
#12544=CARTESIAN_POINT ( 'NONE',  ( -160.0000000000000284, 59.99999999999994316, 100.0000000000000142 ) ) ;
#12551=CARTESIAN_POINT ( 'NONE',  ( -187.2855578089503013, 105.0618758895388254, -32.61441565267596587 ) ) ;
#12555=DIRECTION ( 'NONE',  ( 0.000000000000000000, 0.000000000000000000, 1.000000000000000000 ) ) ;
#12557=AXIS2_PLACEMENT_3D ( 'NONE', #19641, #17338, #23529 ) ;
#12559=VERTEX_POINT ( 'NONE', #4466 ) ;
#12563=CARTESIAN_POINT ( 'NONE',  ( -31.71380104971701641, 128.0308663543026739, -17.49104459963816893 ) ) ;
#12564=CARTESIAN_POINT ( 'NONE',  ( -215.9344744818343429, 87.83801675608414428, 18.87891717999596253 ) ) ;
#12566=CARTESIAN_POINT ( 'NONE',  ( -236.8177751472017007, 82.33896643611701904, 15.00000000000000000 ) ) ;
#12569=CARTESIAN_POINT ( 'NONE',  ( 109.9895023066273723, 259.3387059742136671, 43.85457132728548402 ) ) ;
#12571=AXIS2_PLACEMENT_3D ( 'NONE', #21679, #1992, #2409 ) ;
#12577=ORIENTED_EDGE ( 'NONE', *, *, #21100, .F. ) ;
#12580=EDGE_CURVE ( 'NONE', #18325, #6225, #24593, .T. ) ;
#12586=CARTESIAN_POINT ( 'NONE',  ( 6.071532165918828775E-15, -70.00000000000002842, -70.00000000000001421 ) ) ;
#12589=CARTESIAN_POINT ( 'NONE',  ( -235.8599852676175601, 67.86969485657397172, -15.13802962878465763 ) ) ;
#12594=CARTESIAN_POINT ( 'NONE',  ( 115.1311745403725553, 230.6057037040560544, -98.75303131641626919 ) ) ;
#12597=DIRECTION ( 'NONE',  ( 1.000000000000000000, 0.000000000000000000, 0.000000000000000000 ) ) ;
#12598=CARTESIAN_POINT ( 'NONE',  ( 105.0440993989431604, 246.7662739188597527, -21.68283346401344147 ) ) ;
#12602=AXIS2_PLACEMENT_3D ( 'NONE', #20279, #2313, #2605 ) ;
#12604=CARTESIAN_POINT ( 'NONE',  ( -232.6158302464227461, 77.06694679626161815, 15.48771011243863427 ) ) ;
#12607=ORIENTED_EDGE ( 'NONE', *, *, #4319, .F. ) ;
#12609=DIRECTION ( 'NONE',  ( 1.000000000000000000, 0.000000000000000000, 0.000000000000000000 ) ) ;
#12611=EDGE_CURVE ( 'NONE', #15968, #1390, #7992, .T. ) ;
#12612=EDGE_LOOP ( 'NONE', ( #3954, #5839, #7656, #20820 ) ) ;
#12613=CARTESIAN_POINT ( 'NONE',  ( -175.0000000000000000, -120.0000000000001847, -69.99999999999998579 ) ) ;
#12620=CARTESIAN_POINT ( 'NONE',  ( -149.4366259724174597, 124.9893150903529886, -17.81052309126764754 ) ) ;
#12624=CARTESIAN_POINT ( 'NONE',  ( 28.11522373509561845, -43.91897918210346319, 99.74458822874382236 ) ) ;
#12625=CARTESIAN_POINT ( 'NONE',  ( -217.2920046552164308, 87.79525986223114842, -17.98591562465373173 ) ) ;
#12627=CARTESIAN_POINT ( 'NONE',  ( -211.1110268895868671, 87.67313158452103039, 24.45088837201200604 ) ) ;
#12629=DIRECTION ( 'NONE',  ( -1.000000000000000000, -0.000000000000000000, -0.000000000000000000 ) ) ;
#12631=ORIENTED_EDGE ( 'NONE', *, *, #5945, .F. ) ;
#12633=FACE_OUTER_BOUND ( 'NONE', #28395, .T. ) ;
#12635=VERTEX_POINT ( 'NONE', #6004 ) ;
#12637=VECTOR ( 'NONE', #9147, 1000.000000000000000 ) ;
#12639=CARTESIAN_POINT ( 'NONE',  ( 91.45931183161239630, 239.6823639899074863, -17.19464119471857089 ) ) ;
#12645=EDGE_CURVE ( 'NONE', #17385, #3706, #14895, .T. ) ;
#12646=ORIENTED_EDGE ( 'NONE', *, *, #14801, .T. ) ;
#12652=CARTESIAN_POINT ( 'NONE',  ( -230.8916957670046486, 130.8330661503599117, 5.000000000000002665 ) ) ;
#12658=AXIS2_PLACEMENT_3D ( 'NONE', #13986, #16270, #18555 ) ;
#12660=CYLINDRICAL_SURFACE ( 'NONE', #19385, 19.99999999999998934 ) ;
#12664=DIRECTION ( 'NONE',  ( 1.000000000000000000, 8.313992734408275564E-16, 0.000000000000000000 ) ) ;
#12665=ORIENTED_EDGE ( 'NONE', *, *, #15982, .T. ) ;
#12669=CIRCLE ( 'NONE', #2103, 68.83858790703926900 ) ;
#12672=AXIS2_PLACEMENT_3D ( 'NONE', #9577, #7420, #24659 ) ;
#12673=AXIS2_PLACEMENT_3D ( 'NONE', #18283, #22736, #20570 ) ;
#12674=ORIENTED_EDGE ( 'NONE', *, *, #5004, .T. ) ;
#12676=CARTESIAN_POINT ( 'NONE',  ( 119.9999999987673220, 136.1131920015923811, 100.0000000000000142 ) ) ;
#12679=AXIS2_PLACEMENT_3D ( 'NONE', #20522, #24840, #22542 ) ;
#12680=ORIENTED_EDGE ( 'NONE', *, *, #24395, .T. ) ;
#12682=CARTESIAN_POINT ( 'NONE',  ( 101.6154567033504748, 236.6169251702747545, 24.17999014744245656 ) ) ;
#12684=VERTEX_POINT ( 'NONE', #27024 ) ;
#12689=CARTESIAN_POINT ( 'NONE',  ( -107.3221550338875687, 69.54464929955099706, 80.00000000000001421 ) ) ;
#12692=CARTESIAN_POINT ( 'NONE',  ( -68.57415822541635464, 24.64876300893806160, 95.00000000000000000 ) ) ;
#12694=ORIENTED_EDGE ( 'NONE', *, *, #9629, .T. ) ;
#12695=CARTESIAN_POINT ( 'NONE',  ( 79.99999999999994316, 80.00000000000001421, 100.0000000000000142 ) ) ;
#12701=ADVANCED_FACE ( 'NONE', ( #12633 ), #22859, .T. ) ;
#12711=CARTESIAN_POINT ( 'NONE',  ( -189.6026171856603355, 103.6733896582188663, -32.02322945567066625 ) ) ;
#12712=EDGE_LOOP ( 'NONE', ( #15554, #4949, #24625, #20299, #9901, #7409, #3637, #17898, #16548 ) ) ;
#12713=AXIS2_PLACEMENT_3D ( 'NONE', #20294, #7083, #5059 ) ;
#12722=DIRECTION ( 'NONE',  ( -1.000000000000000000, -2.312964634635742957E-16, 0.000000000000000000 ) ) ;
#12723=CARTESIAN_POINT ( 'NONE',  ( -141.6428522700808230, 17.24192588826928585, 80.00000000000001421 ) ) ;
#12724=LINE ( 'NONE', #16602, #467 ) ;
#12727=CARTESIAN_POINT ( 'NONE',  ( -228.8737713456793017, 63.73618850397832603, -17.32239903714437901 ) ) ;
#12730=CYLINDRICAL_SURFACE ( 'NONE', #25286, 21.59849023212046149 ) ;
#12731=LINE ( 'NONE', #2071, #10496 ) ;
#12732=CARTESIAN_POINT ( 'NONE',  ( 112.4997598733875463, 219.4957354009212622, -96.61410599988441561 ) ) ;
#12736=CYLINDRICAL_SURFACE ( 'NONE', #10488, 178.6603051211419597 ) ;
#12745=ORIENTED_EDGE ( 'NONE', *, *, #25500, .F. ) ;
#12750=CARTESIAN_POINT ( 'NONE',  ( -42.65532241761713550, 131.0044336801081784, 16.34779397420838265 ) ) ;
#12753=FACE_BOUND ( 'NONE', #6867, .T. ) ;
#12755=CARTESIAN_POINT ( 'NONE',  ( -152.1205167745108326, 122.9384117505879885, -20.31814181434752342 ) ) ;
#12758=CARTESIAN_POINT ( 'NONE',  ( -122.8178735660354306, 132.7857580173457279, -15.82982010538316153 ) ) ;
#12761=CARTESIAN_POINT ( 'NONE',  ( -223.8285381716049187, 88.79728400276415812, -16.70700657864426475 ) ) ;
#12763=CARTESIAN_POINT ( 'NONE',  ( -216.0423832044228902, 86.42328519517769791, 21.02196399024839479 ) ) ;
#12764=DIRECTION ( 'NONE',  ( 0.000000000000000000, 0.000000000000000000, -1.000000000000000000 ) ) ;
#12765=FACE_OUTER_BOUND ( 'NONE', #11037, .T. ) ;
#12770=DIRECTION ( 'NONE',  ( -0.000000000000000000, -0.000000000000000000, 1.000000000000000000 ) ) ;
#12775=EDGE_CURVE ( 'NONE', #11684, #15436, #1691, .T. ) ;
#12776=EDGE_CURVE ( 'NONE', #22333, #13234, #13335, .T. ) ;
#12777=CARTESIAN_POINT ( 'NONE',  ( 93.75109487930336627, 231.1752187890907351, -18.33298295918092435 ) ) ;
#12779=VERTEX_POINT ( 'NONE', #6575 ) ;
#12785=CARTESIAN_POINT ( 'NONE',  ( -175.0000000000000000, -120.0000000000001847, -75.99999999999998579 ) ) ;
#12786=ADVANCED_FACE ( 'NONE', ( #15062 ), #24107, .T. ) ;
#12791=EDGE_CURVE ( 'NONE', #10678, #22419, #28109, .T. ) ;
#12795=AXIS2_PLACEMENT_3D ( 'NONE', #28212, #12597, #21336 ) ;
#12796=CARTESIAN_POINT ( 'NONE',  ( -31.54256950484095867, 129.2255411891219978, 16.97092939656602795 ) ) ;
#12797=CARTESIAN_POINT ( 'NONE',  ( 20.92655468430566756, 155.3461090732848220, 12.99999999999999822 ) ) ;
#12798=DIRECTION ( 'NONE',  ( 0.000000000000000000, 0.000000000000000000, 1.000000000000000000 ) ) ;
#12800=FACE_OUTER_BOUND ( 'NONE', #15751, .T. ) ;
#12802=CARTESIAN_POINT ( 'NONE',  ( -162.3832362631574426, 119.5298884965290682, 23.01156641556860549 ) ) ;
#12804=AXIS2_PLACEMENT_3D ( 'NONE', #23280, #23142, #5886 ) ;
#12808=CARTESIAN_POINT ( 'NONE',  ( -160.0000000000000284, 109.9999999999999432, 100.0000000000000142 ) ) ;
#12812=ORIENTED_EDGE ( 'NONE', *, *, #15839, .F. ) ;
#12813=CARTESIAN_POINT ( 'NONE',  ( 88.58553289616391169, 111.2425746093149002, 99.99999999998919975 ) ) ;
#12814=DIRECTION ( 'NONE',  ( -0.000000000000000000, -0.000000000000000000, -1.000000000000000000 ) ) ;
#12817=CARTESIAN_POINT ( 'NONE',  ( 109.9999999984624850, 137.0808454111539447, -100.0000000001515872 ) ) ;
#12818=CARTESIAN_POINT ( 'NONE',  ( 95.14885519176667117, 231.7800616880396092, 19.10095409356435070 ) ) ;
#12822=CARTESIAN_POINT ( 'NONE',  ( -226.3114843550383171, 89.76160135746334845, 15.90464330981206054 ) ) ;
#12824=DIRECTION ( 'NONE',  ( 1.000000000000000000, 8.570722872813602225E-16, 0.000000000000000000 ) ) ;
#12828=AXIS2_PLACEMENT_3D ( 'NONE', #5599, #23130, #11945 ) ;
#12829=DIRECTION ( 'NONE',  ( 0.5804519453834686704, -0.8142945039115434547, 0.000000000000000000 ) ) ;
#12830=EDGE_CURVE ( 'NONE', #7854, #11439, #17193, .T. ) ;
#12832=CARTESIAN_POINT ( 'NONE',  ( -160.0000000000000284, 59.99999999999994316, 80.00000000000001421 ) ) ;
#12839=EDGE_CURVE ( 'NONE', #9431, #17312, #4326, .T. ) ;
#12840=DIRECTION ( 'NONE',  ( -0.000000000000000000, -0.000000000000000000, 1.000000000000000000 ) ) ;
#12841=DIRECTION ( 'NONE',  ( 0.000000000000000000, 0.000000000000000000, 1.000000000000000000 ) ) ;
#12842=CARTESIAN_POINT ( 'NONE',  ( -211.7675867465070496, 88.48852952219857571, 21.99030125636233635 ) ) ;
#12843=ORIENTED_EDGE ( 'NONE', *, *, #18839, .T. ) ;
#12846=AXIS2_PLACEMENT_3D ( 'NONE', #2937, #22480, #24635 ) ;
#12849=CARTESIAN_POINT ( 'NONE',  ( -183.1579956025468618, 108.0230262084780435, -31.30096897312795434 ) ) ;
#12852=VECTOR ( 'NONE', #13043, 1000.000000000000000 ) ;
#12864=TOROIDAL_SURFACE ( 'NONE', #24329, 18.46313063346208239, 2.000000000000000000 ) ;
#12867=CARTESIAN_POINT ( 'NONE',  ( -233.4632575733478745, 77.89441575050611277, -15.30815287833104854 ) ) ;
#12876=DIRECTION ( 'NONE',  ( 1.541976423090495387E-16, -1.000000000000000000, 0.000000000000000000 ) ) ;
#12877=CARTESIAN_POINT ( 'NONE',  ( 179.9999999999999147, 330.0000000000000000, -84.99999999999997158 ) ) ;
#12880=ORIENTED_EDGE ( 'NONE', *, *, #13000, .T. ) ;
#12884=ORIENTED_EDGE ( 'NONE', *, *, #11001, .F. ) ;
#12892=ORIENTED_EDGE ( 'NONE', *, *, #4213, .F. ) ;
#12895=DIRECTION ( 'NONE',  ( -1.000000000000000000, 0.000000000000000000, 0.000000000000000000 ) ) ;
#12900=CARTESIAN_POINT ( 'NONE',  ( -160.0000000000000284, 59.99999999999994316, 70.00000000000001421 ) ) ;
#12902=CARTESIAN_POINT ( 'NONE',  ( -225.0668536777367308, 87.15822506044099782, -16.53154426491069628 ) ) ;
#12911=VECTOR ( 'NONE', #21402, 1000.000000000000000 ) ;
#12912=CARTESIAN_POINT ( 'NONE',  ( 117.3825211564071225, 140.0000000000000284, 99.73972676668319082 ) ) ;
#12913=CARTESIAN_POINT ( 'NONE',  ( -175.0000000000000000, -120.0250000000001762, 70.00000000000001421 ) ) ;
#12915=ORIENTED_EDGE ( 'NONE', *, *, #7748, .F. ) ;
#12916=CARTESIAN_POINT ( 'NONE',  ( 88.05061285013169936, 239.8951213614055007, -16.09479252966708529 ) ) ;
#12918=CARTESIAN_POINT ( 'NONE',  ( -42.53273978471831640, 130.9733465240572627, -14.93735646117640492 ) ) ;
#12925=VECTOR ( 'NONE', #17451, 1000.000000000000000 ) ;
#12928=DIRECTION ( 'NONE',  ( -0.5975062131282553590, 0.8018642810807399268, 0.000000000000000000 ) ) ;
#12930=ADVANCED_FACE ( 'NONE', ( #24816 ), #18068, .T. ) ;
#12940=CARTESIAN_POINT ( 'NONE',  ( -175.8417606860892874, 246.9430296707336652, 12.99999999999999822 ) ) ;
#12945=CARTESIAN_POINT ( 'NONE',  ( -185.8734447760280091, 106.0260592552631635, 32.44447814219098802 ) ) ;
#12948=ORIENTED_EDGE ( 'NONE', *, *, #406, .F. ) ;
#12952=CARTESIAN_POINT ( 'NONE',  ( -225.9729034214362855, 132.4331356209112300, -12.99353264133693742 ) ) ;
#12957=CARTESIAN_POINT ( 'NONE',  ( 79.99999999999991473, 110.0000000000000142, -100.0000000000000142 ) ) ;
#12964=CARTESIAN_POINT ( 'NONE',  ( -227.5151209178948477, 90.37154496853476360, 15.60286242741050700 ) ) ;
#12965=ORIENTED_EDGE ( 'NONE', *, *, #21453, .T. ) ;
#12966=CIRCLE ( 'NONE', #6528, 16.07743405327025243 ) ;
#12967=CARTESIAN_POINT ( 'NONE',  ( -220.5365384948381120, 71.33200643684088504, 21.30906822952360358 ) ) ;
#12973=CARTESIAN_POINT ( 'NONE',  ( -248.1546605714623013, -91.18033988749901653, 0.000000000000000000 ) ) ;
#12977=DIRECTION ( 'NONE',  ( 0.000000000000000000, 0.000000000000000000, -1.000000000000000000 ) ) ;
#12979=DIRECTION ( 'NONE',  ( 1.000000000000000000, 0.000000000000000000, 0.000000000000000000 ) ) ;
#12981=ORIENTED_EDGE ( 'NONE', *, *, #8195, .F. ) ;
#12982=VECTOR ( 'NONE', #27867, 1000.000000000000000 ) ;
#12983=FACE_OUTER_BOUND ( 'NONE', #4588, .T. ) ;
#12985=DIRECTION ( 'NONE',  ( 0.000000000000000000, 0.000000000000000000, 1.000000000000000000 ) ) ;
#12986=DIRECTION ( 'NONE',  ( 1.000000000000000000, 0.000000000000000000, 0.000000000000000000 ) ) ;
#12987=CARTESIAN_POINT ( 'NONE',  ( -204.2392738945716530, 92.18060771344825355, 28.15437548428747405 ) ) ;
#12991=VERTEX_POINT ( 'NONE', #4688 ) ;
#12994=CARTESIAN_POINT ( 'NONE',  ( -173.5201714974283220, 113.8162285326356198, -26.99751449988017882 ) ) ;
#12997=CARTESIAN_POINT ( 'NONE',  ( -112.1757387330262645, 70.43811608390225842, 82.87215587302765130 ) ) ;
#13000=EDGE_CURVE ( 'NONE', #7514, #19329, #822, .T. ) ;
#13004=VECTOR ( 'NONE', #770, 1000.000000000000000 ) ;
#13007=EDGE_CURVE ( 'NONE', #2948, #15785, #14441, .T. ) ;
#13010=DIRECTION ( 'NONE',  ( -0.000000000000000000, -0.000000000000000000, 1.000000000000000000 ) ) ;
#13014=CARTESIAN_POINT ( 'NONE',  ( -227.3197243376772860, 73.27520359174637576, -17.23934621637404163 ) ) ;
#13015=ADVANCED_FACE ( 'NONE', ( #20359 ), #687, .F. ) ;
#13020=CARTESIAN_POINT ( 'NONE',  ( 112.5876798426281482, 217.9501953190548988, -96.71269508460397901 ) ) ;
#13021=ORIENTED_EDGE ( 'NONE', *, *, #13845, .T. ) ;
#13031=ORIENTED_EDGE ( 'NONE', *, *, #2403, .T. ) ;
#13033=VERTEX_POINT ( 'NONE', #2389 ) ;
#13038=EDGE_LOOP ( 'NONE', ( #11623, #22840, #24480, #27243, #12079, #11263 ) ) ;
#13040=DIRECTION ( 'NONE',  ( 0.000000000000000000, 0.000000000000000000, -1.000000000000000000 ) ) ;
#13043=DIRECTION ( 'NONE',  ( -0.000000000000000000, -0.000000000000000000, 1.000000000000000000 ) ) ;
#13044=DIRECTION ( 'NONE',  ( 0.000000000000000000, 0.000000000000000000, 1.000000000000000000 ) ) ;
#13045=CARTESIAN_POINT ( 'NONE',  ( -279.3160071107327553, -512.7211954420570237, 0.000000000000000000 ) ) ;
#13047=CARTESIAN_POINT ( 'NONE',  ( -219.2341581334216301, 87.88245300808631555, -16.82493878253857034 ) ) ;
#13050=EDGE_CURVE ( 'NONE', #10749, #19092, #17671, .T. ) ;
#13053=CIRCLE ( 'NONE', #12602, 58.59270260175150469 ) ;
#13056=CARTESIAN_POINT ( 'NONE',  ( -279.3160071107327553, -98.68033988749907337, 0.000000000000000000 ) ) ;
#13058=CARTESIAN_POINT ( 'NONE',  ( -160.0000000000000284, 221.6666220619077876, -13.00000000000000000 ) ) ;
#13059=DIRECTION ( 'NONE',  ( 0.000000000000000000, 0.000000000000000000, 1.000000000000000000 ) ) ;
#13060=CARTESIAN_POINT ( 'NONE',  ( 119.9999999999999289, 110.0000000000000142, 100.0000000000000142 ) ) ;
#13065=CARTESIAN_POINT ( 'NONE',  ( 94.60831035304303782, 240.0858928317209688, -18.63379520591212213 ) ) ;
#13070=ORIENTED_EDGE ( 'NONE', *, *, #17239, .T. ) ;
#13072=ORIENTED_EDGE ( 'NONE', *, *, #20910, .F. ) ;
#13073=DIRECTION ( 'NONE',  ( 1.000000000000000000, 0.000000000000000000, 0.000000000000000000 ) ) ;
#13074=CARTESIAN_POINT ( 'NONE',  ( 156.4999999999998579, 220.0000000000000284, -99.00000000000001421 ) ) ;
#13075=DIRECTION ( 'NONE',  ( 0.000000000000000000, 1.000000000000000000, 0.000000000000000000 ) ) ;
#13082=DIRECTION ( 'NONE',  ( -0.000000000000000000, -0.000000000000000000, 1.000000000000000000 ) ) ;
#13084=CARTESIAN_POINT ( 'NONE',  ( -229.0203060419763972, 74.22047013562770701, -16.53676392287966479 ) ) ;
#13085=AXIS2_PLACEMENT_3D ( 'NONE', #10771, #20382, #18517 ) ;
#13086=FACE_OUTER_BOUND ( 'NONE', #15291, .T. ) ;
#13087=CARTESIAN_POINT ( 'NONE',  ( -210.0005531657457425, 60.15481638329399061, 20.01096819387401737 ) ) ;
#13089=CARTESIAN_POINT ( 'NONE',  ( 65.00000000000000000, -120.0250000000000625, 76.00000000000002842 ) ) ;
#13094=CARTESIAN_POINT ( 'NONE',  ( -160.0000000000000568, 119.7660240611718763, 22.85081902853004010 ) ) ;
#13099=EDGE_CURVE ( 'NONE', #12217, #25416, #6178, .T. ) ;
#13100=ORIENTED_EDGE ( 'NONE', *, *, #1442, .F. ) ;
#13109=CARTESIAN_POINT ( 'NONE',  ( 90.17595424778114932, 111.7661400906783626, -100.0000000000108571 ) ) ;
#13112=CARTESIAN_POINT ( 'NONE',  ( -228.1049675858170076, 88.39191058023563130, 15.64816112534147763 ) ) ;
#13113=ORIENTED_EDGE ( 'NONE', *, *, #3152, .F. ) ;
#13119=CARTESIAN_POINT ( 'NONE',  ( 119.9999999999999147, 203.2294901687515676, 100.0000000000000142 ) ) ;
#13122=DIRECTION ( 'NONE',  ( 1.000000000000000000, 0.000000000000000000, 0.000000000000000000 ) ) ;
#13124=AXIS2_PLACEMENT_3D ( 'NONE', #3515, #15016, #23767 ) ;
#13134=ORIENTED_EDGE ( 'NONE', *, *, #25587, .F. ) ;
#13138=CARTESIAN_POINT ( 'NONE',  ( -189.5865564510991703, 103.6848570016005056, -32.44697421272680060 ) ) ;
#13141=CARTESIAN_POINT ( 'NONE',  ( -113.4248494255375164, 71.17701621305222659, 82.82902054666689651 ) ) ;
#13143=ORIENTED_EDGE ( 'NONE', *, *, #24736, .F. ) ;
#13146=CARTESIAN_POINT ( 'NONE',  ( -175.0000000000000000, -120.0000000000001705, 76.00000000000001421 ) ) ;
#13152=CARTESIAN_POINT ( 'NONE',  ( -209.9392232950165749, 62.66904268397140498, -27.74475063248219087 ) ) ;
#13154=ORIENTED_EDGE ( 'NONE', *, *, #8546, .T. ) ;
#13161=DIRECTION ( 'NONE',  ( 0.5555587585212683477, 0.8314772792026894344, -0.000000000000000000 ) ) ;
#13162=CARTESIAN_POINT ( 'NONE',  ( 89.99999999999994316, -90.00000000000001421, -100.0000000000000142 ) ) ;
#13163=DIRECTION ( 'NONE',  ( -0.000000000000000000, -0.000000000000000000, 1.000000000000000000 ) ) ;
#13166=ORIENTED_EDGE ( 'NONE', *, *, #8571, .F. ) ;
#13168=ADVANCED_FACE ( 'NONE', ( #11896 ), #25093, .T. ) ;
#13173=VERTEX_POINT ( 'NONE', #6252 ) ;
#13176=PRODUCT_DEFINITION ( 'UNKNOWN', '', #14340, #24688 ) ;
#13179=CARTESIAN_POINT ( 'NONE',  ( -189.8086322075389774, 92.49158130768422836, -15.00000000000000000 ) ) ;
#13180=CARTESIAN_POINT ( 'NONE',  ( 89.37316688736845549, 230.0797033051429707, 16.48577246127769058 ) ) ;
#13183=VECTOR ( 'NONE', #2443, 1000.000000000000000 ) ;
#13188=LINE ( 'NONE', #8444, #21809 ) ;
#13192=CARTESIAN_POINT ( 'NONE',  ( -124.9781469243919076, 222.2250949724356985, 15.00000000000000000 ) ) ;
#13198=ORIENTED_EDGE ( 'NONE', *, *, #20310, .F. ) ;
#13201=EDGE_CURVE ( 'NONE', #18699, #26642, #18108, .T. ) ;
#13202=ORIENTED_EDGE ( 'NONE', *, *, #23624, .T. ) ;
#13209=CARTESIAN_POINT ( 'NONE',  ( -210.0000000000000284, 59.99999999999993605, -70.00000000000001421 ) ) ;
#13214=CARTESIAN_POINT ( 'NONE',  ( -204.6417490964275885, 60.41478268044740219, 22.13567842568468436 ) ) ;
#13215=CYLINDRICAL_SURFACE ( 'NONE', #8734, 30.00000000000000000 ) ;
#13216=VECTOR ( 'NONE', #20663, 1000.000000000000000 ) ;
#13218=FACE_OUTER_BOUND ( 'NONE', #9341, .T. ) ;
#13221=DIRECTION ( 'NONE',  ( 0.000000000000000000, 0.000000000000000000, -1.000000000000000000 ) ) ;
#13222=CARTESIAN_POINT ( 'NONE',  ( -224.6648725863131233, 72.14980496866132853, -18.55523389629916409 ) ) ;
#13223=ADVANCED_FACE ( 'NONE', ( #19326 ), #4374, .F. ) ;
#13225=FACE_OUTER_BOUND ( 'NONE', #11728, .T. ) ;
#13230=CARTESIAN_POINT ( 'NONE',  ( -228.3238744270677500, 88.44394938709523046, -15.56515158583171576 ) ) ;
#13234=VERTEX_POINT ( 'NONE', #12877 ) ;
#13238=CARTESIAN_POINT ( 'NONE',  ( 79.99999999999991473, 140.0000000000000000, 100.0000000000000142 ) ) ;
#13242=CARTESIAN_POINT ( 'NONE',  ( 96.92716526682083611, 115.1868982021453149, -77.49999999976235188 ) ) ;
#13243=DIRECTION ( 'NONE',  ( 1.000000000000000000, 0.000000000000000000, 0.000000000000000000 ) ) ;
#13245=CARTESIAN_POINT ( 'NONE',  ( -209.0571706919526775, 89.42610521641519483, 24.27378870941836198 ) ) ;
#13253=ORIENTED_EDGE ( 'NONE', *, *, #11410, .F. ) ;
#13254=DIRECTION ( 'NONE',  ( 1.000000000000000000, 0.000000000000000000, 0.000000000000000000 ) ) ;
#13255=AXIS2_PLACEMENT_3D ( 'NONE', #25810, #6942, #2628 ) ;
#13256=EDGE_CURVE ( 'NONE', #2012, #12468, #24071, .T. ) ;
#13257=CARTESIAN_POINT ( 'NONE',  ( -224.0246150495876805, 134.1142769380900575, -12.98324324887284043 ) ) ;
#13262=AXIS2_PLACEMENT_3D ( 'NONE', #22280, #17823, #13243 ) ;
#13265=ORIENTED_EDGE ( 'NONE', *, *, #3753, .T. ) ;
#13266=ORIENTED_EDGE ( 'NONE', *, *, #10319, .F. ) ;
#13267=DIRECTION ( 'NONE',  ( -0.000000000000000000, -0.000000000000000000, -1.000000000000000000 ) ) ;
#13269=CARTESIAN_POINT ( 'NONE',  ( -194.8998556634137174, 99.79200883561803437, -31.71479442048328323 ) ) ;
#13271=VERTEX_POINT ( 'NONE', #10998 ) ;
#13278=DIRECTION ( 'NONE',  ( 0.9960550913260672878, 1.086714821493792890E-17, 0.08873699929240054518 ) ) ;
#13283=ADVANCED_FACE ( 'NONE', ( #17592 ), #14745, .F. ) ;
#13288=EDGE_LOOP ( 'NONE', ( #21633, #449, #19753, #11181 ) ) ;
#13289=AXIS2_PLACEMENT_3D ( 'NONE', #6561, #21792, #17615 ) ;
#13290=CARTESIAN_POINT ( 'NONE',  ( -219.2467648448761395, 139.5102435001769265, 5.000000000000002665 ) ) ;
#13299=CYLINDRICAL_SURFACE ( 'NONE', #15732, 22.49999999999999289 ) ;
#13302=CARTESIAN_POINT ( 'NONE',  ( 22.58950924271104554, 154.2349915562422780, -13.00000000000000000 ) ) ;
#13304=CIRCLE ( 'NONE', #27322, 22.49999999999997868 ) ;
#13307=EDGE_CURVE ( 'NONE', #1799, #7680, #2517, .T. ) ;
#13311=CIRCLE ( 'NONE', #24794, 43.76444293738737912 ) ;
#13312=ADVANCED_FACE ( 'NONE', ( #20466 ), #7109, .T. ) ;
#13315=CARTESIAN_POINT ( 'NONE',  ( -226.9034654753193365, 131.5715075452304745, 15.04814241295084543 ) ) ;
#13316=CARTESIAN_POINT ( 'NONE',  ( 94.58250724493628070, 231.5191281348353982, 18.77838886173626420 ) ) ;
#13317=TOROIDAL_SURFACE ( 'NONE', #4559, 20.00000000000000355, 30.00000000000000000 ) ;
#13319=ADVANCED_FACE ( 'NONE', ( #20031 ), #26350, .F. ) ;
#13324=PLANE ( 'NONE',  #17538 ) ;
#13325=EDGE_CURVE ( 'NONE', #20275, #2290, #24561, .T. ) ;
#13326=CARTESIAN_POINT ( 'NONE',  ( -160.0000000000000284, 109.9999999999999432, 100.0000000000000142 ) ) ;
#13332=DIRECTION ( 'NONE',  ( 0.000000000000000000, 0.000000000000000000, 1.000000000000000000 ) ) ;
#13335=LINE ( 'NONE', #15492, #17643 ) ;
#13342=CARTESIAN_POINT ( 'NONE',  ( 8.117852850209610338, 141.5785587194356197, -13.00000000000000000 ) ) ;
#13346=ORIENTED_EDGE ( 'NONE', *, *, #15432, .T. ) ;
#13354=VECTOR ( 'NONE', #1196, 1000.000000000000000 ) ;
#13355=CARTESIAN_POINT ( 'NONE',  ( -202.1528982378584658, 60.83080389531669852, 24.93098023360008142 ) ) ;
#13359=DIRECTION ( 'NONE',  ( -1.000000000000000000, -2.602085213965211135E-16, 0.000000000000000000 ) ) ;
#13360=CARTESIAN_POINT ( 'NONE',  ( -40.40953891503691153, 0.000000000000000000, 99.00000000000000000 ) ) ;
#13362=CARTESIAN_POINT ( 'NONE',  ( 88.58553289623721128, 111.2425746091579413, 71.46484375014649970 ) ) ;
#13364=CARTESIAN_POINT ( 'NONE',  ( -5.148328491344469349, 133.7892143339873599, 15.61121058808317841 ) ) ;
#13365=CARTESIAN_POINT ( 'NONE',  ( -210.0000000000000284, 59.99999999999994316, 17.29233506344265336 ) ) ;
#13370=CARTESIAN_POINT ( 'NONE',  ( -181.6419045364029614, 108.9881197006330353, 30.31385955260705956 ) ) ;
#13373=ORIENTED_EDGE ( 'NONE', *, *, #1822, .T. ) ;
#13378=CARTESIAN_POINT ( 'NONE',  ( -97.83317650214073069, 134.5241583270075978, 15.50066840981723182 ) ) ;
#13380=CARTESIAN_POINT ( 'NONE',  ( -196.7918453702777128, 71.54464929955099706, 82.80879831960034210 ) ) ;
#13381=EDGE_CURVE ( 'NONE', #8519, #14427, #11727, .T. ) ;
#13385=CARTESIAN_POINT ( 'NONE',  ( -209.0251556266169075, 89.43021808311971199, 25.51491776097941511 ) ) ;
#13394=ADVANCED_FACE ( 'NONE', ( #1346 ), #23634, .T. ) ;
#13395=DIRECTION ( 'NONE',  ( 1.000000000000000000, -0.000000000000000000, -0.000000000000000000 ) ) ;
#13417=DIRECTION ( 'NONE',  ( -0.000000000000000000, 0.000000000000000000, 1.000000000000000000 ) ) ;
#13429=DIRECTION ( 'NONE',  ( 1.000000000000000000, 8.673617379884036705E-17, 0.000000000000000000 ) ) ;
#13438=DIRECTION ( 'NONE',  ( -1.000000000000000000, 0.000000000000000000, 0.000000000000000000 ) ) ;
#13440=VERTEX_POINT ( 'NONE', #18730 ) ;
#13443=CARTESIAN_POINT ( 'NONE',  ( -208.6642397829361926, 74.78008005802638536, 37.85499228847417186 ) ) ;
#13447=ADVANCED_FACE ( 'NONE', ( #16308 ), #4347, .F. ) ;
#13456=VERTEX_POINT ( 'NONE', #18317 ) ;
#13458=CARTESIAN_POINT ( 'NONE',  ( 99.07849735471529584, 234.2556710009807546, 21.83147064533734394 ) ) ;
#13464=CYLINDRICAL_SURFACE ( 'NONE', #18919, 30.00000000000000000 ) ;
#13465=DIRECTION ( 'NONE',  ( 0.000000000000000000, 0.000000000000000000, -1.000000000000000000 ) ) ;
#13474=DIRECTION ( 'NONE',  ( 0.000000000000000000, 0.000000000000000000, -1.000000000000000000 ) ) ;
#13481=VERTEX_POINT ( 'NONE', #16582 ) ;
#13484=EDGE_CURVE ( 'NONE', #18244, #2835, #24168, .T. ) ;
#13487=ORIENTED_EDGE ( 'NONE', *, *, #23656, .F. ) ;
#13488=ORIENTED_EDGE ( 'NONE', *, *, #13540, .F. ) ;
#13491=CIRCLE ( 'NONE', #9369, 1.000000000000000888 ) ;
#13492=DIRECTION ( 'NONE',  ( -1.000000000000000000, 0.000000000000000000, 0.000000000000000000 ) ) ;
#13497=CARTESIAN_POINT ( 'NONE',  ( -216.3288264717405696, 60.34946693787963312, 12.99564918865531382 ) ) ;
#13499=CARTESIAN_POINT ( 'NONE',  ( 33.10302365956999182, 203.2034914284457159, 12.99999999999999822 ) ) ;
#13506=CARTESIAN_POINT ( 'NONE',  ( -209.1829431684195129, 69.04425972296263581, 36.49229859027995815 ) ) ;
#13515=CARTESIAN_POINT ( 'NONE',  ( 125.3433571860710884, 197.9412384757604286, 0.000000000000000000 ) ) ;
#13516=CARTESIAN_POINT ( 'NONE',  ( -207.8525085575914488, 89.95873525663041903, -26.39520176074849545 ) ) ;
#13519=ORIENTED_EDGE ( 'NONE', *, *, #11663, .F. ) ;
#13522=DIRECTION ( 'NONE',  ( -1.000000000000000000, 0.000000000000000000, 0.000000000000000000 ) ) ;
#13523=CARTESIAN_POINT ( 'NONE',  ( -144.6612699377151046, 126.7250878843629778, 18.05549492154933233 ) ) ;
#13527=CARTESIAN_POINT ( 'NONE',  ( 9.999999999999957367, -20.00000000000004974, 110.0000000000000284 ) ) ;
#13529=FACE_OUTER_BOUND ( 'NONE', #11259, .T. ) ;
#13535=AXIS2_PLACEMENT_3D ( 'NONE', #23642, #6395, #10570 ) ;
#13536=CARTESIAN_POINT ( 'NONE',  ( -160.0000000000000568, 139.9999999999999716, 45.00000000000000000 ) ) ;
#13537=CARTESIAN_POINT ( 'NONE',  ( -214.6111699653790197, 58.62522005598040664, -31.77808924747014885 ) ) ;
#13538=ORIENTED_EDGE ( 'NONE', *, *, #6908, .F. ) ;
#13540=EDGE_CURVE ( 'NONE', #18881, #7534, #8950, .T. ) ;
#13542=FACE_OUTER_BOUND ( 'NONE', #8704, .T. ) ;
#13547=CARTESIAN_POINT ( 'NONE',  ( 157.4999999999998579, 220.0000000000000284, -90.00000000000002842 ) ) ;
#13554=CARTESIAN_POINT ( 'NONE',  ( -200.0107575506397097, 95.40263130992853746, -31.09616731377015597 ) ) ;
#13555=EDGE_CURVE ( 'NONE', #15494, #18153, #19434, .T. ) ;
#13557=AXIS2_PLACEMENT_3D ( 'NONE', #17991, #15852, #2180 ) ;
#13566=DIRECTION ( 'NONE',  ( 0.000000000000000000, 0.000000000000000000, -1.000000000000000000 ) ) ;
#13567=AXIS2_PLACEMENT_3D ( 'NONE', #28334, #20012, #4074 ) ;
#13569=CARTESIAN_POINT ( 'NONE',  ( -25.38497998821648594, 129.2235485674940776, -16.97173567987970344 ) ) ;
#13570=DIRECTION ( 'NONE',  ( 1.000000000000000000, -0.000000000000000000, -0.000000000000000000 ) ) ;
#13571=TOROIDAL_SURFACE ( 'NONE', #1617, 23.59849023212046859, 2.000000000000000000 ) ;
#13572=EDGE_CURVE ( 'NONE', #24273, #26495, #22497, .T. ) ;
#13573=CARTESIAN_POINT ( 'NONE',  ( -207.7939942406169109, 74.68924146014083476, -43.59008735158577963 ) ) ;
#13575=EDGE_LOOP ( 'NONE', ( #27490, #5049, #19158, #15573 ) ) ;
#13580=CARTESIAN_POINT ( 'NONE',  ( -214.3828916364065833, 175.2783111443768576, -15.00000000000000000 ) ) ;
#13583=ORIENTED_EDGE ( 'NONE', *, *, #4448, .F. ) ;
#13584=EDGE_CURVE ( 'NONE', #10866, #14018, #25921, .T. ) ;
#13586=CARTESIAN_POINT ( 'NONE',  ( -211.3876077005475906, 59.97725620786449952, -16.20275295307625640 ) ) ;
#13588=ORIENTED_EDGE ( 'NONE', *, *, #21347, .T. ) ;
#13591=CARTESIAN_POINT ( 'NONE',  ( -218.7894661267191054, 71.27542015156993216, 22.74148974320709016 ) ) ;
#13592=ORIENTED_EDGE ( 'NONE', *, *, #23175, .T. ) ;
#13595=CIRCLE ( 'NONE', #15899, 50.00000000000000000 ) ;
#13604=AXIS2_PLACEMENT_3D ( 'NONE', #9478, #18374, #5574 ) ;
#13606=CARTESIAN_POINT ( 'NONE',  ( 104.2862437451156268, 245.6633304404780347, 27.19020029358115309 ) ) ;
#13610=CYLINDRICAL_SURFACE ( 'NONE', #10552, 22.49999999999999289 ) ;
#13615=CARTESIAN_POINT ( 'NONE',  ( 4.996003610813208850E-14, -120.0000000000001137, -25.00000000000000000 ) ) ;
#13616=FACE_OUTER_BOUND ( 'NONE', #17236, .T. ) ;
#13618=CIRCLE ( 'NONE', #15438, 60.59270260175150469 ) ;
#13623=B_SPLINE_CURVE_WITH_KNOTS ( 'NONE', 3,
 ( #7871, #20380, #707, #19069, #3835, #10310, #4116, #21221, #5992, #1544, #19208, #12624, #27953, #3688, #14769, #8152, #1682, #27814 ),
 .UNSPECIFIED., .F., .F.,
 ( 4, 2, 2, 2, 2, 2, 2, 2, 4 ),
 ( 0.000000000000000000, 0.006295559550953947446, 0.009443339326430920735, 0.01101722921416940434, 0.01259111910190788969, 0.01888667865286182412, 0.02046056854060030253, 0.02203445842833878440, 0.02518223820381573427 ),
 .UNSPECIFIED. ) ;
#13625=DIRECTION ( 'NONE',  ( 3.469446951953614189E-16, -1.000000000000000000, 0.000000000000000000 ) ) ;
#13627=DIRECTION ( 'NONE',  ( 0.9960550913260672878, 0.000000000000000000, -0.08873699929240111417 ) ) ;
#13634=ORIENTED_EDGE ( 'NONE', *, *, #1618, .T. ) ;
#13635=EDGE_CURVE ( 'NONE', #13747, #22333, #26748, .T. ) ;
#13640=CARTESIAN_POINT ( 'NONE',  ( -141.6428522700808230, 17.24192588826928585, 83.00000000000001421 ) ) ;
#13642=FACE_OUTER_BOUND ( 'NONE', #2573, .T. ) ;
#13644=CARTESIAN_POINT ( 'NONE',  ( -206.8153965817337223, 60.16463287088505751, 19.99797379519356610 ) ) ;
#13646=DIRECTION ( 'NONE',  ( 0.000000000000000000, 0.000000000000000000, -1.000000000000000000 ) ) ;
#13647=FACE_OUTER_BOUND ( 'NONE', #7260, .T. ) ;
#13648=CARTESIAN_POINT ( 'NONE',  ( -205.8153486680121489, 91.09410686308810057, -26.99305210841084701 ) ) ;
#13654=DIRECTION ( 'NONE',  ( -0.000000000000000000, -1.000000000000000000, -0.000000000000000000 ) ) ;
#13658=ORIENTED_EDGE ( 'NONE', *, *, #8445, .F. ) ;
#13659=EDGE_LOOP ( 'NONE', ( #15003, #15101, #28300, #12915 ) ) ;
#13660=CARTESIAN_POINT ( 'NONE',  ( -222.0755484219518507, 86.46466326799983904, -17.72675295328876643 ) ) ;
#13661=VECTOR ( 'NONE', #122, 1000.000000000000000 ) ;
#13667=DIRECTION ( 'NONE',  ( -3.469446951953614189E-16, 1.000000000000000000, 0.000000000000000000 ) ) ;
#13672=DIRECTION ( 'NONE',  ( 0.000000000000000000, 0.000000000000000000, -1.000000000000000000 ) ) ;
#13675=FACE_OUTER_BOUND ( 'NONE', #22835, .T. ) ;
#13678=AXIS2_PLACEMENT_3D ( 'NONE', #15368, #11044, #23550 ) ;
#13682=EDGE_CURVE ( 'NONE', #20039, #20004, #26597, .T. ) ;
#13684=CARTESIAN_POINT ( 'NONE',  ( -208.1368626653883780, 75.14204529818155720, -39.73078884062161364 ) ) ;
#13685=EDGE_CURVE ( 'NONE', #2005, #12217, #5048, .T. ) ;
#13688=EDGE_CURVE ( 'NONE', #2661, #8764, #182, .T. ) ;
#13689=CARTESIAN_POINT ( 'NONE',  ( -216.6285193170544972, 139.2238166778980712, -12.99999999956374452 ) ) ;
#13690=DIRECTION ( 'NONE',  ( 1.000000000000000000, 0.000000000000000000, -0.000000000000000000 ) ) ;
#13694=CONICAL_SURFACE ( 'NONE', #24219, 16.36034929305424512, 0.08885387018394150238 ) ;
#13696=AXIS2_PLACEMENT_3D ( 'NONE', #12832, #25885, #1889 ) ;
#13697=CARTESIAN_POINT ( 'NONE',  ( -142.1532754773451757, 70.11332714433679314, 82.89218380363524830 ) ) ;
#13699=ORIENTED_EDGE ( 'NONE', *, *, #1822, .F. ) ;
#13700=CARTESIAN_POINT ( 'NONE',  ( 87.74278500247204704, 111.0010834413667453, 71.13281249985656984 ) ) ;
#13702=ORIENTED_EDGE ( 'NONE', *, *, #5201, .T. ) ;
#13704=FACE_OUTER_BOUND ( 'NONE', #22351, .T. ) ;
#13706=AXIS2_PLACEMENT_3D ( 'NONE', #7002, #14192, #20784 ) ;
#13710=FACE_BOUND ( 'NONE', #25640, .T. ) ;
#13711=AXIS2_PLACEMENT_3D ( 'NONE', #533, #9296, #18061 ) ;
#13712=EDGE_CURVE ( 'NONE', #15645, #4667, #9661, .T. ) ;
#13714=LINE ( 'NONE', #22884, #1166 ) ;
#13715=CARTESIAN_POINT ( 'NONE',  ( -270.1025481742786951, -91.18033988749901653, 0.000000000000000000 ) ) ;
#13716=CARTESIAN_POINT ( 'NONE',  ( -23.68577686495459389, 129.3251568248628587, -16.93270094945798832 ) ) ;
#13718=DIRECTION ( 'NONE',  ( -0.000000000000000000, 1.000000000000000000, -1.387778780781445429E-16 ) ) ;
#13719=LINE ( 'NONE', #9543, #17094 ) ;
#13720=EDGE_LOOP ( 'NONE', ( #7072, #21816, #20041, #15929 ) ) ;
#13732=CARTESIAN_POINT ( 'NONE',  ( -210.0000000000000284, 59.99999999999993605, -17.29233506344264626 ) ) ;
#13737=AXIS2_PLACEMENT_3D ( 'NONE', #19106, #10070, #7907 ) ;
#13738=DIRECTION ( 'NONE',  ( 0.000000000000000000, 0.000000000000000000, 1.000000000000000000 ) ) ;
#13740=CARTESIAN_POINT ( 'NONE',  ( 93.75313621282120380, 240.3341199031587507, 8.151442483331582167 ) ) ;
#13743=ORIENTED_EDGE ( 'NONE', *, *, #23750, .F. ) ;
#13745=ORIENTED_EDGE ( 'NONE', *, *, #3111, .T. ) ;
#13747=VERTEX_POINT ( 'NONE', #3452 ) ;
#13748=CARTESIAN_POINT ( 'NONE',  ( 107.1040180392210743, 249.6169203092825626, 26.84244457533995742 ) ) ;
#13751=CARTESIAN_POINT ( 'NONE',  ( -222.0211651016020085, 135.7213904098416322, 12.97555235349485514 ) ) ;
#13755=CIRCLE ( 'NONE', #4533, 6.000000000000005329 ) ;
#13757=DIRECTION ( 'NONE',  ( 0.000000000000000000, 0.000000000000000000, -1.000000000000000000 ) ) ;
#13760=DIRECTION ( 'NONE',  ( 1.000000000000000000, 0.000000000000000000, 0.000000000000000000 ) ) ;
#13766=EDGE_CURVE ( 'NONE', #12684, #14756, #3170, .T. ) ;
#13770=DIRECTION ( 'NONE',  ( 0.000000000000000000, 0.000000000000000000, 1.000000000000000000 ) ) ;
#13774=ORIENTED_EDGE ( 'NONE', *, *, #14015, .T. ) ;
#13781=ORIENTED_EDGE ( 'NONE', *, *, #20410, .F. ) ;
#13783=CARTESIAN_POINT ( 'NONE',  ( -189.8086322075389774, 92.49158130768422836, -15.00000000000000000 ) ) ;
#13785=DIRECTION ( 'NONE',  ( 0.000000000000000000, 0.000000000000000000, 1.000000000000000000 ) ) ;
#13787=CARTESIAN_POINT ( 'NONE',  ( -100.2451658495067477, 134.3005718521120286, -15.54624248649205853 ) ) ;
#13791=CARTESIAN_POINT ( 'NONE',  ( -214.2384622483376688, 55.08766841006207926, 45.11431866370089239 ) ) ;
#13795=DIRECTION ( 'NONE',  ( 0.000000000000000000, 0.000000000000000000, -1.000000000000000000 ) ) ;
#13796=CARTESIAN_POINT ( 'NONE',  ( -228.6461399146356257, 91.02766744526201137, -13.29913430599589219 ) ) ;
#13800=CIRCLE ( 'NONE', #26601, 32.49120955644046660 ) ;
#13801=CARTESIAN_POINT ( 'NONE',  ( -6.675997603934725078, 131.5976059255800408, 16.20004726215371704 ) ) ;
#13805=ORIENTED_EDGE ( 'NONE', *, *, #4995, .T. ) ;
#13809=VERTEX_POINT ( 'NONE', #9520 ) ;
#13810=ORIENTED_EDGE ( 'NONE', *, *, #18339, .F. ) ;
#13814=CARTESIAN_POINT ( 'NONE',  ( -148.8594576708775037, 124.1404238845194357, 19.51865504791162564 ) ) ;
#13817=CARTESIAN_POINT ( 'NONE',  ( -167.5793538779647918, 116.3743944715606204, -25.89383771362038544 ) ) ;
#13819=ADVANCED_FACE ( 'NONE', ( #1306 ), #11687, .T. ) ;
#13824=CARTESIAN_POINT ( 'NONE',  ( -204.4116019472746473, 91.57545976731941550, 29.21054719826555868 ) ) ;
#13825=CARTESIAN_POINT ( 'NONE',  ( 87.50000000000029843, 230.0000000000000284, -15.95262490344447492 ) ) ;
#13827=DIRECTION ( 'NONE',  ( -0.000000000000000000, -1.000000000000000000, -0.000000000000000000 ) ) ;
#13828=CARTESIAN_POINT ( 'NONE',  ( -213.1074610084601773, 72.43174512725769887, -29.09741138161720642 ) ) ;
#13829=CIRCLE ( 'NONE', #6013, 7.499999999999992895 ) ;
#13838=CARTESIAN_POINT ( 'NONE',  ( -244.5479615644635487, 75.99513337129094737, 15.00000000000000000 ) ) ;
#13844=EDGE_LOOP ( 'NONE', ( #4916, #10227, #832, #21593, #6043, #16381, #11657, #24528 ) ) ;
#13845=EDGE_CURVE ( 'NONE', #12991, #26678, #20981, .T. ) ;
#13848=FACE_OUTER_BOUND ( 'NONE', #4123, .T. ) ;
#13849=EDGE_CURVE ( 'NONE', #12468, #4808, #22283, .T. ) ;
#13853=CARTESIAN_POINT ( 'NONE',  ( 134.9999999999998579, 220.0000000000000284, -99.00000000000001421 ) ) ;
#13855=DIRECTION ( 'NONE',  ( 0.000000000000000000, 0.000000000000000000, -1.000000000000000000 ) ) ;
#13856=ORIENTED_EDGE ( 'NONE', *, *, #5887, .T. ) ;
#13858=DIRECTION ( 'NONE',  ( 0.000000000000000000, 0.000000000000000000, -1.000000000000000000 ) ) ;
#13862=CARTESIAN_POINT ( 'NONE',  ( -1.123482218186120596, 135.6325438607385649, -15.26633278495360635 ) ) ;
#13868=CARTESIAN_POINT ( 'NONE',  ( -229.2498027451139251, 132.0565166830976693, 15.00000000000000000 ) ) ;
#13869=FACE_OUTER_BOUND ( 'NONE', #3989, .T. ) ;
#13872=CARTESIAN_POINT ( 'NONE',  ( -235.5935699371920293, 67.74125567661748448, 5.863186529791164503 ) ) ;
#13873=ORIENTED_EDGE ( 'NONE', *, *, #1145, .T. ) ;
#13875=CARTESIAN_POINT ( 'NONE',  ( 112.4999999999998863, 220.0000000000000284, 84.99999999999995737 ) ) ;
#13879=DIRECTION ( 'NONE',  ( -0.000000000000000000, 0.000000000000000000, 1.000000000000000000 ) ) ;
#13882=EDGE_CURVE ( 'NONE', #18977, #12684, #2069, .T. ) ;
#13884=EDGE_CURVE ( 'NONE', #15785, #4808, #19981, .T. ) ;
#13888=EDGE_LOOP ( 'NONE', ( #10607, #27444 ) ) ;
#13891=ORIENTED_EDGE ( 'NONE', *, *, #1721, .F. ) ;
#13895=TOROIDAL_SURFACE ( 'NONE', #15323, 79.71075545852265520, 9.999999999999996447 ) ;
#13896=CARTESIAN_POINT ( 'NONE',  ( 109.2338094452269246, 254.3984564255594591, 35.27666983503019082 ) ) ;
#13897=EDGE_CURVE ( 'NONE', #2501, #19721, #16331, .T. ) ;
#13898=AXIS2_PLACEMENT_3D ( 'NONE', #16264, #16403, #9373 ) ;
#13899=CARTESIAN_POINT ( 'NONE',  ( -28.05246235954390244, 188.0718642840173516, 12.99999999999999822 ) ) ;
#13901=VECTOR ( 'NONE', #17815, 1000.000000000000000 ) ;
#13907=DIRECTION ( 'NONE',  ( 1.000000000000000000, 0.000000000000000000, -0.000000000000000000 ) ) ;
#13911=VERTEX_POINT ( 'NONE', #23285 ) ;
#13912=DIRECTION ( 'NONE',  ( 1.000000000000000000, 0.000000000000000000, 0.000000000000000000 ) ) ;
#13915=ORIENTED_EDGE ( 'NONE', *, *, #912, .F. ) ;
#13917=EDGE_CURVE ( 'NONE', #15896, #19755, #8484, .T. ) ;
#13918=AXIS2_PLACEMENT_3D ( 'NONE', #26558, #23852, #6887 ) ;
#13920=ORIENTED_EDGE ( 'NONE', *, *, #6850, .T. ) ;
#13922=AXIS2_PLACEMENT_3D ( 'NONE', #6735, #10773, #25847 ) ;
#13928=CARTESIAN_POINT ( 'NONE',  ( -135.2376737518963807, 129.6700313254847856, 15.43675878823252035 ) ) ;
#13931=B_SPLINE_CURVE_WITH_KNOTS ( 'NONE', 3,
 ( #18715, #7941, #27745, #27463, #12130, #5922, #23594, #14694, #8082, #16847, #3762, #12551, #6062, #23030, #1192, #20873, #7803, #25323, #5645, #14095, #731, #24861, #13817, #20543, #14372, #18670 ),
 .UNSPECIFIED., .F., .F.,
 ( 4, 2, 2, 2, 2, 2, 2, 2, 2, 2, 2, 2, 4 ),
 ( 0.000000000000000000, 0.003366647192498294170, 0.006733294384996588340, 0.01346658876999323913, 0.01683323596249157797, 0.02019988315498991160, 0.02188320675123906975, 0.02356653034748822442, 0.02693317753998661010, 0.03366647192498332941, 0.04039976630998005913, 0.04713306069497678885, 0.05386635507997350469 ),
 .UNSPECIFIED. ) ;
#13937=CARTESIAN_POINT ( 'NONE',  ( -194.2411556039511709, 63.21395545898181467, 45.39084185613187827 ) ) ;
#13944=DIRECTION ( 'NONE',  ( -0.000000000000000000, -0.000000000000000000, -1.000000000000000000 ) ) ;
#13946=DIRECTION ( 'NONE',  ( 1.000000000000000000, 0.000000000000000000, 0.000000000000000000 ) ) ;
#13949=CARTESIAN_POINT ( 'NONE',  ( -210.0000000000000284, 59.99999999999993605, -17.29233506344264626 ) ) ;
#13950=FACE_OUTER_BOUND ( 'NONE', #19548, .T. ) ;
#13957=VECTOR ( 'NONE', #2737, 1000.000000000000000 ) ;
#13958=ORIENTED_EDGE ( 'NONE', *, *, #5735, .F. ) ;
#13959=AXIS2_PLACEMENT_3D ( 'NONE', #7218, #18136, #15992 ) ;
#13962=ORIENTED_EDGE ( 'NONE', *, *, #11215, .F. ) ;
#13966=DIRECTION ( 'NONE',  ( 1.530283246943720875E-16, -1.000000000000000000, 0.000000000000000000 ) ) ;
#13967=EDGE_CURVE ( 'NONE', #16893, #1362, #3919, .T. ) ;
#13968=ADVANCED_FACE ( 'NONE', ( #1586 ), #10354, .F. ) ;
#13973=CARTESIAN_POINT ( 'NONE',  ( -215.0107612850210899, 71.82996193033663701, -26.64107447012230878 ) ) ;
#13977=DIRECTION ( 'NONE',  ( 0.000000000000000000, 0.000000000000000000, -1.000000000000000000 ) ) ;
#13985=CARTESIAN_POINT ( 'NONE',  ( -244.5479615644635487, 75.99513337129094737, 5.000000000000002665 ) ) ;
#13986=CARTESIAN_POINT ( 'NONE',  ( -160.0000000000000284, 59.99999999999994316, 15.00000000000000000 ) ) ;
#13987=ORIENTED_EDGE ( 'NONE', *, *, #10519, .T. ) ;
#13990=CARTESIAN_POINT ( 'NONE',  ( 96.92716526683047107, 115.1868982021512124, 77.49999999971905140 ) ) ;
#13996=CARTESIAN_POINT ( 'NONE',  ( -205.1370039499190625, 144.1304017549904586, -15.00000000000000000 ) ) ;
#14000=AXIS2_PLACEMENT_3D ( 'NONE', #25788, #27930, #28073 ) ;
#14003=DIRECTION ( 'NONE',  ( -1.000000000000000000, -0.000000000000000000, 0.000000000000000000 ) ) ;
#14004=CARTESIAN_POINT ( 'NONE',  ( -27.07984315909205009, 129.1630299464794405, -16.99514979029525108 ) ) ;
#14008=ORIENTED_EDGE ( 'NONE', *, *, #27343, .F. ) ;
#14010=VECTOR ( 'NONE', #23481, 1000.000000000000000 ) ;
#14011=LINE ( 'NONE', #9826, #8799 ) ;
#14012=FACE_BOUND ( 'NONE', #18758, .T. ) ;
#14014=VECTOR ( 'NONE', #15660, 1000.000000000000000 ) ;
#14015=EDGE_CURVE ( 'NONE', #27002, #25971, #3001, .T. ) ;
#14018=VERTEX_POINT ( 'NONE', #7 ) ;
#14020=CARTESIAN_POINT ( 'NONE',  ( 89.99999999999988631, 240.0000000000000284, -45.00000000000000000 ) ) ;
#14022=DIRECTION ( 'NONE',  ( 0.000000000000000000, 0.000000000000000000, 1.000000000000000000 ) ) ;
#14024=CARTESIAN_POINT ( 'NONE',  ( -21.33210486176665910, 0.000000000000000000, 100.0000000000000000 ) ) ;
#14025=LINE ( 'NONE', #5375, #10682 ) ;
#14029=CARTESIAN_POINT ( 'NONE',  ( 97.40125796617704168, 241.4156732773147667, 11.01277537798790007 ) ) ;
#14039=DIRECTION ( 'NONE',  ( 1.000000000000000000, 0.000000000000000000, 0.000000000000000000 ) ) ;
#14040=DIRECTION ( 'NONE',  ( -0.000000000000000000, -0.000000000000000000, 1.000000000000000000 ) ) ;
#14042=DIRECTION ( 'NONE',  ( 1.000000000000000000, 0.000000000000000000, 0.000000000000000000 ) ) ;
#14046=DIRECTION ( 'NONE',  ( 1.000000000000000000, 1.530283246943720628E-16, 0.000000000000000000 ) ) ;
#14049=CARTESIAN_POINT ( 'NONE',  ( 115.1343022193454004, 209.3890158820094314, -98.75454612047968794 ) ) ;
#14051=EDGE_CURVE ( 'NONE', #7786, #7612, #8044, .T. ) ;
#14052=ADVANCED_FACE ( 'NONE', ( #26420 ), #1289, .T. ) ;
#14055=CIRCLE ( 'NONE', #1635, 1.999999999999993339 ) ;
#14056=CARTESIAN_POINT ( 'NONE',  ( -146.6428522700808230, 74.54464929955099706, 80.00000000000001421 ) ) ;
#14063=VERTEX_POINT ( 'NONE', #6421 ) ;
#14064=ORIENTED_EDGE ( 'NONE', *, *, #6850, .F. ) ;
#14066=CARTESIAN_POINT ( 'NONE',  ( -67.47855672616037737, 135.5178657931547832, 13.65870838648359964 ) ) ;
#14068=DIRECTION ( 'NONE',  ( 1.000000000000000000, 1.850371707708594316E-16, -0.000000000000000000 ) ) ;
#14069=CARTESIAN_POINT ( 'NONE',  ( -90.16297593177748126, 134.7821557438530533, -15.45724512967298026 ) ) ;
#14070=CIRCLE ( 'NONE', #25071, 4.355764593064429313 ) ;
#14071=CARTESIAN_POINT ( 'NONE',  ( 134.9999999999998579, 171.5103103742661688, 84.99999999999995737 ) ) ;
#14072=CARTESIAN_POINT ( 'NONE',  ( -194.7277720219268815, 63.01928361507884091, 39.96465835449415493 ) ) ;
#14073=FACE_OUTER_BOUND ( 'NONE', #14930, .T. ) ;
#14076=CARTESIAN_POINT ( 'NONE',  ( 79.99999999999997158, 81.96349540849362825, -100.0000000000000284 ) ) ;
#14077=CARTESIAN_POINT ( 'NONE',  ( -221.0514588393455142, 88.12431193532715668, -15.86718054107228859 ) ) ;
#14079=CARTESIAN_POINT ( 'NONE',  ( -254.3350114625770289, -91.18033988749901653, 0.000000000000000000 ) ) ;
#14080=DIRECTION ( 'NONE',  ( 0.000000000000000000, 0.000000000000000000, 1.000000000000000000 ) ) ;
#14082=CARTESIAN_POINT ( 'NONE',  ( -76.25760768171835480, 219.6666220619077876, -15.00000000000000000 ) ) ;
#14083=CARTESIAN_POINT ( 'NONE',  ( 111.0641325991587252, 99.15168937823352735, -100.0000000000000142 ) ) ;
#14084=DIRECTION ( 'NONE',  ( 1.000000000000000000, 0.000000000000000000, 0.000000000000000000 ) ) ;
#14087=EDGE_CURVE ( 'NONE', #26198, #19256, #23657, .T. ) ;
#14092=DIRECTION ( 'NONE',  ( -1.000000000000000000, 0.000000000000000000, 0.000000000000000000 ) ) ;
#14095=CARTESIAN_POINT ( 'NONE',  ( -174.9473576776401842, 112.5984928542032151, -28.94822812299444337 ) ) ;
#14104=CARTESIAN_POINT ( 'NONE',  ( -202.1528982378773946, 60.83080389531252763, -24.93098023360007431 ) ) ;
#14107=DIRECTION ( 'NONE',  ( -1.000000000000000000, -8.673617379884036705E-17, 0.000000000000000000 ) ) ;
#14108=CARTESIAN_POINT ( 'NONE',  ( -138.6428522700808230, 71.54464929955099706, 83.00000000000001421 ) ) ;
#14114=CARTESIAN_POINT ( 'NONE',  ( -231.1655399901254384, 65.02775169233193253, 6.844214734954432444 ) ) ;
#14115=CARTESIAN_POINT ( 'NONE',  ( -156.8436863811591593, 180.7779002010535692, 12.99999999999999822 ) ) ;
#14118=VERTEX_POINT ( 'NONE', #28056 ) ;
#14119=CARTESIAN_POINT ( 'NONE',  ( 109.9999999999999147, 140.0000000000000000, 90.00000000000002842 ) ) ;
#14126=CIRCLE ( 'NONE', #1714, 55.86582179324592090 ) ;
#14127=CARTESIAN_POINT ( 'NONE',  ( -76.25760768171836901, 154.8982798170083299, -15.00000000000000000 ) ) ;
#14128=CARTESIAN_POINT ( 'NONE',  ( -273.6211430000234373, -91.18033988749901653, 0.000000000000000000 ) ) ;
#14131=ORIENTED_EDGE ( 'NONE', *, *, #2663, .F. ) ;
#14133=EDGE_CURVE ( 'NONE', #606, #5551, #4219, .T. ) ;
#14137=CARTESIAN_POINT ( 'NONE',  ( 4.490032364213274008, 138.9202551321229464, -13.09535261425119224 ) ) ;
#14147=CARTESIAN_POINT ( 'NONE',  ( -124.9781469243919076, 222.2250949724356985, 5.000000000000002665 ) ) ;
#14149=CARTESIAN_POINT ( 'NONE',  ( -242.2383635333241898, 73.34843395317835757, 5.047097023363151358 ) ) ;
#14156=DIRECTION ( 'NONE',  ( -0.5555587585212683477, -0.8314772792026894344, 0.000000000000000000 ) ) ;
#14157=ORIENTED_EDGE ( 'NONE', *, *, #27411, .T. ) ;
#14158=CARTESIAN_POINT ( 'NONE',  ( -81.41884555190407013, 134.7389654164047386, 15.46487976177122015 ) ) ;
#14159=CARTESIAN_POINT ( 'NONE',  ( 95.84672108982582017, 240.8689139502125158, 9.670646206302331294 ) ) ;
#14161=EDGE_LOOP ( 'NONE', ( #19888, #21151, #6787, #24540 ) ) ;
#14166=ORIENTED_EDGE ( 'NONE', *, *, #27771, .T. ) ;
#14169=CARTESIAN_POINT ( 'NONE',  ( 108.2753065237184984, 248.3531133182649739, 34.86527342666781237 ) ) ;
#14172=CARTESIAN_POINT ( 'NONE',  ( -218.8273392347298341, 140.3457761587514767, -14.99191580167117266 ) ) ;
#14173=CARTESIAN_POINT ( 'NONE',  ( 88.58553289623264959, 111.2425746091564491, -71.46484375013500312 ) ) ;
#14175=DIRECTION ( 'NONE',  ( 0.5555587585212703461, 0.8314772792026879911, -9.637408206913768347E-16 ) ) ;
#14177=LINE ( 'NONE', #20203, #1669 ) ;
#14180=DIRECTION ( 'NONE',  ( 1.000000000000000000, -0.000000000000000000, -0.000000000000000000 ) ) ;
#14182=AXIS2_PLACEMENT_3D ( 'NONE', #25778, #27922, #28065 ) ;
#14184=CARTESIAN_POINT ( 'NONE',  ( 93.75311240682748348, 240.3341156238397218, -8.151427701230094414 ) ) ;
#14185=CARTESIAN_POINT ( 'NONE',  ( 18.34304381486422741, 88.89403053572398505, 98.65506662663811710 ) ) ;
#14188=AXIS2_PLACEMENT_3D ( 'NONE', #6621, #4598, #9360 ) ;
#14190=EDGE_LOOP ( 'NONE', ( #25129, #14883, #11227, #6296 ) ) ;
#14192=DIRECTION ( 'NONE',  ( -0.6343833064826058799, 0.7730186417261851739, 0.000000000000000000 ) ) ;
#14194=VECTOR ( 'NONE', #19008, 1000.000000000000000 ) ;
#14198=EDGE_CURVE ( 'NONE', #7226, #11653, #15880, .T. ) ;
#14200=FACE_OUTER_BOUND ( 'NONE', #4134, .T. ) ;
#14206=ADVANCED_FACE ( 'NONE', ( #24475 ), #6065, .T. ) ;
#14207=CARTESIAN_POINT ( 'NONE',  ( -62.70704562728440834, 133.3662835691973214, -15.73207420746911289 ) ) ;
#14210=CARTESIAN_POINT ( 'NONE',  ( -214.1250002713545086, 55.22895589251825754, 44.08339233875913976 ) ) ;
#14212=CARTESIAN_POINT ( 'NONE',  ( -142.3347590520894812, 127.5090500945063070, -16.40665191978878568 ) ) ;
#14214=CARTESIAN_POINT ( 'NONE',  ( -203.7172301001751578, 92.58626701197334796, -28.49277624592259528 ) ) ;
#14220=AXIS2_PLACEMENT_3D ( 'NONE', #26830, #24531, #27244 ) ;
#14227=VERTEX_POINT ( 'NONE', #17366 ) ;
#14228=ORIENTED_EDGE ( 'NONE', *, *, #15411, .F. ) ;
#14237=VECTOR ( 'NONE', #14040, 1000.000000000000000 ) ;
#14239=CARTESIAN_POINT ( 'NONE',  ( 109.9999999999999574, -120.0000000000000426, 100.0000000000000142 ) ) ;
#14240=CARTESIAN_POINT ( 'NONE',  ( 97.56713245600785456, 233.1474958787437970, -20.66394368293470407 ) ) ;
#14242=CARTESIAN_POINT ( 'NONE',  ( -210.7172313291012529, 103.7585653882801182, -15.00000000000000000 ) ) ;
#14246=CARTESIAN_POINT ( 'NONE',  ( -217.2638015013723418, 71.38783981852336069, -24.17165906551136700 ) ) ;
#14248=DIRECTION ( 'NONE',  ( 4.163336342344337027E-16, -1.000000000000000000, 1.387778780781445429E-16 ) ) ;
#14252=CARTESIAN_POINT ( 'NONE',  ( 118.3245732435423037, 235.1487993679093051, -99.88685888571279747 ) ) ;
#14260=CARTESIAN_POINT ( 'NONE',  ( 104.1118574119297762, 122.0584436052485700, 84.84374999969743669 ) ) ;
#14264=CARTESIAN_POINT ( 'NONE',  ( -160.8326600028555902, 120.2355194873575073, 21.37420696376536711 ) ) ;
#14268=CARTESIAN_POINT ( 'NONE',  ( 119.9999999987673220, 136.1131920015923811, 100.0000000000000142 ) ) ;
#14277=DIRECTION ( 'NONE',  ( -0.000000000000000000, 1.000000000000000000, -1.387778780781445429E-16 ) ) ;
#14285=CARTESIAN_POINT ( 'NONE',  ( -180.0000000000000284, -40.00000000000004974, 25.00000000000000711 ) ) ;
#14286=ORIENTED_EDGE ( 'NONE', *, *, #6270, .F. ) ;
#14288=CARTESIAN_POINT ( 'NONE',  ( -234.1469129038714811, 66.78385994367808109, 6.149209796590400678 ) ) ;
#14289=ORIENTED_EDGE ( 'NONE', *, *, #21100, .T. ) ;
#14295=VERTEX_POINT ( 'NONE', #16565 ) ;
#14296=AXIS2_PLACEMENT_3D ( 'NONE', #9582, #18755, #11889 ) ;
#14297=CARTESIAN_POINT ( 'NONE',  ( -134.5347440196730133, 128.5535302534177617, 17.26723801115314316 ) ) ;
#14298=CARTESIAN_POINT ( 'NONE',  ( 109.8317202412775657, 257.3567735479731482, 40.41962601158171964 ) ) ;
#14300=VERTEX_POINT ( 'NONE', #5641 ) ;
#14303=CIRCLE ( 'NONE', #27574, 23.59849023212046149 ) ;
#14310=CARTESIAN_POINT ( 'NONE',  ( 105.2480867101029531, 123.6573351780301095, -85.93750000029402258 ) ) ;
#14317=CARTESIAN_POINT ( 'NONE',  ( 33.10302365956999182, 221.6666220619077876, -13.00000000000000000 ) ) ;
#14319=ORIENTED_EDGE ( 'NONE', *, *, #12611, .T. ) ;
#14320=CARTESIAN_POINT ( 'NONE',  ( -6.136237936124284253, 131.7900252471816884, 16.14451440323835740 ) ) ;
#14321=CARTESIAN_POINT ( 'NONE',  ( 109.9999999999998863, 258.9419543489020725, -43.16741111682571130 ) ) ;
#14323=DIRECTION ( 'NONE',  ( -0.000000000000000000, -1.000000000000000000, -0.000000000000000000 ) ) ;
#14327=EDGE_CURVE ( 'NONE', #13271, #2501, #6692, .T. ) ;
#14333=ORIENTED_EDGE ( 'NONE', *, *, #313, .F. ) ;
#14335=ORIENTED_EDGE ( 'NONE', *, *, #11073, .F. ) ;
#14337=ORIENTED_EDGE ( 'NONE', *, *, #8884, .T. ) ;
#14338=CIRCLE ( 'NONE', #2862, 30.00000000000000000 ) ;
#14340=PRODUCT_DEFINITION_FORMATION_WITH_SPECIFIED_SOURCE ( 'ANY', '', #14871, .NOT_KNOWN. ) ;
#14341=DIRECTION ( 'NONE',  ( 0.000000000000000000, 1.000000000000000000, -0.000000000000000000 ) ) ;
#14342=PLANE ( 'NONE',  #28082 ) ;
#14344=CARTESIAN_POINT ( 'NONE',  ( -96.55704474936557347, 136.1739396949002980, -15.19855580619790025 ) ) ;
#14348=FACE_OUTER_BOUND ( 'NONE', #20789, .T. ) ;
#14355=AXIS2_PLACEMENT_3D ( 'NONE', #3275, #17173, #23640 ) ;
#14360=CIRCLE ( 'NONE', #5651, 18.46313063346208239 ) ;
#14362=ORIENTED_EDGE ( 'NONE', *, *, #25574, .T. ) ;
#14363=VECTOR ( 'NONE', #21589, 1000.000000000000000 ) ;
#14367=ORIENTED_EDGE ( 'NONE', *, *, #23498, .T. ) ;
#14371=EDGE_LOOP ( 'NONE', ( #10763, #21884, #6108, #4775 ) ) ;
#14372=CARTESIAN_POINT ( 'NONE',  ( -161.9247682478280979, 118.9584040179142761, -23.58860542993421916 ) ) ;
#14377=CIRCLE ( 'NONE', #27660, 1.999999999999996891 ) ;
#14378=AXIS2_PLACEMENT_3D ( 'NONE', #12038, #12181, #7581 ) ;
#14382=CARTESIAN_POINT ( 'NONE',  ( 134.9999999999998579, 220.0000000000000284, 100.0000000000000142 ) ) ;
#14383=ADVANCED_FACE ( 'NONE', ( #13647 ), #11198, .F. ) ;
#14387=ORIENTED_EDGE ( 'NONE', *, *, #16341, .F. ) ;
#14388=AXIS2_PLACEMENT_3D ( 'NONE', #14652, #6167, #23131 ) ;
#14389=CARTESIAN_POINT ( 'NONE',  ( -203.1779787704217313, 93.05164332230201296, 28.77272332722130699 ) ) ;
#14394=ORIENTED_EDGE ( 'NONE', *, *, #1295, .T. ) ;
#14403=CARTESIAN_POINT ( 'NONE',  ( 88.58553289623264959, 111.2425746091564491, -71.46484375013500312 ) ) ;
#14404=CARTESIAN_POINT ( 'NONE',  ( 95.56986273107233387, 231.9897703952537995, 19.35213621132750106 ) ) ;
#14406=VERTEX_POINT ( 'NONE', #8755 ) ;
#14409=CONICAL_SURFACE ( 'NONE', #22213, 21.20097097723064294, 0.08885387018394180769 ) ;
#14412=DIRECTION ( 'NONE',  ( 0.8790438869537404720, 0.4767408570798813972, -0.000000000000000000 ) ) ;
#14413=EDGE_CURVE ( 'NONE', #18325, #22419, #19670, .T. ) ;
#14416=DIRECTION ( 'NONE',  ( 1.000000000000000000, 0.000000000000000000, 0.000000000000000000 ) ) ;
#14421=CARTESIAN_POINT ( 'NONE',  ( 134.9999999999998579, -150.0000000000000284, -84.99999999999997158 ) ) ;
#14426=CARTESIAN_POINT ( 'NONE',  ( -175.0000000000000000, -120.0000000000001705, 76.02500000000001990 ) ) ;
#14427=VERTEX_POINT ( 'NONE', #24405 ) ;
#14428=ADVANCED_FACE ( 'NONE', ( #22108 ), #17793, .T. ) ;
#14429=CARTESIAN_POINT ( 'NONE',  ( -112.3221550338875687, 22.24192588826928585, 83.00000000000001421 ) ) ;
#14430=CARTESIAN_POINT ( 'NONE',  ( 20.92655468430566756, 155.3461090732848220, -15.00000000000000000 ) ) ;
#14435=ORIENTED_EDGE ( 'NONE', *, *, #20600, .F. ) ;
#14437=ADVANCED_FACE ( 'NONE', ( #15229 ), #21963, .T. ) ;
#14439=CARTESIAN_POINT ( 'NONE',  ( 109.3255224386495001, 254.7368901578298050, 35.86658157783330836 ) ) ;
#14440=EDGE_LOOP ( 'NONE', ( #12249, #25836, #24537, #21664 ) ) ;
#14441=CIRCLE ( 'NONE', #24994, 2.000000000000012879 ) ;
#14442=ORIENTED_EDGE ( 'NONE', *, *, #11141, .F. ) ;
#14446=ORIENTED_EDGE ( 'NONE', *, *, #24142, .T. ) ;
#14450=DIRECTION ( 'NONE',  ( 0.8018642810807399268, 0.5975062131282553590, 0.000000000000000000 ) ) ;
#14452=CARTESIAN_POINT ( 'NONE',  ( -43.02437977270766822, 129.7200458115293031, -16.81627168235288394 ) ) ;
#14453=CARTESIAN_POINT ( 'NONE',  ( 109.9999999999999432, -100.0000000000000142, 25.00000000000000000 ) ) ;
#14458=CARTESIAN_POINT ( 'NONE',  ( 65.00000000000000000, -120.0000000000000995, -63.97499999999998721 ) ) ;
#14459=CARTESIAN_POINT ( 'NONE',  ( -270.1025481742786951, -91.18033988749901653, 14.95564396479129243 ) ) ;
#14462=CARTESIAN_POINT ( 'NONE',  ( 101.0657985141824611, 243.3257530605124543, -15.10239625482412507 ) ) ;
#14463=CARTESIAN_POINT ( 'NONE',  ( 15.23471640472432043, 89.54451151409071485, 98.44134334489216087 ) ) ;
#14467=ADVANCED_FACE ( 'NONE', ( #13218 ), #27330, .T. ) ;
#14469=CARTESIAN_POINT ( 'NONE',  ( -68.57415822541635464, -18.01420295945611727, 80.00000000000001421 ) ) ;
#14472=ORIENTED_EDGE ( 'NONE', *, *, #3474, .F. ) ;
#14476=CARTESIAN_POINT ( 'NONE',  ( -75.08089385218988809, 136.1113822420730912, 13.54512463695272650 ) ) ;
#14484=DIRECTION ( 'NONE',  ( -8.673617379884036705E-17, 1.000000000000000000, 0.000000000000000000 ) ) ;
#14485=EDGE_CURVE ( 'NONE', #23195, #25296, #25053, .T. ) ;
#14493=DIRECTION ( 'NONE',  ( -0.000000000000000000, -0.000000000000000000, 1.000000000000000000 ) ) ;
#14499=CARTESIAN_POINT ( 'NONE',  ( 99.60675733924797726, 85.63108538499818678, -100.0000000000000284 ) ) ;
#14503=DIRECTION ( 'NONE',  ( 0.000000000000000000, 0.000000000000000000, 1.000000000000000000 ) ) ;
#14506=ADVANCED_FACE ( 'NONE', ( #14348 ), #3126, .F. ) ;
#14508=VERTEX_POINT ( 'NONE', #12201 ) ;
#14509=VECTOR ( 'NONE', #10450, 1000.000000000000000 ) ;
#14513=CARTESIAN_POINT ( 'NONE',  ( -203.2481855153402250, 92.57460631283319685, 29.78692811926998729 ) ) ;
#14514=FACE_BOUND ( 'NONE', #16474, .T. ) ;
#14516=FACE_OUTER_BOUND ( 'NONE', #14161, .T. ) ;
#14520=DIRECTION ( 'NONE',  ( -1.000000000000000000, 0.000000000000000000, 0.000000000000000000 ) ) ;
#14521=FACE_OUTER_BOUND ( 'NONE', #8170, .T. ) ;
#14524=DIRECTION ( 'NONE',  ( 0.000000000000000000, 1.000000000000000000, 0.000000000000000000 ) ) ;
#14529=CARTESIAN_POINT ( 'NONE',  ( -189.6824478863817092, 103.6171365956006980, 32.45239274750386471 ) ) ;
#14536=CARTESIAN_POINT ( 'NONE',  ( 114.5273445118512967, 107.2595481030940476, 100.0000000000000142 ) ) ;
#14537=EDGE_CURVE ( 'NONE', #19657, #9810, #22805, .T. ) ;
#14545=EDGE_CURVE ( 'NONE', #25901, #6225, #2092, .T. ) ;
#14546=CARTESIAN_POINT ( 'NONE',  ( 116.3389527601132869, 113.0483370489294543, 100.0000000000000142 ) ) ;
#14552=ADVANCED_FACE ( 'NONE', ( #25112 ), #20805, .F. ) ;
#14554=DIRECTION ( 'NONE',  ( 0.000000000000000000, 0.000000000000000000, -1.000000000000000000 ) ) ;
#14560=DIRECTION ( 'NONE',  ( -0.000000000000000000, 1.000000000000000000, -1.387778780781445429E-16 ) ) ;
#14565=ORIENTED_EDGE ( 'NONE', *, *, #15870, .F. ) ;
#14567=CARTESIAN_POINT ( 'NONE',  ( 89.99999999999994316, -90.00000000000001421, -25.00000000000000711 ) ) ;
#14569=VERTEX_POINT ( 'NONE', #5429 ) ;
#14570=LINE ( 'NONE', #1348, #28044 ) ;
#14578=DIRECTION ( 'NONE',  ( -1.000000000000000000, 0.000000000000000000, -0.000000000000000000 ) ) ;
#14582=ORIENTED_EDGE ( 'NONE', *, *, #27850, .T. ) ;
#14585=VECTOR ( 'NONE', #16259, 1000.000000000000000 ) ;
#14591=CARTESIAN_POINT ( 'NONE',  ( -226.8880901706862971, 73.06320664976456669, -17.43415524067905409 ) ) ;
#14596=CARTESIAN_POINT ( 'NONE',  ( -175.0000000000000000, -150.0000000000000853, 70.00000000000001421 ) ) ;
#14597=VERTEX_POINT ( 'NONE', #10743 ) ;
#14599=CARTESIAN_POINT ( 'NONE',  ( 109.9161154791872690, 257.8825900702938725, -41.33255568694282545 ) ) ;
#14608=VECTOR ( 'NONE', #16849, 1000.000000000000000 ) ;
#14611=CARTESIAN_POINT ( 'NONE',  ( -47.63323754515640474, 132.2630729665446836, 15.94942322957973069 ) ) ;
#14613=ORIENTED_EDGE ( 'NONE', *, *, #26281, .T. ) ;
#14617=FACE_OUTER_BOUND ( 'NONE', #22445, .T. ) ;
#14619=DIRECTION ( 'NONE',  ( 0.000000000000000000, 0.000000000000000000, -1.000000000000000000 ) ) ;
#14622=DIRECTION ( 'NONE',  ( 0.000000000000000000, 0.000000000000000000, -1.000000000000000000 ) ) ;
#14623=DIRECTION ( 'NONE',  ( 1.000000000000000000, 1.530283246943720875E-16, -0.000000000000000000 ) ) ;
#14629=CARTESIAN_POINT ( 'NONE',  ( -230.9590218388320295, 90.04903060735585996, 15.10580296129862177 ) ) ;
#14630=CARTESIAN_POINT ( 'NONE',  ( -43.02437977270766822, 129.7200458115292747, 16.81627168235289815 ) ) ;
#14637=ORIENTED_EDGE ( 'NONE', *, *, #2510, .T. ) ;
#14638=ADVANCED_FACE ( 'NONE', ( #19211 ), #8301, .F. ) ;
#14641=CARTESIAN_POINT ( 'NONE',  ( 100.3999191023820003, 235.3978472240765711, -22.98606999220681857 ) ) ;
#14648=ORIENTED_EDGE ( 'NONE', *, *, #16275, .T. ) ;
#14649=ORIENTED_EDGE ( 'NONE', *, *, #11782, .F. ) ;
#14651=FACE_OUTER_BOUND ( 'NONE', #24603, .T. ) ;
#14652=CARTESIAN_POINT ( 'NONE',  ( -270.1025481742786951, -91.18033988749901653, 0.000000000000000000 ) ) ;
#14656=CARTESIAN_POINT ( 'NONE',  ( -17.24491960465745777, 0.000000000000000000, 100.0000000000000000 ) ) ;
#14671=EDGE_CURVE ( 'NONE', #2370, #4186, #26092, .T. ) ;
#14676=DIRECTION ( 'NONE',  ( -0.000000000000000000, 1.000000000000000000, -1.387778780781445429E-16 ) ) ;
#14682=CARTESIAN_POINT ( 'NONE',  ( 79.99999999999992895, 110.0000000000000000, 70.00000000000001421 ) ) ;
#14684=CARTESIAN_POINT ( 'NONE',  ( -184.1653517315182569, 107.3698090412221404, -31.09403837874923582 ) ) ;
#14694=CARTESIAN_POINT ( 'NONE',  ( -192.2868888506042708, 101.5231402318620582, -32.81226276753037041 ) ) ;
#14699=CARTESIAN_POINT ( 'NONE',  ( -160.0000000000000284, 59.99999999999994316, -15.00000000000000000 ) ) ;
#14703=CARTESIAN_POINT ( 'NONE',  ( 117.2367070128591990, 233.8218819039115886, 99.61792820886471134 ) ) ;
#14706=CARTESIAN_POINT ( 'NONE',  ( -170.0252337835103162, 115.7161349404674411, 25.41356568217192802 ) ) ;
#14708=CARTESIAN_POINT ( 'NONE',  ( -205.2925087133504860, 91.43105200015486389, 27.40227028352467897 ) ) ;
#14712=ADVANCED_FACE ( 'NONE', ( #21797 ), #26510, .T. ) ;
#14713=ORIENTED_EDGE ( 'NONE', *, *, #13484, .T. ) ;
#14717=ADVANCED_FACE ( 'NONE', ( #2670 ), #3509, .F. ) ;
#14725=VERTEX_POINT ( 'NONE', #15771 ) ;
#14727=AXIS2_PLACEMENT_3D ( 'NONE', #13058, #24235, #13332 ) ;
#14729=CARTESIAN_POINT ( 'NONE',  ( -68.57415822541635464, 24.64876300893806160, 95.00000000000000000 ) ) ;
#14731=CARTESIAN_POINT ( 'NONE',  ( 89.99999999999994316, -70.00000000000001421, -70.00000000000001421 ) ) ;
#14732=DIRECTION ( 'NONE',  ( 0.000000000000000000, 0.000000000000000000, 1.000000000000000000 ) ) ;
#14733=CARTESIAN_POINT ( 'NONE',  ( -244.5479615644635487, 75.99513337129094737, -5.000000000000002665 ) ) ;
#14738=CARTESIAN_POINT ( 'NONE',  ( 115.6411010564591777, 231.4666050640012429, -99.00000000000001421 ) ) ;
#14739=ORIENTED_EDGE ( 'NONE', *, *, #27962, .T. ) ;
#14745=PLANE ( 'NONE',  #17216 ) ;
#14748=ORIENTED_EDGE ( 'NONE', *, *, #10910, .F. ) ;
#14751=DIRECTION ( 'NONE',  ( 0.000000000000000000, 1.000000000000000000, 0.000000000000000000 ) ) ;
#14756=VERTEX_POINT ( 'NONE', #27362 ) ;
#14757=DIRECTION ( 'NONE',  ( 0.000000000000000000, 0.000000000000000000, 1.000000000000000000 ) ) ;
#14760=CARTESIAN_POINT ( 'NONE',  ( 112.7775258882239910, 216.4408397934976449, 96.91707758366527514 ) ) ;
#14763=VECTOR ( 'NONE', #2242, 1000.000000000000000 ) ;
#14764=CARTESIAN_POINT ( 'NONE',  ( -152.9413447092802869, 123.6266336979618785, -18.69402831667922626 ) ) ;
#14765=CIRCLE ( 'NONE', #20253, 50.00000000000000000 ) ;
#14766=VECTOR ( 'NONE', #25120, 1000.000000000000000 ) ;
#14769=CARTESIAN_POINT ( 'NONE',  ( 29.75659119584032908, -42.58214737927222160, 99.89076439235542182 ) ) ;
#14770=CARTESIAN_POINT ( 'NONE',  ( -218.9419962481124742, 86.22404402610023055, -19.29714585459672094 ) ) ;
#14777=EDGE_CURVE ( 'NONE', #13271, #21857, #4966, .T. ) ;
#14779=CARTESIAN_POINT ( 'NONE',  ( -71.37541315349507443, 150.2892445414773590, 15.00000000000000000 ) ) ;
#14784=CARTESIAN_POINT ( 'NONE',  ( 96.75280658369999287, 240.7143248587423159, -19.91790936281032032 ) ) ;
#14786=ORIENTED_EDGE ( 'NONE', *, *, #5201, .F. ) ;
#14796=DIRECTION ( 'NONE',  ( 0.000000000000000000, 0.000000000000000000, -1.000000000000000000 ) ) ;
#14797=DIRECTION ( 'NONE',  ( 0.000000000000000000, 2.498359269027536814E-16, -1.000000000000000000 ) ) ;
#14798=ADVANCED_FACE ( 'NONE', ( #22654 ), #15914, .T. ) ;
#14800=CARTESIAN_POINT ( 'NONE',  ( -17.95129507155921544, 128.7178007427875457, -17.19838318425743040 ) ) ;
#14801=EDGE_CURVE ( 'NONE', #20650, #25890, #14177, .T. ) ;
#14802=AXIS2_PLACEMENT_3D ( 'NONE', #2174, #6347, #4465 ) ;
#14805=CARTESIAN_POINT ( 'NONE',  ( -63.57415822541634043, -18.01420295945611727, 95.00000000000000000 ) ) ;
#14807=CARTESIAN_POINT ( 'NONE',  ( -208.5031313904178774, 74.88898109331546493, -38.37316925720519833 ) ) ;
#14808=AXIS2_PLACEMENT_3D ( 'NONE', #7331, #11510, #581 ) ;
#14811=DIRECTION ( 'NONE',  ( -1.000000000000000000, 0.000000000000000000, 0.000000000000000000 ) ) ;
#14815=CARTESIAN_POINT ( 'NONE',  ( 115.6411010564591777, 231.4666050640012429, -99.00000000000001421 ) ) ;
#14822=EDGE_CURVE ( 'NONE', #17042, #1725, #9443, .T. ) ;
#14826=CARTESIAN_POINT ( 'NONE',  ( -125.2895325436292069, 200.2180533211636657, 15.00000000000000000 ) ) ;
#14832=CARTESIAN_POINT ( 'NONE',  ( 105.5625267348463581, 242.0882338934268887, 29.27839960683066067 ) ) ;
#14833=CARTESIAN_POINT ( 'NONE',  ( -188.7053934046000734, 104.3037723739169991, -31.95410354694828925 ) ) ;
#14835=CARTESIAN_POINT ( 'NONE',  ( 99.60675733924549036, 85.63108538499666622, 100.0000000000000142 ) ) ;
#14836=ORIENTED_EDGE ( 'NONE', *, *, #1009, .F. ) ;
#14837=CARTESIAN_POINT ( 'NONE',  ( -248.1546605714623013, -91.18033988749901653, -10.70611877156249214 ) ) ;
#14839=FACE_OUTER_BOUND ( 'NONE', #13888, .T. ) ;
#14841=EDGE_CURVE ( 'NONE', #10216, #16435, #7570, .T. ) ;
#14843=EDGE_CURVE ( 'NONE', #25070, #16727, #26915, .T. ) ;
#14855=DIRECTION ( 'NONE',  ( 3.469446951953614189E-16, -1.000000000000000000, 0.000000000000000000 ) ) ;
#14856=DIRECTION ( 'NONE',  ( 1.000000000000000000, 0.000000000000000000, 0.000000000000000000 ) ) ;
#14857=FACE_OUTER_BOUND ( 'NONE', #17527, .T. ) ;
#14860=DIRECTION ( 'NONE',  ( 1.000000000000000000, 0.000000000000000000, 0.000000000000000000 ) ) ;
#14861=CYLINDRICAL_SURFACE ( 'NONE', #15264, 30.00000000000000000 ) ;
#14863=DIRECTION ( 'NONE',  ( -0.000000000000000000, 1.000000000000000000, -1.387778780781445429E-16 ) ) ;
#14864=CARTESIAN_POINT ( 'NONE',  ( -199.1750262236165270, 96.10583454779617796, -31.38733092741667008 ) ) ;
#14868=ORIENTED_EDGE ( 'NONE', *, *, #26220, .F. ) ;
#14871=PRODUCT ( 'Structural Component', 'Structural Component', '', ( #24001 ) ) ;
#14873=VERTEX_POINT ( 'NONE', #12023 ) ;
#14876=CARTESIAN_POINT ( 'NONE',  ( 6.333040578238042784, 140.1900314533376388, 13.00000000000000355 ) ) ;
#14879=EDGE_CURVE ( 'NONE', #10475, #25995, #21854, .T. ) ;
#14882=CARTESIAN_POINT ( 'NONE',  ( -236.2188936947904381, 81.35702876104954839, -15.00000000000000178 ) ) ;
#14883=ORIENTED_EDGE ( 'NONE', *, *, #13884, .F. ) ;
#14895=CIRCLE ( 'NONE', #21753, 79.71075545852265520 ) ;
#14902=CARTESIAN_POINT ( 'NONE',  ( -52.43980137721120371, 133.2615281902219238, 14.19467156484360082 ) ) ;
#14903=ORIENTED_EDGE ( 'NONE', *, *, #20444, .T. ) ;
#14904=ORIENTED_EDGE ( 'NONE', *, *, #9189, .F. ) ;
#14906=AXIS2_PLACEMENT_3D ( 'NONE', #165, #26162, #2448 ) ;
#14907=CARTESIAN_POINT ( 'NONE',  ( -175.0000000000000000, -150.0000000000000853, -75.99999999999998579 ) ) ;
#14909=CARTESIAN_POINT ( 'NONE',  ( -122.9571926194021501, 132.7586943017250007, -14.33743497904945485 ) ) ;
#14911=ADVANCED_FACE ( 'NONE', ( #7281 ), #24661, .F. ) ;
#14914=CARTESIAN_POINT ( 'NONE',  ( -209.6054486774690133, 88.33790154040774212, -25.57920806210336551 ) ) ;
#14921=ORIENTED_EDGE ( 'NONE', *, *, #13967, .T. ) ;
#14922=CARTESIAN_POINT ( 'NONE',  ( 113.8545328002507659, 140.0000000000000284, 97.99666842398181643 ) ) ;
#14928=CIRCLE ( 'NONE', #2513, 22.49999999999997868 ) ;
#14929=CARTESIAN_POINT ( 'NONE',  ( 98.38712641049866647, 233.7235291372444692, -21.27834768225378426 ) ) ;
#14930=EDGE_LOOP ( 'NONE', ( #27102, #16826, #18638, #19480 ) ) ;
#14933=EDGE_LOOP ( 'NONE', ( #26189, #8987, #3592, #20419 ) ) ;
#14936=EDGE_LOOP ( 'NONE', ( #7264, #11071, #9571, #15057 ) ) ;
#14941=VECTOR ( 'NONE', #2201, 1000.000000000000000 ) ;
#14943=CARTESIAN_POINT ( 'NONE',  ( 106.6902583091410719, 244.3125670946242849, -31.28102666700890211 ) ) ;
#14949=CARTESIAN_POINT ( 'NONE',  ( -227.3081281289699973, 73.26923787007372368, -17.24424915250854085 ) ) ;
#14951=CARTESIAN_POINT ( 'NONE',  ( -33.92892658514118409, 128.1932174690772683, 17.41923701875080965 ) ) ;
#14952=CARTESIAN_POINT ( 'NONE',  ( -40.40953891503691153, 0.000000000000000000, 100.0000000000000000 ) ) ;
#14956=CARTESIAN_POINT ( 'NONE',  ( -163.7740599641838912, 118.1414984323162258, 24.33163590040494739 ) ) ;
#14961=EDGE_LOOP ( 'NONE', ( #12012, #22880, #7183, #6363, #20145 ) ) ;
#14963=ADVANCED_FACE ( 'NONE', ( #16882 ), #14987, .T. ) ;
#14964=ORIENTED_EDGE ( 'NONE', *, *, #6976, .T. ) ;
#14970=CARTESIAN_POINT ( 'NONE',  ( 95.20156243613460845, 83.09913198707280912, -100.0000000000000284 ) ) ;
#14971=ADVANCED_FACE ( 'NONE', ( #3659 ), #27786, .T. ) ;
#14972=CARTESIAN_POINT ( 'NONE',  ( 65.00000000000000000, -120.0000000000000711, 70.00000000000001421 ) ) ;
#14975=CARTESIAN_POINT ( 'NONE',  ( -213.6112859001962363, 88.11147169443837868, 20.55567103321151734 ) ) ;
#14976=ORIENTED_EDGE ( 'NONE', *, *, #27994, .F. ) ;
#14982=B_SPLINE_CURVE_WITH_KNOTS ( 'NONE', 3,
 ( #9477, #24978, #22825, #26981, #11640, #20803, #16640, #9890, #2990, #27125, #5427, #3125, #18372, #20521, #2848, #980, #27259, #10031, #25253, #14212, #11781, #7458, #24839, #11919, #25395, #20941, #22960, #7734 ),
 .UNSPECIFIED., .F., .F.,
 ( 4, 2, 2, 2, 2, 2, 2, 2, 2, 2, 2, 2, 2, 4 ),
 ( 0.000000000000000000, 0.01515445388940273724, 0.03030890777880547449, 0.04546336166820825336, 0.05304058861290963933, 0.05682920208526034273, 0.06061781555761103224, 0.07577226944701370703, 0.09092672333641636795, 0.09850395028111769147, 0.1060811772258190289, 0.1098697906981696837, 0.1136584041705203107, 0.1212356311152215788 ),
 .UNSPECIFIED. ) ;
#14984=EDGE_CURVE ( 'NONE', #1752, #15077, #2586, .T. ) ;
#14987=TOROIDAL_SURFACE ( 'NONE', #9480, 18.46313063346208239, 2.000000000000000000 ) ;
#14993=CARTESIAN_POINT ( 'NONE',  ( -188.8008884155350131, 104.2369363794606443, 31.96258592612735683 ) ) ;
#14994=CARTESIAN_POINT ( 'NONE',  ( 49.56615429303207065, 203.2034914284457159, -13.00000000000000000 ) ) ;
#15000=EDGE_CURVE ( 'NONE', #5063, #15968, #1372, .T. ) ;
#15002=CARTESIAN_POINT ( 'NONE',  ( -183.2595802227681361, 107.9574575171763655, -30.83290447571683046 ) ) ;
#15003=ORIENTED_EDGE ( 'NONE', *, *, #14051, .F. ) ;
#15007=ORIENTED_EDGE ( 'NONE', *, *, #9979, .F. ) ;
#15011=CARTESIAN_POINT ( 'NONE',  ( 9.345921402568901470, 140.0000000000000000, 15.00000000000000000 ) ) ;
#15016=DIRECTION ( 'NONE',  ( -0.000000000000000000, -0.000000000000000000, 1.000000000000000000 ) ) ;
#15017=CARTESIAN_POINT ( 'NONE',  ( -230.6117145417363190, 64.61843588005640981, -16.59905221104221695 ) ) ;
#15020=DIRECTION ( 'NONE',  ( 0.4767408570798813972, -0.8790438869537404720, 0.000000000000000000 ) ) ;
#15023=CIRCLE ( 'NONE', #2615, 5.000000000000000888 ) ;
#15024=VERTEX_POINT ( 'NONE', #9998 ) ;
#15025=DIRECTION ( 'NONE',  ( 0.000000000000000000, 0.000000000000000000, 1.000000000000000000 ) ) ;
#15026=TOROIDAL_SURFACE ( 'NONE', #17755, 60.59270260175150469, 2.000000000000000000 ) ;
#15031=ORIENTED_EDGE ( 'NONE', *, *, #20903, .T. ) ;
#15033=ORIENTED_EDGE ( 'NONE', *, *, #6008, .T. ) ;
#15034=LINE ( 'NONE', #24499, #21825 ) ;
#15036=ORIENTED_EDGE ( 'NONE', *, *, #26998, .T. ) ;
#15042=DIRECTION ( 'NONE',  ( -0.000000000000000000, -0.000000000000000000, 1.000000000000000000 ) ) ;
#15043=VECTOR ( 'NONE', #14341, 1000.000000000000000 ) ;
#15044=PLANE ( 'NONE',  #26556 ) ;
#15046=CARTESIAN_POINT ( 'NONE',  ( -147.5692307249372277, 124.5789548200514218, -19.26288188869894924 ) ) ;
#15047=B_SPLINE_CURVE_WITH_KNOTS ( 'NONE', 3,
 ( #3968, #1536, #28091, #12755, #10304, #21357, #8291, #17325, #17045, #2095, #25805, #23800, #19341, #19489, #19628, #24088, #21494, #1811, #8436, #23942, #6131, #19063, #17190, #10587, #25949, #10871, #27808, #16908 ),
 .UNSPECIFIED., .F., .F.,
 ( 4, 2, 2, 2, 2, 2, 2, 2, 2, 2, 2, 2, 2, 4 ),
 ( 0.000000000000000000, 0.007596912630457928854, 0.01139536894568684774, 0.01519382526091576577, 0.02279073789137358100, 0.03038765052183138929, 0.04558147578274701628, 0.06077530104366264674, 0.06457375735889157864, 0.06837221367412052442, 0.07596912630457833271, 0.09116295156549394929, 0.1063567768264095659, 0.1215506020873251825 ),
 .UNSPECIFIED. ) ;
#15048=DIRECTION ( 'NONE',  ( 0.000000000000000000, 0.000000000000000000, 1.000000000000000000 ) ) ;
#15051=CARTESIAN_POINT ( 'NONE',  ( -223.8731558706656699, 88.82041552423905273, -14.63364721595453233 ) ) ;
#15057=ORIENTED_EDGE ( 'NONE', *, *, #11069, .F. ) ;
#15061=CARTESIAN_POINT ( 'NONE',  ( -40.40953891503691153, 0.000000000000000000, 99.00000000000000000 ) ) ;
#15062=FACE_OUTER_BOUND ( 'NONE', #16136, .T. ) ;
#15063=DIRECTION ( 'NONE',  ( 0.000000000000000000, 0.000000000000000000, 1.000000000000000000 ) ) ;
#15064=( BOUNDED_SURFACE ( )  B_SPLINE_SURFACE ( 3, 2, ( 
 ( #9206, #26426, #24284 ),
 ( #20257, #26571, #15679 ),
 ( #7047, #11367, #303 ),
 ( #15967, #15536, #24858 ),
 ( #13814, #24428, #2728 ),
 ( #11075, #13523, #728 ),
 ( #22564, #24716, #17966 ),
 ( #9498, #20400, #11222 ),
 ( #9059, #8919, #11664 ),
 ( #18253, #27005, #9353 ),
 ( #22274, #7194, #26717 ),
 ( #15829, #22128, #16108 ),
 ( #5172, #24572, #18112 ),
 ( #4883, #2872, #19829 ),
 ( #157, #17673, #4592 ),
 ( #13378, #12328, #19058 ),
 ( #8140, #5704, #5979 ),
 ( #18392, #12467, #17040 ),
 ( #6127, #23365, #8002 ),
 ( #27145, #21068, #10299 ),
 ( #6263, #7479, #16249 ),
 ( #24997, #28084, #3678 ),
 ( #25800, #1391, #14476 ),
 ( #23654, #3964, #23233 ),
 ( #20540, #3535, #16769 ),
 ( #10160, #3009, #14902 ),
 ( #21207, #14611, #25521 ),
 ( #25654, #12750, #18914 ) ),
 .UNSPECIFIED., .F., .F., .T. ) 
 B_SPLINE_SURFACE_WITH_KNOTS ( ( 4, 2, 2, 2, 2, 2, 2, 2, 2, 2, 2, 2, 2, 4 ),
 ( 3, 3 ),
 ( 0.000000000000000000, 0.007529199611455438673, 0.01505839922291087735, 0.02258759883436631602, 0.02635219864009403362, 0.03011679844582175469, 0.04517519766873263204, 0.06023359689164350939, 0.07529199611455439367, 0.07905659592028210780, 0.08282119572600982194, 0.09035039533746526408, 0.1054087945603761345, 0.1204671937832870188 ),
 ( 0.000000000000000000, 1.000000000000000000 ),
 .UNSPECIFIED. ) 
 GEOMETRIC_REPRESENTATION_ITEM ( )  RATIONAL_B_SPLINE_SURFACE ( (
 ( 1.000000000000000000, 0.8981184559478656571, 1.000000000000000000),
 ( 1.000000000000000000, 0.8913409640699760939, 1.000000000000000000),
 ( 1.000000000000000000, 0.8845625463580112369, 1.000000000000000000),
 ( 1.000000000000000000, 0.8711578316887859108, 1.000000000000000000),
 ( 1.000000000000000000, 0.8645314129694308125, 1.000000000000000000),
 ( 1.000000000000000000, 0.8515750003171709270, 1.000000000000000000),
 ( 1.000000000000000000, 0.8452448728250648857, 1.000000000000000000),
 ( 1.000000000000000000, 0.8360775906454407380, 1.000000000000000000),
 ( 1.000000000000000000, 0.8330764670878353373, 1.000000000000000000),
 ( 1.000000000000000000, 0.8272009908158640679, 1.000000000000000000),
 ( 1.000000000000000000, 0.8243270960686099880, 1.000000000000000000),
 ( 1.000000000000000000, 0.8103905206081341017, 1.000000000000000000),
 ( 1.000000000000000000, 0.8005641981319898681, 1.000000000000000000),
 ( 1.000000000000000000, 0.7842823063492941893, 1.000000000000000000),
 ( 1.000000000000000000, 0.7778294879052323196, 1.000000000000000000),
 ( 1.000000000000000000, 0.7688627540743353528, 1.000000000000000000),
 ( 1.000000000000000000, 0.7663513471414680200, 1.000000000000000000),
 ( 1.000000000000000000, 0.7658761447369581976, 1.000000000000000000),
 ( 1.000000000000000000, 0.7659136159393603593, 1.000000000000000000),
 ( 1.000000000000000000, 0.7662557092201324194, 1.000000000000000000),
 ( 1.000000000000000000, 0.7665607478393150487, 1.000000000000000000),
 ( 1.000000000000000000, 0.7678709653268237512, 1.000000000000000000),
 ( 1.000000000000000000, 0.7692719988712057866, 1.000000000000000000),
 ( 1.000000000000000000, 0.7749914125728452063, 1.000000000000000000),
 ( 1.000000000000000000, 0.7808328044829244696, 1.000000000000000000),
 ( 1.000000000000000000, 0.7960310293872467913, 1.000000000000000000),
 ( 1.000000000000000000, 0.8053828549108267287, 1.000000000000000000),
 ( 1.000000000000000000, 0.8161343730438193056, 1.000000000000000000) ) ) 
 REPRESENTATION_ITEM ( '' )  SURFACE ( )  );
#15066=CARTESIAN_POINT ( 'NONE',  ( 104.4928295061288281, 246.1605864358141673, -20.56267333362882255 ) ) ;
#15068=CARTESIAN_POINT ( 'NONE',  ( -273.6211430000234373, -91.18033988749901653, 0.000000000000000000 ) ) ;
#15071=ORIENTED_EDGE ( 'NONE', *, *, #18828, .F. ) ;
#15074=VECTOR ( 'NONE', #9866, 1000.000000000000000 ) ;
#15077=VERTEX_POINT ( 'NONE', #4497 ) ;
#15079=DIRECTION ( 'NONE',  ( -1.224646799147353207E-16, 1.000000000000000000, 0.000000000000000000 ) ) ;
#15084=CARTESIAN_POINT ( 'NONE',  ( 65.00000000000000000, -150.0000000000000568, -64.00000000000000000 ) ) ;
#15087=CARTESIAN_POINT ( 'NONE',  ( -236.8177751472017007, 82.33896643611701904, -15.00000000000000000 ) ) ;
#15088=CARTESIAN_POINT ( 'NONE',  ( -24.75943805428697786, 129.2472029784736662, 15.64972235346578167 ) ) ;
#15089=VECTOR ( 'NONE', #10210, 1000.000000000000000 ) ;
#15095=ADVANCED_FACE ( 'NONE', ( #6669 ), #15448, .T. ) ;
#15101=ORIENTED_EDGE ( 'NONE', *, *, #8298, .T. ) ;
#15108=ADVANCED_FACE ( 'NONE', ( #1924 ), #2486, .F. ) ;
#15109=ORIENTED_EDGE ( 'NONE', *, *, #12775, .T. ) ;
#15111=CARTESIAN_POINT ( 'NONE',  ( 109.5756401947800356, 134.3783162856662159, -100.0000000000000142 ) ) ;
#15113=CARTESIAN_POINT ( 'NONE',  ( 92.44907173541768941, 230.7276239336879371, 17.70004142540128456 ) ) ;
#15117=CARTESIAN_POINT ( 'NONE',  ( -216.2392880859841284, 87.80609967497970558, 20.45738389094162457 ) ) ;
#15118=VERTEX_POINT ( 'NONE', #28204 ) ;
#15121=CARTESIAN_POINT ( 'NONE',  ( 90.00000000000042633, 230.0000000000000284, -6.270166537925968342 ) ) ;
#15126=FACE_BOUND ( 'NONE', #22377, .T. ) ;
#15127=CARTESIAN_POINT ( 'NONE',  ( -21.33210486176665910, 0.000000000000000000, 99.00000000000000000 ) ) ;
#15130=ORIENTED_EDGE ( 'NONE', *, *, #8022, .F. ) ;
#15134=DIRECTION ( 'NONE',  ( -0.000000000000000000, -0.000000000000000000, -1.000000000000000000 ) ) ;
#15135=CARTESIAN_POINT ( 'NONE',  ( -226.7417855643314226, 89.97934261517927723, 13.71636754133556302 ) ) ;
#15138=CARTESIAN_POINT ( 'NONE',  ( -63.57415822541634043, 80.97823757117562593, 95.00000000000000000 ) ) ;
#15142=CARTESIAN_POINT ( 'NONE',  ( -187.2788549371262832, 105.2860637900685674, -32.19960561888341743 ) ) ;
#15145=CARTESIAN_POINT ( 'NONE',  ( -68.57415822541635464, 75.97823757117562593, 80.00000000000001421 ) ) ;
#15146=VERTEX_POINT ( 'NONE', #19882 ) ;
#15155=DIRECTION ( 'NONE',  ( 0.9960550913260672878, 0.000000000000000000, -0.08873699929240054518 ) ) ;
#15163=CARTESIAN_POINT ( 'NONE',  ( -237.6054256748464013, 69.18099216265484586, -14.87827728787998538 ) ) ;
#15175=DIRECTION ( 'NONE',  ( 1.000000000000000000, 0.000000000000000000, 0.000000000000000000 ) ) ;
#15177=TOROIDAL_SURFACE ( 'NONE', #6898, 421.5408555545579929, 7.500000000000000000 ) ;
#15184=DIRECTION ( 'NONE',  ( 0.000000000000000000, 0.000000000000000000, 1.000000000000000000 ) ) ;
#15186=EDGE_CURVE ( 'NONE', #3239, #14756, #27886, .T. ) ;
#15188=VERTEX_POINT ( 'NONE', #17583 ) ;
#15189=CARTESIAN_POINT ( 'NONE',  ( -227.8378063125350650, 130.6400894613934724, 15.00000000000001954 ) ) ;
#15190=CARTESIAN_POINT ( 'NONE',  ( 134.9999999999998579, 220.0000000000000284, 84.99999999999995737 ) ) ;
#15194=CARTESIAN_POINT ( 'NONE',  ( 139.9999999999999432, -90.00000000000000000, -70.00000000000001421 ) ) ;
#15196=CARTESIAN_POINT ( 'NONE',  ( -214.1881881672503312, 87.99490168924762656, -20.10759990481813375 ) ) ;
#15201=DIRECTION ( 'NONE',  ( 1.000000000000000000, 0.000000000000000000, 0.000000000000000000 ) ) ;
#15207=AXIS2_PLACEMENT_3D ( 'NONE', #7772, #16677, #13977 ) ;
#15208=CARTESIAN_POINT ( 'NONE',  ( 109.9999999999999005, 140.0000000000000284, 91.30899693899577585 ) ) ;
#15213=CARTESIAN_POINT ( 'NONE',  ( 98.38958437017922165, 241.8303606468361409, -11.96405203492589564 ) ) ;
#15215=CARTESIAN_POINT ( 'NONE',  ( 0.6789813131199424756, 136.5995534334086301, -13.39369412120168157 ) ) ;
#15222=( GEOMETRIC_REPRESENTATION_CONTEXT ( 3 ) GLOBAL_UNCERTAINTY_ASSIGNED_CONTEXT ( ( #19802 ) ) GLOBAL_UNIT_ASSIGNED_CONTEXT ( ( #6958, #22483, #11581 ) ) REPRESENTATION_CONTEXT ( 'NONE', 'WORKASPACE' ) );
#15223=FACE_OUTER_BOUND ( 'NONE', #23997, .T. ) ;
#15225=CARTESIAN_POINT ( 'NONE',  ( 65.00000000000000000, -120.0000000000000711, 70.00000000000001421 ) ) ;
#15229=FACE_OUTER_BOUND ( 'NONE', #997, .T. ) ;
#15231=ADVANCED_FACE ( 'NONE', ( #917 ), #5224, .F. ) ;
#15233=DIRECTION ( 'NONE',  ( 1.000000000000000000, 0.000000000000000000, 0.000000000000000000 ) ) ;
#15245=CARTESIAN_POINT ( 'NONE',  ( -178.8123904115888934, 110.7331632632894411, 29.85040004129419700 ) ) ;
#15246=AXIS2_PLACEMENT_3D ( 'NONE', #24922, #5517, #5091 ) ;
#15252=CARTESIAN_POINT ( 'NONE',  ( -160.8326600028555902, 120.2355194873575073, -21.37420696376537776 ) ) ;
#15256=CARTESIAN_POINT ( 'NONE',  ( 105.2480867104912790, 123.6573351778161793, -99.99999999997838529 ) ) ;
#15260=CARTESIAN_POINT ( 'NONE',  ( -229.0920485471770860, 88.91763133824811405, 15.43435999875618236 ) ) ;
#15262=AXIS2_PLACEMENT_3D ( 'NONE', #9148, #24366, #15483 ) ;
#15264=AXIS2_PLACEMENT_3D ( 'NONE', #3918, #7819, #21444 ) ;
#15282=CARTESIAN_POINT ( 'NONE',  ( 184.9999999999999147, -150.0000000000000284, 84.99999999999995737 ) ) ;
#15283=ORIENTED_EDGE ( 'NONE', *, *, #17292, .T. ) ;
#15285=CIRCLE ( 'NONE', #18941, 2.000000000000000444 ) ;
#15287=VECTOR ( 'NONE', #1211, 1000.000000000000000 ) ;
#15289=CARTESIAN_POINT ( 'NONE',  ( -189.4726776444009317, 103.5548156087989184, -32.83427761469911843 ) ) ;
#15291=EDGE_LOOP ( 'NONE', ( #19788, #16996, #26634, #21292 ) ) ;
#15292=CARTESIAN_POINT ( 'NONE',  ( -114.3540299464916785, 71.47411450562970003, 82.81256190651343729 ) ) ;
#15293=LINE ( 'NONE', #24048, #5213 ) ;
#15296=ORIENTED_EDGE ( 'NONE', *, *, #7986, .T. ) ;
#15299=CIRCLE ( 'NONE', #8423, 55.86582179324592090 ) ;
#15300=DIRECTION ( 'NONE',  ( 1.000000000000000000, 0.000000000000000000, 0.000000000000000000 ) ) ;
#15302=DIRECTION ( 'NONE',  ( 1.000000000000000000, 0.000000000000000000, 0.000000000000000000 ) ) ;
#15307=ORIENTED_EDGE ( 'NONE', *, *, #15000, .T. ) ;
#15316=DIRECTION ( 'NONE',  ( 0.000000000000000000, 0.000000000000000000, 1.000000000000000000 ) ) ;
#15323=AXIS2_PLACEMENT_3D ( 'NONE', #24317, #339, #4774 ) ;
#15324=CARTESIAN_POINT ( 'NONE',  ( -220.8227294558590756, 71.35641261643398536, 21.08939097871950707 ) ) ;
#15330=ORIENTED_EDGE ( 'NONE', *, *, #13307, .F. ) ;
#15336=CARTESIAN_POINT ( 'NONE',  ( 89.82706236705463709, 239.6935390653904392, 16.61376038146385170 ) ) ;
#15341=LINE ( 'NONE', #527, #12637 ) ;
#15342=CARTESIAN_POINT ( 'NONE',  ( -227.5045087581038388, 90.32113136995671709, -15.58012468608450440 ) ) ;
#15345=CARTESIAN_POINT ( 'NONE',  ( 134.9999999999998579, 220.0000000000000284, -84.99999999999997158 ) ) ;
#15348=VERTEX_POINT ( 'NONE', #7535 ) ;
#15357=CARTESIAN_POINT ( 'NONE',  ( 109.9999999999998863, 259.4346755187099802, -44.02082925162862637 ) ) ;
#15358=ORIENTED_EDGE ( 'NONE', *, *, #20845, .T. ) ;
#15364=EDGE_LOOP ( 'NONE', ( #28262, #517, #18738, #26117, #9086 ) ) ;
#15365=AXIS2_PLACEMENT_3D ( 'NONE', #23080, #1098, #27650 ) ;
#15368=CARTESIAN_POINT ( 'NONE',  ( -160.0000000000000284, 79.99999999999994316, 70.00000000000001421 ) ) ;
#15371=EDGE_CURVE ( 'NONE', #14295, #10017, #11392, .T. ) ;
#15373=CARTESIAN_POINT ( 'NONE',  ( -226.6109647992649059, 62.69877383610198507, 18.44381613006064313 ) ) ;
#15377=CIRCLE ( 'NONE', #4813, 55.86582179324592090 ) ;
#15379=DIRECTION ( 'NONE',  ( 1.000000000000000000, -9.102812259465213132E-16, 0.000000000000000000 ) ) ;
#15380=LINE ( 'NONE', #28134, #12533 ) ;
#15381=VECTOR ( 'NONE', #1008, 1000.000000000000114 ) ;
#15382=CARTESIAN_POINT ( 'NONE',  ( -160.0000000000000284, 109.9999999999999432, -70.00000000000001421 ) ) ;
#15384=CARTESIAN_POINT ( 'NONE',  ( -173.2089802904066573, 113.5335206920022273, 28.23679712238971007 ) ) ;
#15390=CARTESIAN_POINT ( 'NONE',  ( -203.2481855153402250, 92.57460631283319685, -29.78692811926999795 ) ) ;
#15391=VERTEX_POINT ( 'NONE', #14421 ) ;
#15397=ORIENTED_EDGE ( 'NONE', *, *, #16944, .F. ) ;
#15398=EDGE_CURVE ( 'NONE', #21416, #5481, #4220, .T. ) ;
#15399=CIRCLE ( 'NONE', #12187, 16.36034929305424512 ) ;
#15400=CARTESIAN_POINT ( 'NONE',  ( 93.07270601809125310, 112.9533406970419378, -100.0000000000000142 ) ) ;
#15404=CARTESIAN_POINT ( 'NONE',  ( -209.6027893482759907, 89.20079749152587567, 25.07826924335527607 ) ) ;
#15410=FACE_BOUND ( 'NONE', #26958, .T. ) ;
#15411=EDGE_CURVE ( 'NONE', #5960, #1808, #16573, .T. ) ;
#15412=AXIS2_PLACEMENT_3D ( 'NONE', #25588, #12405, #21682 ) ;
#15422=CARTESIAN_POINT ( 'NONE',  ( -140.5419864827275660, 71.17632247292569048, 82.82905917779648064 ) ) ;
#15426=ORIENTED_EDGE ( 'NONE', *, *, #5035, .F. ) ;
#15428=CARTESIAN_POINT ( 'NONE',  ( -178.3823435749502266, 110.6645840747622032, -30.26113312571055047 ) ) ;
#15429=ORIENTED_EDGE ( 'NONE', *, *, #2306, .T. ) ;
#15432=EDGE_CURVE ( 'NONE', #19721, #9863, #12325, .T. ) ;
#15433=DIRECTION ( 'NONE',  ( 1.000000000000000000, 0.000000000000000000, 0.000000000000000000 ) ) ;
#15435=EDGE_CURVE ( 'NONE', #15494, #23088, #10525, .T. ) ;
#15436=VERTEX_POINT ( 'NONE', #25739 ) ;
#15438=AXIS2_PLACEMENT_3D ( 'NONE', #1804, #14757, #12609 ) ;
#15440=CARTESIAN_POINT ( 'NONE',  ( 125.3433571860711453, 242.0587615242396566, -84.99999999999997158 ) ) ;
#15441=DIRECTION ( 'NONE',  ( 1.000000000000000000, 0.000000000000000000, 0.000000000000000000 ) ) ;
#15442=CARTESIAN_POINT ( 'NONE',  ( -63.57415822541634043, 75.97823757117562593, 80.00000000000001421 ) ) ;
#15444=CARTESIAN_POINT ( 'NONE',  ( -180.0000000000000284, -40.00000000000004974, 98.28427124746191623 ) ) ;
#15445=CARTESIAN_POINT ( 'NONE',  ( -210.0000000000000853, 59.99999999999993605, -18.66499754458839178 ) ) ;
#15448=CYLINDRICAL_SURFACE ( 'NONE', #10383, 9.999999999999982236 ) ;
#15449=CARTESIAN_POINT ( 'NONE',  ( 51.56615429303207065, 203.2034914284457159, -15.00000000000000000 ) ) ;
#15450=DIRECTION ( 'NONE',  ( -0.000000000000000000, -1.000000000000000000, -0.000000000000000000 ) ) ;
#15451=DIRECTION ( 'NONE',  ( 0.000000000000000000, 0.000000000000000000, -1.000000000000000000 ) ) ;
#15456=CARTESIAN_POINT ( 'NONE',  ( -236.3091765109048481, 68.24607436519741555, -5.736201002603987575 ) ) ;
#15458=ORIENTED_EDGE ( 'NONE', *, *, #5945, .T. ) ;
#15465=CARTESIAN_POINT ( 'NONE',  ( -212.6581729763558712, 72.57237399018264057, 29.67346677899678298 ) ) ;
#15474=ORIENTED_EDGE ( 'NONE', *, *, #25716, .F. ) ;
#15476=CARTESIAN_POINT ( 'NONE',  ( 98.38712641049259844, 233.7235291372264214, 21.27834768224934692 ) ) ;
#15479=LINE ( 'NONE', #6273, #25657 ) ;
#15483=DIRECTION ( 'NONE',  ( 1.000000000000000000, 0.000000000000000000, 0.000000000000000000 ) ) ;
#15492=CARTESIAN_POINT ( 'NONE',  ( 0.000000000000000000, 330.0000000000000000, -84.99999999999997158 ) ) ;
#15494=VERTEX_POINT ( 'NONE', #18858 ) ;
#15497=FACE_OUTER_BOUND ( 'NONE', #11700, .T. ) ;
#15499=CARTESIAN_POINT ( 'NONE',  ( -210.0000000000000000, -120.0000000000000711, -100.0000000000000142 ) ) ;
#15500=ORIENTED_EDGE ( 'NONE', *, *, #17034, .F. ) ;
#15501=AXIS2_PLACEMENT_3D ( 'NONE', #17078, #28266, #25838 ) ;
#15505=ORIENTED_EDGE ( 'NONE', *, *, #27119, .T. ) ;
#15512=CARTESIAN_POINT ( 'NONE',  ( -210.9349024751243178, 73.41979635535319915, 32.58420779144454826 ) ) ;
#15514=CIRCLE ( 'NONE', #22846, 9.999999999999996447 ) ;
#15516=DIRECTION ( 'NONE',  ( 1.000000000000000000, 0.000000000000000000, 0.000000000000000000 ) ) ;
#15518=DIRECTION ( 'NONE',  ( -0.000000000000000000, -0.000000000000000000, -1.000000000000000000 ) ) ;
#15519=DIRECTION ( 'NONE',  ( -0.000000000000000000, -0.000000000000000000, 1.000000000000000000 ) ) ;
#15520=ADVANCED_FACE ( 'NONE', ( #15410, #24166, #15126 ), #24299, .T. ) ;
#15522=CARTESIAN_POINT ( 'NONE',  ( -28.14180936505419695, 127.9576626828097545, 17.52305135179860685 ) ) ;
#15524=DIRECTION ( 'NONE',  ( 1.000000000000000000, 0.000000000000000000, 0.000000000000000000 ) ) ;
#15525=CARTESIAN_POINT ( 'NONE',  ( 33.10302365956999182, 219.6666220619077876, 12.99999999999999822 ) ) ;
#15527=VERTEX_POINT ( 'NONE', #21576 ) ;
#15528=DIRECTION ( 'NONE',  ( 0.000000000000000000, 0.000000000000000000, -1.000000000000000000 ) ) ;
#15530=DIRECTION ( 'NONE',  ( 0.000000000000000000, 0.000000000000000000, -1.000000000000000000 ) ) ;
#15531=VERTEX_POINT ( 'NONE', #4043 ) ;
#15533=ORIENTED_EDGE ( 'NONE', *, *, #17413, .F. ) ;
#15536=CARTESIAN_POINT ( 'NONE',  ( -151.6073178449016154, 124.1689584723159072, 19.47232524047854341 ) ) ;
#15540=ADVANCED_FACE ( 'NONE', ( #4463 ), #28333, .F. ) ;
#15543=CARTESIAN_POINT ( 'NONE',  ( -221.2146732495352239, 88.15369072822400653, 15.78728978121136883 ) ) ;
#15547=AXIS2_PLACEMENT_3D ( 'NONE', #11128, #9408, #15882 ) ;
#15550=CIRCLE ( 'NONE', #1305, 10.00000000000000888 ) ;
#15551=LINE ( 'NONE', #9221, #11965 ) ;
#15554=ORIENTED_EDGE ( 'NONE', *, *, #27528, .T. ) ;
#15559=CARTESIAN_POINT ( 'NONE',  ( -141.7923270636435404, 70.43557993099105374, 82.87231033183468298 ) ) ;
#15560=EDGE_LOOP ( 'NONE', ( #12745, #1624, #20922, #7127 ) ) ;
#15564=CIRCLE ( 'NONE', #428, 17.46154499483315448 ) ;
#15573=ORIENTED_EDGE ( 'NONE', *, *, #206, .T. ) ;
#15574=CARTESIAN_POINT ( 'NONE',  ( -17.91222884894589029, 128.7240434152827788, 17.19583536164714488 ) ) ;
#15581=EDGE_LOOP ( 'NONE', ( #861, #1930, #24612, #21193 ) ) ;
#15585=ADVANCED_FACE ( 'NONE', ( #6206 ), #28025, .F. ) ;
#15604=CARTESIAN_POINT ( 'NONE',  ( -208.5121489769019547, 74.88284981659903394, 38.34302025979879858 ) ) ;
#15607=ORIENTED_EDGE ( 'NONE', *, *, #18568, .F. ) ;
#15608=ORIENTED_EDGE ( 'NONE', *, *, #10522, .F. ) ;
#15611=CIRCLE ( 'NONE', #22028, 1.999999999999994893 ) ;
#15614=CARTESIAN_POINT ( 'NONE',  ( -223.0228900756071653, 134.9178336739567499, 12.97939780113086705 ) ) ;
#15615=CARTESIAN_POINT ( 'NONE',  ( 94.04374108504261187, 240.3974664687521567, 8.346404539543760492 ) ) ;
#15617=CARTESIAN_POINT ( 'NONE',  ( -254.3350114625770289, -91.18033988749901653, 16.36034929305424512 ) ) ;
#15618=DIRECTION ( 'NONE',  ( 0.000000000000000000, 0.000000000000000000, -1.000000000000000000 ) ) ;
#15619=EDGE_CURVE ( 'NONE', #2501, #11684, #23917, .T. ) ;
#15620=DIRECTION ( 'NONE',  ( 1.000000000000000000, 0.000000000000000000, 0.000000000000000000 ) ) ;
#15623=FACE_OUTER_BOUND ( 'NONE', #22697, .T. ) ;
#15625=CARTESIAN_POINT ( 'NONE',  ( 79.99999999999994316, -70.00000000000002842, 25.00000000000000000 ) ) ;
#15627=FACE_OUTER_BOUND ( 'NONE', #7429, .T. ) ;
#15632=AXIS2_PLACEMENT_3D ( 'NONE', #9681, #2924, #7532 ) ;
#15636=DIRECTION ( 'NONE',  ( 1.000000000000000000, 1.764238432794959761E-15, 0.000000000000000000 ) ) ;
#15639=CARTESIAN_POINT ( 'NONE',  ( 107.7348956500412385, 246.7603209947076834, -33.46154240484388964 ) ) ;
#15640=VERTEX_POINT ( 'NONE', #7355 ) ;
#15641=CARTESIAN_POINT ( 'NONE',  ( 4.489296788125576754, 138.9197681802679369, -13.09539705602191972 ) ) ;
#15645=VERTEX_POINT ( 'NONE', #15845 ) ;
#15651=DIRECTION ( 'NONE',  ( 0.000000000000000000, 0.000000000000000000, 1.000000000000000000 ) ) ;
#15655=CARTESIAN_POINT ( 'NONE',  ( -214.3579997887104298, 72.01340221155322752, 27.44224251620622113 ) ) ;
#15660=DIRECTION ( 'NONE',  ( 1.541976423090495387E-16, -1.000000000000000000, 0.000000000000000000 ) ) ;
#15663=CARTESIAN_POINT ( 'NONE',  ( -5.301150576437182238, 133.7253806968913636, 14.04417438168983345 ) ) ;
#15664=DIRECTION ( 'NONE',  ( 1.000000000000000000, 0.000000000000000000, 0.000000000000000000 ) ) ;
#15673=CARTESIAN_POINT ( 'NONE',  ( -207.2829329158516316, 90.24556741685469774, -26.81980500862954031 ) ) ;
#15677=AXIS2_PLACEMENT_3D ( 'NONE', #3026, #14107, #22857 ) ;
#15678=DIRECTION ( 'NONE',  ( -0.000000000000000000, -0.000000000000000000, -1.000000000000000000 ) ) ;
#15679=CARTESIAN_POINT ( 'NONE',  ( -158.6464230094932191, 121.2366000616820116, 20.46992577562846094 ) ) ;
#15682=ADVANCED_FACE ( 'NONE', ( #24873 ), #16123, .T. ) ;
#15683=FACE_OUTER_BOUND ( 'NONE', #20542, .T. ) ;
#15686=CARTESIAN_POINT ( 'NONE',  ( -205.2899939696512206, 91.43266760401971283, 27.40424638492752862 ) ) ;
#15692=CARTESIAN_POINT ( 'NONE',  ( -196.2821818994568162, 62.43869624199520985, -34.70549414534111321 ) ) ;
#15696=CARTESIAN_POINT ( 'NONE',  ( -226.9194714820147567, 131.5555516077983782, -12.99999999956374452 ) ) ;
#15701=EDGE_CURVE ( 'NONE', #12426, #17181, #6915, .T. ) ;
#15703=DIRECTION ( 'NONE',  ( -4.625929269271485914E-16, 1.000000000000000000, 0.000000000000000000 ) ) ;
#15704=CARTESIAN_POINT ( 'NONE',  ( -139.1329441303325325, 71.54464929955096864, 82.80879831960034210 ) ) ;
#15707=VERTEX_POINT ( 'NONE', #20554 ) ;
#15710=CARTESIAN_POINT ( 'NONE',  ( -199.1252820381085655, 96.45000389891778525, -30.47981965597484688 ) ) ;
#15711=ORIENTED_EDGE ( 'NONE', *, *, #27341, .F. ) ;
#15712=AXIS2_PLACEMENT_3D ( 'NONE', #98, #385, #7279 ) ;
#15717=LINE ( 'NONE', #28326, #19833 ) ;
#15720=EDGE_CURVE ( 'NONE', #4224, #16662, #12353, .T. ) ;
#15721=CARTESIAN_POINT ( 'NONE',  ( -11.21207136966835449, 130.1511864905693017, 16.65378689143514634 ) ) ;
#15726=CARTESIAN_POINT ( 'NONE',  ( -20.10010832150799587, 128.4146997938364052, -17.32638360930989663 ) ) ;
#15729=CARTESIAN_POINT ( 'NONE',  ( -209.5848674449188422, 66.48010988065568938, -33.34549737723507690 ) ) ;
#15732=AXIS2_PLACEMENT_3D ( 'NONE', #6954, #20029, #6811 ) ;
#15735=CIRCLE ( 'NONE', #24912, 5.999999999999991118 ) ;
#15737=CARTESIAN_POINT ( 'NONE',  ( 109.9999999999999432, 110.0000000000000142, 70.00000000000001421 ) ) ;
#15739=DIRECTION ( 'NONE',  ( 1.000000000000000000, 0.000000000000000000, 0.000000000000000000 ) ) ;
#15740=AXIS2_PLACEMENT_3D ( 'NONE', #26861, #11360, #16102 ) ;
#15743=CARTESIAN_POINT ( 'NONE',  ( -233.4149848405407965, 66.33036726544322903, -6.308275885109299708 ) ) ;
#15745=ORIENTED_EDGE ( 'NONE', *, *, #3191, .F. ) ;
#15750=CARTESIAN_POINT ( 'NONE',  ( 134.9999999999998579, 220.0000000000000284, 90.00000000000002842 ) ) ;
#15751=EDGE_LOOP ( 'NONE', ( #1588, #5823, #5137, #13070 ) ) ;
#15763=CARTESIAN_POINT ( 'NONE',  ( 105.7038310726827888, 247.5990904218997173, 23.20200675067667362 ) ) ;
#15764=VECTOR ( 'NONE', #401, 1000.000000000000000 ) ;
#15768=FACE_OUTER_BOUND ( 'NONE', #5773, .T. ) ;
#15770=CARTESIAN_POINT ( 'NONE',  ( -63.57415822541634043, 75.97823757117562593, 100.0000000000000000 ) ) ;
#15771=CARTESIAN_POINT ( 'NONE',  ( -207.5044420441007276, 75.59897387903043864, -45.00000000000000000 ) ) ;
#15773=DIRECTION ( 'NONE',  ( 0.000000000000000000, 0.000000000000000000, 1.000000000000000000 ) ) ;
#15779=CIRCLE ( 'NONE', #3366, 30.00000000000000000 ) ;
#15780=EDGE_CURVE ( 'NONE', #19657, #15896, #22581, .T. ) ;
#15782=CARTESIAN_POINT ( 'NONE',  ( -2.081668171172168513E-14, 79.99999999999998579, 70.00000000000001421 ) ) ;
#15783=FACE_OUTER_BOUND ( 'NONE', #10965, .T. ) ;
#15785=VERTEX_POINT ( 'NONE', #7771 ) ;
#15786=CARTESIAN_POINT ( 'NONE',  ( 109.9760533923165156, 258.8696700914497342, -43.04221176959693196 ) ) ;
#15792=ORIENTED_EDGE ( 'NONE', *, *, #22889, .F. ) ;
#15793=EDGE_CURVE ( 'NONE', #18588, #18153, #19105, .T. ) ;
#15795=CARTESIAN_POINT ( 'NONE',  ( -47.46824071874176099, 132.2249976274591177, 14.48593008886889244 ) ) ;
#15801=CARTESIAN_POINT ( 'NONE',  ( 79.99999999999990052, 230.0000000000000284, -45.00000000000000000 ) ) ;
#15803=UNCERTAINTY_MEASURE_WITH_UNIT (LENGTH_MEASURE( 1.000000000000000082E-05 ), #5516, 'distance_accuracy_value', 'NONE');
#15805=CARTESIAN_POINT ( 'NONE',  ( -217.4092282431682577, 59.59925738963178077, 26.62835594396387506 ) ) ;
#15807=CARTESIAN_POINT ( 'NONE',  ( 134.9999999999998579, 220.0000000000000284, 90.00000000000002842 ) ) ;
#15811=B_SPLINE_CURVE_WITH_KNOTS ( 'NONE', 3,
 ( #14815, #25711, #6036, #1162, #23567, #14252, #16542, #3878 ),
 .UNSPECIFIED., .F., .F.,
 ( 4, 2, 2, 4 ),
 ( 0.03156115556267154870, 0.03330631506936942987, 0.03505147457606731104, 0.03854179358946310113 ),
 .UNSPECIFIED. ) ;
#15812=CARTESIAN_POINT ( 'NONE',  ( 90.17595424772805757, 111.7661400908348384, 72.22656249985354293 ) ) ;
#15813=LINE ( 'NONE', #4865, #16468 ) ;
#15814=FACE_OUTER_BOUND ( 'NONE', #6086, .T. ) ;
#15817=EDGE_LOOP ( 'NONE', ( #9566, #10868, #827, #23146 ) ) ;
#15819=AXIS2_PLACEMENT_3D ( 'NONE', #22750, #14412, #7528 ) ;
#15820=CARTESIAN_POINT ( 'NONE',  ( -208.7912193213397245, 88.73557081762633914, -26.19220075538009240 ) ) ;
#15821=DIRECTION ( 'NONE',  ( -0.000000000000000000, -1.000000000000000000, -0.000000000000000000 ) ) ;
#15822=CARTESIAN_POINT ( 'NONE',  ( -209.0043318837038555, 89.43882380443007207, -25.53063627850903217 ) ) ;
#15829=CARTESIAN_POINT ( 'NONE',  ( -127.4298061085324889, 130.3533807148441213, 16.56307014168300995 ) ) ;
#15830=VERTEX_POINT ( 'NONE', #10069 ) ;
#15832=DIRECTION ( 'NONE',  ( -3.469446951953614189E-16, 1.000000000000000000, 0.000000000000000000 ) ) ;
#15837=AXIS2_PLACEMENT_3D ( 'NONE', #24406, #17367, #11347 ) ;
#15838=CARTESIAN_POINT ( 'NONE',  ( 105.5625601981895585, 242.0882937662017014, -29.27845391395231545 ) ) ;
#15839=EDGE_CURVE ( 'NONE', #13234, #24608, #23279, .T. ) ;
#15842=DIRECTION ( 'NONE',  ( 1.000000000000000000, 0.000000000000000000, 0.000000000000000000 ) ) ;
#15843=CARTESIAN_POINT ( 'NONE',  ( -195.1986077931981356, 62.83738171803135231, -37.97438512083786577 ) ) ;
#15845=CARTESIAN_POINT ( 'NONE',  ( -12.24491960465745599, -18.01420295945611727, 80.00000000000001421 ) ) ;
#15846=CARTESIAN_POINT ( 'NONE',  ( -219.9212092885467484, 137.1730549828544667, -15.11921763784017436 ) ) ;
#15848=DIRECTION ( 'NONE',  ( 0.000000000000000000, 0.000000000000000000, 1.000000000000000000 ) ) ;
#15849=ORIENTED_EDGE ( 'NONE', *, *, #24397, .F. ) ;
#15850=DIRECTION ( 'NONE',  ( -0.000000000000000000, -0.000000000000000000, 1.000000000000000000 ) ) ;
#15851=CARTESIAN_POINT ( 'NONE',  ( 79.99999999999991473, 139.9999999999999716, -45.00000000000000000 ) ) ;
#15852=DIRECTION ( 'NONE',  ( 0.000000000000000000, 0.000000000000000000, -1.000000000000000000 ) ) ;
#15858=CARTESIAN_POINT ( 'NONE',  ( 94.38583646782731762, 113.6320904521816857, 75.15625000028097702 ) ) ;
#15859=CARTESIAN_POINT ( 'NONE',  ( -201.5824907507999342, 94.41641349969115993, -29.50224322716549707 ) ) ;
#15862=ORIENTED_EDGE ( 'NONE', *, *, #2804, .F. ) ;
#15865=ORIENTED_EDGE ( 'NONE', *, *, #15371, .F. ) ;
#15866=CARTESIAN_POINT ( 'NONE',  ( 91.70829090827390928, 81.72138244997330503, 100.0000000000000142 ) ) ;
#15868=FACE_BOUND ( 'NONE', #17120, .T. ) ;
#15870=EDGE_CURVE ( 'NONE', #19273, #17375, #21950, .T. ) ;
#15873=CARTESIAN_POINT ( 'NONE',  ( -17.81748447342208053, 128.7387662681335883, -17.18977265686632094 ) ) ;
#15875=AXIS2_PLACEMENT_3D ( 'NONE', #10084, #18836, #5764 ) ;
#15880=CIRCLE ( 'NONE', #3464, 9.999999999999998224 ) ;
#15882=DIRECTION ( 'NONE',  ( -0.5975062131282562472, 0.8018642810807392607, 0.000000000000000000 ) ) ;
#15885=EDGE_CURVE ( 'NONE', #9167, #25901, #10777, .T. ) ;
#15887=EDGE_LOOP ( 'NONE', ( #11823, #16586, #6514 ) ) ;
#15890=CARTESIAN_POINT ( 'NONE',  ( -248.1546605714623013, -91.18033988749901653, 0.000000000000000000 ) ) ;
#15891=CARTESIAN_POINT ( 'NONE',  ( -189.5231184314577320, 157.6231267382823376, -13.00000000000000000 ) ) ;
#15894=ORIENTED_EDGE ( 'NONE', *, *, #16693, .F. ) ;
#15896=VERTEX_POINT ( 'NONE', #15382 ) ;
#15898=EDGE_LOOP ( 'NONE', ( #19962, #5126, #9413, #5019 ) ) ;
#15899=AXIS2_PLACEMENT_3D ( 'NONE', #11345, #20090, #22394 ) ;
#15908=CARTESIAN_POINT ( 'NONE',  ( 98.38958437018622760, 241.8303606468397220, 11.96405203492901137 ) ) ;
#15909=CARTESIAN_POINT ( 'NONE',  ( -217.7401460507884110, 138.5677444271666161, 12.99353264133693742 ) ) ;
#15911=CARTESIAN_POINT ( 'NONE',  ( 79.99999999999992895, 110.0000000000000000, -70.00000000000001421 ) ) ;
#15914=PLANE ( 'NONE',  #8568 ) ;
#15916=DIRECTION ( 'NONE',  ( 1.000000000000000000, 0.000000000000000000, 0.000000000000000000 ) ) ;
#15919=TOROIDAL_SURFACE ( 'NONE', #3503, 55.86582179324592090, 2.000000000000000000 ) ;
#15920=EDGE_LOOP ( 'NONE', ( #21694, #18504, #26422, #6551 ) ) ;
#15929=ORIENTED_EDGE ( 'NONE', *, *, #22171, .F. ) ;
#15932=ORIENTED_EDGE ( 'NONE', *, *, #9877, .F. ) ;
#15937=DIRECTION ( 'NONE',  ( 0.000000000000000000, 0.000000000000000000, -1.000000000000000000 ) ) ;
#15938=CARTESIAN_POINT ( 'NONE',  ( 109.9999999999999574, -120.0000000000000426, 70.00000000000001421 ) ) ;
#15941=CARTESIAN_POINT ( 'NONE',  ( -224.2911920753103345, 72.03214051460449241, 18.76861173149748652 ) ) ;
#15945=CARTESIAN_POINT ( 'NONE',  ( 79.99999999999995737, 98.29969375664606446, -93.85322876744665166 ) ) ;
#15946=CARTESIAN_POINT ( 'NONE',  ( -210.6525827442121113, 88.81591185141229516, -22.91848360207728419 ) ) ;
#15948=CARTESIAN_POINT ( 'NONE',  ( 85.90765579575223398, 110.5723347142863702, 70.58593750014345858 ) ) ;
#15949=CARTESIAN_POINT ( 'NONE',  ( -11.46153413423660794, 131.5065341654955091, 16.18491763777246462 ) ) ;
#15951=CARTESIAN_POINT ( 'NONE',  ( -178.7338692018542474, 110.4480143559095069, 30.37507499509654352 ) ) ;
#15952=ADVANCED_FACE ( 'NONE', ( #8621 ), #17371, .F. ) ;
#15957=DIRECTION ( 'NONE',  ( 1.000000000000000000, -0.000000000000000000, -0.000000000000000000 ) ) ;
#15958=ADVANCED_FACE ( 'NONE', ( #13086 ), #7173, .T. ) ;
#15965=EDGE_LOOP ( 'NONE', ( #20608, #11299, #19616, #3534 ) ) ;
#15967=CARTESIAN_POINT ( 'NONE',  ( -151.1419734269974242, 123.3149796224834063, 20.04527379734153314 ) ) ;
#15968=VERTEX_POINT ( 'NONE', #17948 ) ;
#15974=ORIENTED_EDGE ( 'NONE', *, *, #19922, .F. ) ;
#15975=DIRECTION ( 'NONE',  ( 1.000000000000000000, 0.000000000000000000, 0.000000000000000000 ) ) ;
#15978=TOROIDAL_SURFACE ( 'NONE', #7251, 21.49999999999998224, 1.000000000000000000 ) ;
#15980=LINE ( 'NONE', #24871, #14585 ) ;
#15981=CARTESIAN_POINT ( 'NONE',  ( -213.3516035875686896, 56.48049070729078380, -40.70111258791201436 ) ) ;
#15982=EDGE_CURVE ( 'NONE', #2906, #24382, #15813, .T. ) ;
#15983=EDGE_CURVE ( 'NONE', #24382, #26112, #22402, .T. ) ;
#15991=ADVANCED_FACE ( 'NONE', ( #20242 ), #22427, .F. ) ;
#15992=DIRECTION ( 'NONE',  ( 1.000000000000000000, 0.000000000000000000, 0.000000000000000000 ) ) ;
#15993=AXIS2_PLACEMENT_3D ( 'NONE', #21724, #6767, #13254 ) ;
#16003=CIRCLE ( 'NONE', #3582, 16.46313063346208239 ) ;
#16008=AXIS2_PLACEMENT_3D ( 'NONE', #24808, #9152, #17910 ) ;
#16009=AXIS2_PLACEMENT_3D ( 'NONE', #7732, #3124, #25531 ) ;
#16012=CARTESIAN_POINT ( 'NONE',  ( 9.345921402568846403, 139.9999999999999716, -15.00000000000000000 ) ) ;
#16017=ORIENTED_EDGE ( 'NONE', *, *, #17067, .F. ) ;
#16022=ORIENTED_EDGE ( 'NONE', *, *, #2989, .T. ) ;
#16023=CARTESIAN_POINT ( 'NONE',  ( 123.9999999999998579, 220.0000000000000284, 99.00000000000001421 ) ) ;
#16028=CARTESIAN_POINT ( 'NONE',  ( 9.999999999999957367, -20.00000000000004974, 100.0000000000000142 ) ) ;
#16030=DIRECTION ( 'NONE',  ( 0.000000000000000000, 0.000000000000000000, 1.000000000000000000 ) ) ;
#16033=DIRECTION ( 'NONE',  ( 0.000000000000000000, 0.000000000000000000, 1.000000000000000000 ) ) ;
#16034=ORIENTED_EDGE ( 'NONE', *, *, #10567, .F. ) ;
#16044=CARTESIAN_POINT ( 'NONE',  ( 107.0062495987318272, 249.1467455478686759, 31.68887795644912586 ) ) ;
#16045=EDGE_CURVE ( 'NONE', #6225, #10678, #3948, .T. ) ;
#16046=VECTOR ( 'NONE', #14855, 1000.000000000000000 ) ;
#16049=CARTESIAN_POINT ( 'NONE',  ( -223.3099978423094001, 137.4510275522738993, -14.96944044186858491 ) ) ;
#16051=CIRCLE ( 'NONE', #17401, 5.000000000000004441 ) ;
#16053=CARTESIAN_POINT ( 'NONE',  ( 93.99999999999985789, 171.5103103742661972, -84.99999999999997158 ) ) ;
#16054=CARTESIAN_POINT ( 'NONE',  ( -233.2943309833551950, 92.06151970357237246, -13.00000000000000000 ) ) ;
#16056=CARTESIAN_POINT ( 'NONE',  ( 144.9999999999998863, 220.0000000000000284, 90.00000000000002842 ) ) ;
#16061=AXIS2_PLACEMENT_3D ( 'NONE', #19237, #10622, #8037 ) ;
#16062=DIRECTION ( 'NONE',  ( 1.000000000000000000, 0.000000000000000000, 0.000000000000000000 ) ) ;
#16064=DIRECTION ( 'NONE',  ( -0.000000000000000000, -0.000000000000000000, -1.000000000000000000 ) ) ;
#16067=ADVANCED_FACE ( 'NONE', ( #27648 ), #12736, .T. ) ;
#16068=AXIS2_PLACEMENT_3D ( 'NONE', #26860, #15957, #24709 ) ;
#16073=ORIENTED_EDGE ( 'NONE', *, *, #549, .F. ) ;
#16075=ORIENTED_EDGE ( 'NONE', *, *, #21468, .F. ) ;
#16077=ORIENTED_EDGE ( 'NONE', *, *, #10519, .F. ) ;
#16082=CARTESIAN_POINT ( 'NONE',  ( -107.7681813716040580, 133.6595412580404059, -15.67431181523478578 ) ) ;
#16084=DIRECTION ( 'NONE',  ( -0.000000000000000000, 1.000000000000000000, -1.387778780781445429E-16 ) ) ;
#16086=CARTESIAN_POINT ( 'NONE',  ( -213.7039558558103352, 55.82027786946292025, 42.47917487896670963 ) ) ;
#16090=CARTESIAN_POINT ( 'NONE',  ( 79.99999999999995737, 106.0349479707060993, -85.03452022453005554 ) ) ;
#16091=CARTESIAN_POINT ( 'NONE',  ( -204.2442923823817011, 92.17690269152525673, -28.15093001741121981 ) ) ;
#16097=CARTESIAN_POINT ( 'NONE',  ( 91.70829090828171104, 81.72138244998292578, -100.0000000000000284 ) ) ;
#16101=CARTESIAN_POINT ( 'NONE',  ( -203.8025521703607694, 92.07732029363670279, -29.54281560658175465 ) ) ;
#16102=DIRECTION ( 'NONE',  ( 1.000000000000000000, 0.000000000000000000, 0.000000000000000000 ) ) ;
#16105=EDGE_LOOP ( 'NONE', ( #17024, #24465, #19089, #25338 ) ) ;
#16106=DIRECTION ( 'NONE',  ( -1.000000000000000000, -3.469446951953614189E-16, 0.000000000000000000 ) ) ;
#16108=CARTESIAN_POINT ( 'NONE',  ( -127.8937336576301220, 131.6565518472861243, 14.66727481766007202 ) ) ;
#16110=EDGE_LOOP ( 'NONE', ( #22746, #13072, #26449 ) ) ;
#16115=CARTESIAN_POINT ( 'NONE',  ( -203.1779787704217028, 93.05164332230201296, 28.77272332722131054 ) ) ;
#16118=EDGE_CURVE ( 'NONE', #17857, #27076, #25167, .T. ) ;
#16121=CARTESIAN_POINT ( 'NONE',  ( -207.6173544636101553, 75.51556044650348554, -42.73482814336003344 ) ) ;
#16123=CYLINDRICAL_SURFACE ( 'NONE', #28366, 10.00000000000000888 ) ;
#16124=FACE_OUTER_BOUND ( 'NONE', #16864, .T. ) ;
#16130=CARTESIAN_POINT ( 'NONE',  ( -236.8177751472017007, 82.33896643611701904, 15.00000000000000000 ) ) ;
#16134=CARTESIAN_POINT ( 'NONE',  ( 107.3061218088239883, 127.3934823310315920, 99.99999999997838529 ) ) ;
#16136=EDGE_LOOP ( 'NONE', ( #18953, #623, #3932, #22042 ) ) ;
#16137=EDGE_LOOP ( 'NONE', ( #766, #4978, #9346, #5865 ) ) ;
#16138=CARTESIAN_POINT ( 'NONE',  ( -180.0000000000000284, -50.00000000000004263, 80.00000000000001421 ) ) ;
#16139=CIRCLE ( 'NONE', #3723, 1.000000000000000888 ) ;
#16152=CARTESIAN_POINT ( 'NONE',  ( -6.744242412876251258, 131.5654230417238466, -16.20713396055394995 ) ) ;
#16153=CARTESIAN_POINT ( 'NONE',  ( 65.00000000000000000, -120.0250000000000909, -76.00000000000000000 ) ) ;
#16158=CARTESIAN_POINT ( 'NONE',  ( -237.3870311360069536, 121.7710280244218950, 15.00000000000000000 ) ) ;
#16160=DIRECTION ( 'NONE',  ( 0.000000000000000000, -0.000000000000000000, -1.000000000000000000 ) ) ;
#16162=DIRECTION ( 'NONE',  ( -0.8314772792026905446, 0.5555587585212667934, 0.000000000000000000 ) ) ;
#16163=ORIENTED_EDGE ( 'NONE', *, *, #17685, .F. ) ;
#16166=CARTESIAN_POINT ( 'NONE',  ( -215.7935364303660322, 60.28281843632714754, -13.31033261678753910 ) ) ;
#16171=AXIS2_PLACEMENT_3D ( 'NONE', #25483, #23610, #5940 ) ;
#16174=AXIS2_PLACEMENT_3D ( 'NONE', #2941, #7112, #25066 ) ;
#16192=AXIS2_PLACEMENT_3D ( 'NONE', #9973, #23747, #25610 ) ;
#16193=DIRECTION ( 'NONE',  ( -0.000000000000000000, -0.000000000000000000, -1.000000000000000000 ) ) ;
#16200=LINE ( 'NONE', #20350, #12338 ) ;
#16204=CARTESIAN_POINT ( 'NONE',  ( -180.0000000000000284, -40.00000000000004974, 110.0000000000000284 ) ) ;
#16222=CARTESIAN_POINT ( 'NONE',  ( -82.58612381453100681, 136.4858469420659333, -13.47871251474561305 ) ) ;
#16223=DIRECTION ( 'NONE',  ( 0.000000000000000000, 0.000000000000000000, -1.000000000000000000 ) ) ;
#16225=CARTESIAN_POINT ( 'NONE',  ( -210.0090741174316804, 73.93180346605655018, 34.41452853221989727 ) ) ;
#16230=CARTESIAN_POINT ( 'NONE',  ( 79.99999999999997158, 89.66646975086555926, -98.46778313769407021 ) ) ;
#16231=DIRECTION ( 'NONE',  ( 0.000000000000000000, 0.000000000000000000, 1.000000000000000000 ) ) ;
#16232=CIRCLE ( 'NONE', #21707, 20.00000000000001776 ) ;
#16234=FACE_OUTER_BOUND ( 'NONE', #27350, .T. ) ;
#16238=CARTESIAN_POINT ( 'NONE',  ( -40.40953891503691153, 0.000000000000000000, 100.0000000000000000 ) ) ;
#16239=ORIENTED_EDGE ( 'NONE', *, *, #16462, .T. ) ;
#16247=CIRCLE ( 'NONE', #22663, 64.76834224489934400 ) ;
#16249=CARTESIAN_POINT ( 'NONE',  ( -81.44467526201103169, 136.3898447976469868, 13.49545388103471311 ) ) ;
#16253=ORIENTED_EDGE ( 'NONE', *, *, #25377, .T. ) ;
#16254=CARTESIAN_POINT ( 'NONE',  ( 139.9999999999999716, -120.0000000000000568, -100.0000000000000142 ) ) ;
#16256=CARTESIAN_POINT ( 'NONE',  ( -71.37541315349507443, 230.0000000000000000, -5.000000000000002665 ) ) ;
#16257=CARTESIAN_POINT ( 'NONE',  ( 99.01629842454553909, 234.2218078846129856, -21.79257675089547064 ) ) ;
#16259=DIRECTION ( 'NONE',  ( -1.000000000000000000, -8.673617379884036705E-17, -0.000000000000000000 ) ) ;
#16260=CARTESIAN_POINT ( 'NONE',  ( -206.2579005266799186, 60.21847207785817346, -20.52143262683453528 ) ) ;
#16263=DIRECTION ( 'NONE',  ( -1.000000000000000000, -0.000000000000000000, -0.000000000000000000 ) ) ;
#16264=CARTESIAN_POINT ( 'NONE',  ( 134.9999999999998579, 220.0000000000000284, -105.0000000000000284 ) ) ;
#16265=CIRCLE ( 'NONE', #3857, 5.000000000000004441 ) ;
#16267=ORIENTED_EDGE ( 'NONE', *, *, #26865, .T. ) ;
#16268=CARTESIAN_POINT ( 'NONE',  ( -279.3160071107327553, -91.18033988749901653, 14.13483123440684253 ) ) ;
#16269=CARTESIAN_POINT ( 'NONE',  ( -233.3699482038331610, 66.30323757540675444, 6.318463073150136999 ) ) ;
#16270=DIRECTION ( 'NONE',  ( 0.000000000000000000, 0.000000000000000000, 1.000000000000000000 ) ) ;
#16271=ORIENTED_EDGE ( 'NONE', *, *, #7015, .T. ) ;
#16273=EDGE_CURVE ( 'NONE', #15896, #26994, #5907, .T. ) ;
#16275=EDGE_CURVE ( 'NONE', #8411, #22091, #11929, .T. ) ;
#16279=ORIENTED_EDGE ( 'NONE', *, *, #18408, .F. ) ;
#16281=ORIENTED_EDGE ( 'NONE', *, *, #11591, .F. ) ;
#16282=FACE_OUTER_BOUND ( 'NONE', #4694, .T. ) ;
#16284=LINE ( 'NONE', #25450, #8201 ) ;
#16285=ORIENTED_EDGE ( 'NONE', *, *, #11995, .F. ) ;
#16289=CARTESIAN_POINT ( 'NONE',  ( -115.3221550338875687, 66.54464929955099706, 83.00000000000001421 ) ) ;
#16292=CARTESIAN_POINT ( 'NONE',  ( -13.31932916636724151, 129.6218899819808144, -16.84828668634186499 ) ) ;
#16293=DIRECTION ( 'NONE',  ( -0.000000000000000000, 1.000000000000000000, -1.387778780781445429E-16 ) ) ;
#16302=ORIENTED_EDGE ( 'NONE', *, *, #9337, .T. ) ;
#16304=CARTESIAN_POINT ( 'NONE',  ( -238.3976651326582044, 69.81518760999661311, 5.405651710414779210 ) ) ;
#16307=CARTESIAN_POINT ( 'NONE',  ( -217.0264852877946566, -91.18033988749901653, 0.000000000000000000 ) ) ;
#16308=FACE_OUTER_BOUND ( 'NONE', #24508, .T. ) ;
#16312=AXIS2_PLACEMENT_3D ( 'NONE', #24206, #362, #6679 ) ;
#16314=EDGE_CURVE ( 'NONE', #25995, #19755, #23366, .T. ) ;
#16316=CYLINDRICAL_SURFACE ( 'NONE', #8337, 30.00000000000000000 ) ;
#16318=CARTESIAN_POINT ( 'NONE',  ( 104.1955293147850199, 245.8507536825374871, 19.98755400232634116 ) ) ;
#16319=EDGE_LOOP ( 'NONE', ( #3733, #10783 ) ) ;
#16322=ORIENTED_EDGE ( 'NONE', *, *, #18057, .T. ) ;
#16324=ORIENTED_EDGE ( 'NONE', *, *, #13256, .T. ) ;
#16327=AXIS2_PLACEMENT_3D ( 'NONE', #815, #2671, #18345 ) ;
#16331=CIRCLE ( 'NONE', #9905, 22.49999999999999289 ) ;
#16332=CARTESIAN_POINT ( 'NONE',  ( 109.9999999999999147, 140.0000000000000000, -90.00000000000004263 ) ) ;
#16335=DIRECTION ( 'NONE',  ( -0.000000000000000000, -0.000000000000000000, 1.000000000000000000 ) ) ;
#16339=ORIENTED_EDGE ( 'NONE', *, *, #9211, .T. ) ;
#16341=EDGE_CURVE ( 'NONE', #13033, #14756, #26106, .T. ) ;
#16343=DIRECTION ( 'NONE',  ( 1.000000000000000000, 0.000000000000000000, 0.000000000000000000 ) ) ;
#16346=CARTESIAN_POINT ( 'NONE',  ( -248.1546605714623013, -91.18033988749901653, 0.000000000000000000 ) ) ;
#16347=ORIENTED_EDGE ( 'NONE', *, *, #1879, .T. ) ;
#16351=EDGE_CURVE ( 'NONE', #10474, #12013, #3348, .T. ) ;
#16353=AXIS2_PLACEMENT_3D ( 'NONE', #22395, #13359, #10912 ) ;
#16358=CARTESIAN_POINT ( 'NONE',  ( -122.9450662303175363, 132.7613262207298703, 14.33664937305252707 ) ) ;
#16359=CARTESIAN_POINT ( 'NONE',  ( -17.24491960465745777, 0.000000000000000000, 95.00000000000000000 ) ) ;
#16360=CARTESIAN_POINT ( 'NONE',  ( 157.4999999999998579, 220.0000000000000284, -105.0000000000000284 ) ) ;
#16364=CARTESIAN_POINT ( 'NONE',  ( -207.8278798888169945, 75.36218601466582356, 41.22349376586717540 ) ) ;
#16368=CARTESIAN_POINT ( 'NONE',  ( -230.7999239170523538, 92.53513801463330424, -13.02866169270885344 ) ) ;
#16381=ORIENTED_EDGE ( 'NONE', *, *, #11115, .F. ) ;
#16385=EDGE_CURVE ( 'NONE', #5481, #10749, #1062, .T. ) ;
#16386=ADVANCED_FACE ( 'NONE', ( #12139 ), #18173, .T. ) ;
#16392=CARTESIAN_POINT ( 'NONE',  ( 95.14887760048110010, 231.7800724511707813, -19.10096717460264770 ) ) ;
#16394=DIRECTION ( 'NONE',  ( -0.000000000000000000, -0.000000000000000000, 1.000000000000000000 ) ) ;
#16399=CARTESIAN_POINT ( 'NONE',  ( -194.2478650485211062, 63.21120109188145619, -44.02102422013626892 ) ) ;
#16403=DIRECTION ( 'NONE',  ( -0.000000000000000000, -0.000000000000000000, 1.000000000000000000 ) ) ;
#16406=LINE ( 'NONE', #4762, #24770 ) ;
#16407=CARTESIAN_POINT ( 'NONE',  ( -235.5446291276685713, 67.70753763449820894, 5.872244511703956782 ) ) ;
#16409=ORIENTED_EDGE ( 'NONE', *, *, #13635, .T. ) ;
#16412=CIRCLE ( 'NONE', #4069, 30.00000000000000000 ) ;
#16413=EDGE_CURVE ( 'NONE', #7931, #23684, #501, .T. ) ;
#16417=AXIS2_PLACEMENT_3D ( 'NONE', #7161, #24685, #13785 ) ;
#16420=DIRECTION ( 'NONE',  ( 0.000000000000000000, 0.000000000000000000, 1.000000000000000000 ) ) ;
#16423=CARTESIAN_POINT ( 'NONE',  ( 82.91040908012763566, 80.00000000660637056, 100.0000000000000142 ) ) ;
#16429=LINE ( 'NONE', #5497, #26093 ) ;
#16435=VERTEX_POINT ( 'NONE', #19288 ) ;
#16437=EDGE_CURVE ( 'NONE', #18588, #10524, #1619, .T. ) ;
#16441=DIRECTION ( 'NONE',  ( 0.000000000000000000, 0.000000000000000000, -1.000000000000000000 ) ) ;
#16442=ORIENTED_EDGE ( 'NONE', *, *, #13381, .T. ) ;
#16453=VERTEX_POINT ( 'NONE', #14426 ) ;
#16456=VECTOR ( 'NONE', #26956, 1000.000000000000000 ) ;
#16459=ORIENTED_EDGE ( 'NONE', *, *, #20062, .T. ) ;
#16461=CARTESIAN_POINT ( 'NONE',  ( -216.6285223362424404, 139.2238150404710666, 13.00000000000000178 ) ) ;
#16462=EDGE_CURVE ( 'NONE', #12635, #9863, #2635, .T. ) ;
#16464=EDGE_CURVE ( 'NONE', #4054, #8160, #5654, .T. ) ;
#16465=CARTESIAN_POINT ( 'NONE',  ( 87.74278500246884960, 111.0010834413659921, -71.13281249983540988 ) ) ;
#16468=VECTOR ( 'NONE', #13654, 1000.000000000000000 ) ;
#16471=CARTESIAN_POINT ( 'NONE',  ( 113.4999999999998863, 220.0000000000000284, 100.0000000000000142 ) ) ;
#16474=EDGE_LOOP ( 'NONE', ( #6441, #9806 ) ) ;
#16475=CARTESIAN_POINT ( 'NONE',  ( -8.960146631618641777, 132.3429123680572275, 14.45742179905339952 ) ) ;
#16478=CARTESIAN_POINT ( 'NONE',  ( 104.1954684636752972, 245.8506931952819627, -19.98744076451168183 ) ) ;
#16482=AXIS2_PLACEMENT_3D ( 'NONE', #25871, #4173, #23722 ) ;
#16484=EDGE_LOOP ( 'NONE', ( #661, #23885, #22275, #18172 ) ) ;
#16486=ORIENTED_EDGE ( 'NONE', *, *, #11480, .T. ) ;
#16488=AXIS2_PLACEMENT_3D ( 'NONE', #2784, #647, #16162 ) ;
#16489=ORIENTED_EDGE ( 'NONE', *, *, #3145, .F. ) ;
#16492=ORIENTED_EDGE ( 'NONE', *, *, #5750, .F. ) ;
#16493=CARTESIAN_POINT ( 'NONE',  ( 114.6895484223571771, 229.7318084278312540, 98.48649515991442627 ) ) ;
#16498=CARTESIAN_POINT ( 'NONE',  ( -92.74993325912653575, 136.3626345347758502, -13.50003192765508508 ) ) ;
#16504=EDGE_CURVE ( 'NONE', #5960, #230, #15564, .T. ) ;
#16511=CARTESIAN_POINT ( 'NONE',  ( -241.9743096803475453, -91.18033988749901653, 17.46154499483315448 ) ) ;
#16514=ORIENTED_EDGE ( 'NONE', *, *, #24444, .T. ) ;
#16515=ORIENTED_EDGE ( 'NONE', *, *, #2899, .T. ) ;
#16522=ORIENTED_EDGE ( 'NONE', *, *, #26341, .T. ) ;
#16529=DIRECTION ( 'NONE',  ( 1.000000000000000000, 0.000000000000000000, 0.000000000000000000 ) ) ;
#16531=AXIS2_PLACEMENT_3D ( 'NONE', #9556, #20321, #20176 ) ;
#16533=EDGE_CURVE ( 'NONE', #18280, #8829, #10112, .T. ) ;
#16536=CARTESIAN_POINT ( 'NONE',  ( -209.7353312573863207, 74.09610071451170654, -35.01412046639265441 ) ) ;
#16539=LINE ( 'NONE', #12240, #6922 ) ;
#16540=DIRECTION ( 'NONE',  ( 0.000000000000000000, 0.000000000000000000, -1.000000000000000000 ) ) ;
#16542=CARTESIAN_POINT ( 'NONE',  ( 119.1208832861758538, 235.9842039383417784, -100.0000000000002842 ) ) ;
#16546=ORIENTED_EDGE ( 'NONE', *, *, #18181, .F. ) ;
#16548=ORIENTED_EDGE ( 'NONE', *, *, #15435, .T. ) ;
#16549=CIRCLE ( 'NONE', #21583, 24.07986109634097005 ) ;
#16555=EDGE_CURVE ( 'NONE', #26681, #26218, #26553, .T. ) ;
#16557=DIRECTION ( 'NONE',  ( -1.000000000000000000, 0.000000000000000000, 0.000000000000000000 ) ) ;
#16564=CARTESIAN_POINT ( 'NONE',  ( 109.9999999999999432, 140.0000000000000000, -99.99999999999998579 ) ) ;
#16565=CARTESIAN_POINT ( 'NONE',  ( 65.00000000000000000, -120.0000000000000995, -63.97499999999998721 ) ) ;
#16567=EDGE_CURVE ( 'NONE', #16772, #12468, #1343, .T. ) ;
#16568=LINE ( 'NONE', #12692, #20227 ) ;
#16573=LINE ( 'NONE', #3621, #847 ) ;
#16582=CARTESIAN_POINT ( 'NONE',  ( 89.99999999999994316, -70.00000000000001421, -25.00000000000000000 ) ) ;
#16583=ORIENTED_EDGE ( 'NONE', *, *, #17352, .F. ) ;
#16586=ORIENTED_EDGE ( 'NONE', *, *, #24297, .T. ) ;
#16593=ORIENTED_EDGE ( 'NONE', *, *, #1564, .T. ) ;
#16594=ADVANCED_FACE ( 'NONE', ( #6921, #23886 ), #19995, .F. ) ;
#16598=VERTEX_POINT ( 'NONE', #2040 ) ;
#16600=CARTESIAN_POINT ( 'NONE',  ( 109.7119445821606121, 256.4759837302462984, 40.72317850545354645 ) ) ;
#16602=CARTESIAN_POINT ( 'NONE',  ( -146.6428522700808230, 17.24192588826928585, 83.00000000000001421 ) ) ;
#16603=FACE_OUTER_BOUND ( 'NONE', #9521, .T. ) ;
#16607=CARTESIAN_POINT ( 'NONE',  ( -205.7061355896894383, 146.0477147645469813, -13.00000000000000000 ) ) ;
#16610=CIRCLE ( 'NONE', #18896, 11.00000000000001066 ) ;
#16620=DIRECTION ( 'NONE',  ( 0.000000000000000000, 0.000000000000000000, -1.000000000000000000 ) ) ;
#16623=ORIENTED_EDGE ( 'NONE', *, *, #27676, .T. ) ;
#16624=DIRECTION ( 'NONE',  ( 0.000000000000000000, -1.000000000000000000, 0.000000000000000000 ) ) ;
#16629=AXIS2_PLACEMENT_3D ( 'NONE', #1718, #12381, #18968 ) ;
#16630=ORIENTED_EDGE ( 'NONE', *, *, #3981, .F. ) ;
#16633=CARTESIAN_POINT ( 'NONE',  ( 112.5174913703662014, 221.0249876999270953, 96.63436734148048401 ) ) ;
#16634=DIRECTION ( 'NONE',  ( 0.000000000000000000, 0.000000000000000000, -1.000000000000000000 ) ) ;
#16638=CARTESIAN_POINT ( 'NONE',  ( -197.4451421692467079, 62.05060586452424332, 32.13681025546651426 ) ) ;
#16640=CARTESIAN_POINT ( 'NONE',  ( -82.58132619288578269, 136.4857224512149116, -13.47873422864532955 ) ) ;
#16641=ADVANCED_FACE ( 'NONE', ( #21869, #12983 ), #26172, .T. ) ;
#16643=CARTESIAN_POINT ( 'NONE',  ( -206.0012425902573909, 90.39787868968801376, 28.20958337426846541 ) ) ;
#16646=EDGE_LOOP ( 'NONE', ( #8068, #13266 ) ) ;
#16650=CARTESIAN_POINT ( 'NONE',  ( -215.4886702565632390, 139.8420026707766226, -13.00000000000000000 ) ) ;
#16654=CIRCLE ( 'NONE', #26278, 22.49999999999997868 ) ;
#16662=VERTEX_POINT ( 'NONE', #2898 ) ;
#16663=ORIENTED_EDGE ( 'NONE', *, *, #5625, .F. ) ;
#16665=CIRCLE ( 'NONE', #2897, 64.76834224489934400 ) ;
#16666=DIRECTION ( 'NONE',  ( -0.000000000000000000, -0.000000000000000000, -1.000000000000000000 ) ) ;
#16670=CARTESIAN_POINT ( 'NONE',  ( 109.9513937765169516, 257.9883255678629439, -43.25762702467091003 ) ) ;
#16671=CARTESIAN_POINT ( 'NONE',  ( -13.46517964523875399, 129.5882704147440450, -16.86081371659212991 ) ) ;
#16672=DIRECTION ( 'NONE',  ( -0.000000000000000000, -0.000000000000000000, 1.000000000000000000 ) ) ;
#16675=DIRECTION ( 'NONE',  ( -1.000000000000000000, -2.602085213965211135E-16, 0.000000000000000000 ) ) ;
#16677=DIRECTION ( 'NONE',  ( -0.000000000000000000, -1.000000000000000000, -0.000000000000000000 ) ) ;
#16679=ORIENTED_EDGE ( 'NONE', *, *, #18536, .T. ) ;
#16680=AXIS2_PLACEMENT_3D ( 'NONE', #21140, #16980, #23727 ) ;
#16681=CARTESIAN_POINT ( 'NONE',  ( -191.4269953611151891, 102.1549118977063699, 32.85580523774468986 ) ) ;
#16686=VERTEX_POINT ( 'NONE', #18413 ) ;
#16688=VECTOR ( 'NONE', #22041, 1000.000000000000000 ) ;
#16689=VERTEX_POINT ( 'NONE', #16268 ) ;
#16691=CARTESIAN_POINT ( 'NONE',  ( 94.38583646783938264, 113.6320904521619610, 99.99999999997838529 ) ) ;
#16693=EDGE_CURVE ( 'NONE', #5551, #15968, #5046, .T. ) ;
#16699=FACE_OUTER_BOUND ( 'NONE', #11444, .T. ) ;
#16702=ORIENTED_EDGE ( 'NONE', *, *, #17079, .T. ) ;
#16703=VECTOR ( 'NONE', #8116, 1000.000000000000000 ) ;
#16706=DIRECTION ( 'NONE',  ( 0.9682458365518510357, -2.433928644932298160E-14, -0.2500000000000128231 ) ) ;
#16710=CARTESIAN_POINT ( 'NONE',  ( 119.9999999999999289, 110.0000000000000142, 100.0000000000000142 ) ) ;
#16713=CARTESIAN_POINT ( 'NONE',  ( 65.00000000000000000, -120.0000000000000995, -69.99999999999998579 ) ) ;
#16714=CARTESIAN_POINT ( 'NONE',  ( 134.9999999999998579, 220.0000000000000284, 84.99999999999995737 ) ) ;
#16716=LINE ( 'NONE', #5082, #22683 ) ;
#16718=CARTESIAN_POINT ( 'NONE',  ( 134.9999999999998579, 220.0000000000000284, -90.00000000000002842 ) ) ;
#16723=DIRECTION ( 'NONE',  ( 0.000000000000000000, 0.000000000000000000, 1.000000000000000000 ) ) ;
#16725=CARTESIAN_POINT ( 'NONE',  ( 79.99999999999994316, -40.00000000000002842, 70.00000000000001421 ) ) ;
#16727=VERTEX_POINT ( 'NONE', #25020 ) ;
#16730=CARTESIAN_POINT ( 'NONE',  ( 109.8949283312402088, 257.8851048416491949, 41.33580947111263981 ) ) ;
#16732=AXIS2_PLACEMENT_3D ( 'NONE', #6151, #17207, #19782 ) ;
#16734=DIRECTION ( 'NONE',  ( 0.000000000000000000, 0.000000000000000000, -1.000000000000000000 ) ) ;
#16735=ORIENTED_EDGE ( 'NONE', *, *, #23129, .T. ) ;
#16739=ORIENTED_EDGE ( 'NONE', *, *, #16533, .F. ) ;
#16742=CARTESIAN_POINT ( 'NONE',  ( -175.8417606860892874, 246.9430296707336652, -15.00000000000000000 ) ) ;
#16745=CARTESIAN_POINT ( 'NONE',  ( 115.9275995189148603, 208.0497038390087710, -99.13875753836940419 ) ) ;
#16747=CARTESIAN_POINT ( 'NONE',  ( -220.6363270246462776, 61.10744949787153502, -10.70339401868749896 ) ) ;
#16749=CARTESIAN_POINT ( 'NONE',  ( -17.24491960465746132, 75.97823757117562593, 100.0000000000000000 ) ) ;
#16764=DIRECTION ( 'NONE',  ( 0.000000000000000000, 0.000000000000000000, -1.000000000000000000 ) ) ;
#16765=ORIENTED_EDGE ( 'NONE', *, *, #14843, .F. ) ;
#16769=CARTESIAN_POINT ( 'NONE',  ( -62.44622725233823246, 134.9080593881841139, 13.78052965331430180 ) ) ;
#16772=VERTEX_POINT ( 'NONE', #20282 ) ;
#16774=LINE ( 'NONE', #7860, #18700 ) ;
#16775=PLANE ( 'NONE',  #11147 ) ;
#16776=CARTESIAN_POINT ( 'NONE',  ( -141.7175972931275680, 126.5060204430971140, -18.19504477830727751 ) ) ;
#16782=CARTESIAN_POINT ( 'NONE',  ( -224.1971796646980408, 86.90724828645529954, 16.84710691662892046 ) ) ;
#16783=CARTESIAN_POINT ( 'NONE',  ( -221.3650667873343139, -91.18033988749901653, 0.000000000000000000 ) ) ;
#16786=CIRCLE ( 'NONE', #1190, 2.000000000000000000 ) ;
#16789=CARTESIAN_POINT ( 'NONE',  ( -45.67245149924918479, -18.36872794415985766, 100.0000000000000142 ) ) ;
#16792=AXIS2_PLACEMENT_3D ( 'NONE', #11642, #1123, #25255 ) ;
#16794=ORIENTED_EDGE ( 'NONE', *, *, #1814, .F. ) ;
#16802=AXIS2_PLACEMENT_3D ( 'NONE', #26080, #23795, #2090 ) ;
#16804=EDGE_CURVE ( 'NONE', #19256, #9167, #22861, .T. ) ;
#16807=CARTESIAN_POINT ( 'NONE',  ( 107.9379936443569221, 247.3367456615697222, -33.97043262446585743 ) ) ;
#16808=DIRECTION ( 'NONE',  ( -0.000000000000000000, -0.000000000000000000, -1.000000000000000000 ) ) ;
#16812=CARTESIAN_POINT ( 'NONE',  ( -214.2457779686714900, 55.07866962813993439, -44.91461755630191277 ) ) ;
#16813=EDGE_CURVE ( 'NONE', #11368, #25971, #16406, .T. ) ;
#16819=CARTESIAN_POINT ( 'NONE',  ( -40.40953891503691153, 0.000000000000000000, 99.00000000000000000 ) ) ;
#16820=VERTEX_POINT ( 'NONE', #3308 ) ;
#16822=CARTESIAN_POINT ( 'NONE',  ( -189.6972266830665603, 103.6065584371345949, 32.02885553339256575 ) ) ;
#16823=DIRECTION ( 'NONE',  ( -0.000000000000000000, -0.000000000000000000, -1.000000000000000000 ) ) ;
#16826=ORIENTED_EDGE ( 'NONE', *, *, #15701, .T. ) ;
#16828=CARTESIAN_POINT ( 'NONE',  ( 85.90765579567833754, 110.5723347145563338, 99.99999999998919975 ) ) ;
#16829=CARTESIAN_POINT ( 'NONE',  ( -203.2481855153402250, 92.57460631283319685, -29.78692811926998729 ) ) ;
#16830=ORIENTED_EDGE ( 'NONE', *, *, #22149, .T. ) ;
#16838=AXIS2_PLACEMENT_3D ( 'NONE', #3433, #25276, #5598 ) ;
#16840=AXIS2_PLACEMENT_3D ( 'NONE', #24541, #9318, #2837 ) ;
#16841=EDGE_CURVE ( 'NONE', #19335, #6913, #11924, .T. ) ;
#16843=CARTESIAN_POINT ( 'NONE',  ( 109.9999999999999289, -90.00000000000001421, -25.00000000000000000 ) ) ;
#16844=CARTESIAN_POINT ( 'NONE',  ( -33.75989249264057435, 129.4008931478827833, -15.57934110460595001 ) ) ;
#16847=CARTESIAN_POINT ( 'NONE',  ( -189.5876332061210405, 103.4736392598993717, -32.83942934983755890 ) ) ;
#16848=ORIENTED_EDGE ( 'NONE', *, *, #26281, .F. ) ;
#16849=DIRECTION ( 'NONE',  ( -0.000000000000000000, 1.000000000000000000, -0.000000000000000000 ) ) ;
#16853=CARTESIAN_POINT ( 'NONE',  ( 65.00000000000000000, -120.0000000000000995, -69.99999999999998579 ) ) ;
#16862=DIRECTION ( 'NONE',  ( -0.000000000000000000, 1.000000000000000000, -0.000000000000000000 ) ) ;
#16864=EDGE_LOOP ( 'NONE', ( #20314, #16034, #13810, #9028 ) ) ;
#16868=ORIENTED_EDGE ( 'NONE', *, *, #23404, .F. ) ;
#16874=CARTESIAN_POINT ( 'NONE',  ( -244.5479615644635487, 75.99513337129094737, 5.000000000000002665 ) ) ;
#16876=EDGE_CURVE ( 'NONE', #3706, #17245, #1439, .T. ) ;
#16877=CARTESIAN_POINT ( 'NONE',  ( -180.0000000000000284, 59.99999999999994316, 70.00000000000000000 ) ) ;
#16878=CARTESIAN_POINT ( 'NONE',  ( -5.301155171372935904, 133.7253830476667247, 14.04417486721310127 ) ) ;
#16880=CARTESIAN_POINT ( 'NONE',  ( 119.9999999999999432, 2.220446049250311819E-14, -100.0000000000000142 ) ) ;
#16881=CARTESIAN_POINT ( 'NONE',  ( -218.4636426211937987, 60.67881959240489920, -11.81164476506858207 ) ) ;
#16882=FACE_OUTER_BOUND ( 'NONE', #23707, .T. ) ;
#16889=CIRCLE ( 'NONE', #25144, 30.00000000000000000 ) ;
#16893=VERTEX_POINT ( 'NONE', #16959 ) ;
#16900=( BOUNDED_SURFACE ( )  B_SPLINE_SURFACE ( 3, 2, ( 
 ( #18048, #2373, #6556 ),
 ( #4527, #6833, #17751 ),
 ( #13180, #20046, #26366 ),
 ( #24223, #15336, #26502 ),
 ( #4670, #4958, #15615 ),
 ( #26806, #20195, #2807 ),
 ( #4817, #24358, #22210 ),
 ( #13316, #22066, #9435 ),
 ( #523, #11599, #11306 ),
 ( #8852, #380, #17611 ),
 ( #19765, #6695, #15908 ),
 ( #15476, #11155, #20339 ),
 ( #13458, #2662, #6973 ),
 ( #2514, #9139, #667 ),
 ( #17900, #2229, #8998 ),
 ( #18197, #90, #239 ),
 ( #24089, #21923, #11014 ),
 ( #26648, #19909, #15763 ),
 ( #24510, #13606, #7128 ),
 ( #22354, #11451, #4395 ),
 ( #9283, #24653, #13748 ),
 ( #22499, #16044, #9710 ),
 ( #14169, #5251, #3226 ),
 ( #1082, #11878, #13896 ),
 ( #27356, #5677, #27492 ),
 ( #7830, #16600, #7695 ),
 ( #20482, #23202, #27222 ),
 ( #12159, #7415, #9573 ),
 ( #807, #21038, #18334 ),
 ( #7563, #5532, #22922 ) ),
 .UNSPECIFIED., .F., .F., .F. ) 
 B_SPLINE_SURFACE_WITH_KNOTS ( ( 4, 2, 2, 2, 2, 2, 2, 2, 2, 2, 2, 2, 2, 2, 4 ),
 ( 3, 3 ),
 ( 0.000000000000000000, 0.003854887539719073237, 0.007709775079438146474, 0.009637218849297683743, 0.01156466261915722014, 0.01541955015887629295, 0.01927443769859536749, 0.02312932523831444029, 0.03083910031775258589, 0.03469398785747165870, 0.03854887539719073497, 0.04625865047662888058, 0.05396842555606702618, 0.05782331309578610246, 0.06167820063550517179 ),
 ( 0.000000000000000000, 1.000000000000000000 ),
 .UNSPECIFIED. ) 
 GEOMETRIC_REPRESENTATION_ITEM ( )  RATIONAL_B_SPLINE_SURFACE ( (
 ( 1.000000000000000000, 0.7071067811865476838, 1.000000000000000000),
 ( 1.000000000000000000, 0.7108376764366090006, 1.000000000000000000),
 ( 1.000000000000000000, 0.7158505121290739126, 1.000000000000000000),
 ( 1.000000000000000000, 0.7278978148820525185, 1.000000000000000000),
 ( 1.000000000000000000, 0.7349313210305764565, 1.000000000000000000),
 ( 1.000000000000000000, 0.7466216138176463568, 1.000000000000000000),
 ( 1.000000000000000000, 0.7507087799370647518, 1.000000000000000000),
 ( 1.000000000000000000, 0.7592063458285337463, 1.000000000000000000),
 ( 1.000000000000000000, 0.7635836989923795448, 1.000000000000000000),
 ( 1.000000000000000000, 0.7769550404246040598, 1.000000000000000000),
 ( 1.000000000000000000, 0.7862062597107043471, 1.000000000000000000),
 ( 1.000000000000000000, 0.8049739164098205224, 1.000000000000000000),
 ( 1.000000000000000000, 0.8144916847796412895, 1.000000000000000000),
 ( 1.000000000000000000, 0.8334855532651173071, 1.000000000000000000),
 ( 1.000000000000000000, 0.8428380035008721238, 1.000000000000000000),
 ( 1.000000000000000000, 0.8700856926953133286, 1.000000000000000000),
 ( 1.000000000000000000, 0.8872021369655685996, 1.000000000000000000),
 ( 1.000000000000000000, 0.9106340391008400648, 1.000000000000000000),
 ( 1.000000000000000000, 0.9180764524646015667, 1.000000000000000000),
 ( 1.000000000000000000, 0.9321377268943903394, 1.000000000000000000),
 ( 1.000000000000000000, 0.9386792981679147330, 1.000000000000000000),
 ( 1.000000000000000000, 0.9568359836586407541, 1.000000000000000000),
 ( 1.000000000000000000, 0.9669855263615203533, 1.000000000000000000),
 ( 1.000000000000000000, 0.9833405099229461932, 1.000000000000000000),
 ( 1.000000000000000000, 0.9895476861110599209, 1.000000000000000000),
 ( 1.000000000000000000, 0.9958061391665089523, 1.000000000000000000),
 ( 1.000000000000000000, 0.9973811977639622794, 1.000000000000000000),
 ( 1.000000000000000000, 0.9994757700715640736, 1.000000000000000000),
 ( 1.000000000000000000, 1.000000000000000000, 1.000000000000000000),
 ( 1.000000000000000000, 1.000000000000000000, 1.000000000000000000) ) ) 
 REPRESENTATION_ITEM ( '' )  SURFACE ( )  );
#16901=EDGE_CURVE ( 'NONE', #18743, #10961, #15811, .T. ) ;
#16908=CARTESIAN_POINT ( 'NONE',  ( -43.02437977270766822, 129.7200458115293031, -16.81627168235288394 ) ) ;
#16909=CARTESIAN_POINT ( 'NONE',  ( 9.999999999999749534, 90.00000000000001421, 110.0000000000000284 ) ) ;
#16910=AXIS2_PLACEMENT_3D ( 'NONE', #17983, #7210, #9513 ) ;
#16911=CARTESIAN_POINT ( 'NONE',  ( -149.1990966351883117, 125.0787559347685658, -18.94696671105487695 ) ) ;
#16912=CARTESIAN_POINT ( 'NONE',  ( -200.0000000000000284, -91.18033988749901653, 0.000000000000000000 ) ) ;
#16913=CARTESIAN_POINT ( 'NONE',  ( -229.2498027451139251, 132.0565166830976693, 13.00000000000000000 ) ) ;
#16914=CARTESIAN_POINT ( 'NONE',  ( -232.7412786160992084, 91.52974244978815932, -14.99999999999999645 ) ) ;
#16917=AXIS2_PLACEMENT_3D ( 'NONE', #10309, #25252, #21220 ) ;
#16918=CARTESIAN_POINT ( 'NONE',  ( -222.0883063321265638, 86.46654056963494384, 17.72095034480506470 ) ) ;
#16920=CARTESIAN_POINT ( 'NONE',  ( -156.8436863811589603, 180.7779002010536544, 15.00000000000000000 ) ) ;
#16924=ADVANCED_FACE ( 'NONE', ( #7911 ), #9018, .T. ) ;
#16925=CARTESIAN_POINT ( 'NONE',  ( -44.64074837118231187, -18.63255001205507355, 99.96486222153572498 ) ) ;
#16929=ORIENTED_EDGE ( 'NONE', *, *, #21905, .F. ) ;
#16931=CARTESIAN_POINT ( 'NONE',  ( 107.0062495987152715, 249.1467455478701822, -31.68887795646429240 ) ) ;
#16934=EDGE_CURVE ( 'NONE', #11042, #7588, #147, .T. ) ;
#16937=EDGE_LOOP ( 'NONE', ( #1667, #13031, #12346, #26736 ) ) ;
#16941=VECTOR ( 'NONE', #1288, 1000.000000000000000 ) ;
#16942=EDGE_CURVE ( 'NONE', #16979, #12184, #1364, .T. ) ;
#16944=EDGE_CURVE ( 'NONE', #25070, #25446, #12042, .T. ) ;
#16945=FACE_OUTER_BOUND ( 'NONE', #23288, .T. ) ;
#16947=CONICAL_SURFACE ( 'NONE', #13289, 16.36034929305424512, 0.08885387018394150238 ) ;
#16951=CARTESIAN_POINT ( 'NONE',  ( -207.5699030661693030, 75.55056756148773900, -43.24289214104831558 ) ) ;
#16954=DIRECTION ( 'NONE',  ( -1.000000000000000000, 0.000000000000000000, 0.000000000000000000 ) ) ;
#16959=CARTESIAN_POINT ( 'NONE',  ( -42.99650729631200363, 36.92584315232891612, 99.00000000000000000 ) ) ;
#16960=AXIS2_PLACEMENT_3D ( 'NONE', #11915, #26841, #24972 ) ;
#16961=DIRECTION ( 'NONE',  ( -3.469446951953614189E-16, 1.000000000000000000, 0.000000000000000000 ) ) ;
#16963=ORIENTED_EDGE ( 'NONE', *, *, #25902, .T. ) ;
#16966=CIRCLE ( 'NONE', #18373, 6.025000000000002132 ) ;
#16974=CARTESIAN_POINT ( 'NONE',  ( 107.0237601845336712, 245.0637783987590694, 31.95154820714027366 ) ) ;
#16976=CARTESIAN_POINT ( 'NONE',  ( -189.6091703120771967, 103.6687479389959350, -32.02356223315309336 ) ) ;
#16977=ORIENTED_EDGE ( 'NONE', *, *, #27785, .T. ) ;
#16979=VERTEX_POINT ( 'NONE', #2720 ) ;
#16980=DIRECTION ( 'NONE',  ( 1.000000000000000000, 0.000000000000000000, 0.000000000000000000 ) ) ;
#16981=CYLINDRICAL_SURFACE ( 'NONE', #24990, 5.000000000000004441 ) ;
#16982=CARTESIAN_POINT ( 'NONE',  ( -524.0002167759885197, -169.4627935898112696, 0.000000000000000000 ) ) ;
#16985=CIRCLE ( 'NONE', #5528, 2.000000000000000000 ) ;
#16986=DIRECTION ( 'NONE',  ( -0.000000000000000000, -0.000000000000000000, -1.000000000000000000 ) ) ;
#16990=ORIENTED_EDGE ( 'NONE', *, *, #23570, .F. ) ;
#16994=CARTESIAN_POINT ( 'NONE',  ( -27.13451380343252595, 127.9642796392991784, -17.52013407737619488 ) ) ;
#16995=CARTESIAN_POINT ( 'NONE',  ( -207.4141359493844732, 90.18508254785665201, 25.67621972994781387 ) ) ;
#16996=ORIENTED_EDGE ( 'NONE', *, *, #23175, .F. ) ;
#17002=ORIENTED_EDGE ( 'NONE', *, *, #26185, .F. ) ;
#17003=ADVANCED_FACE ( 'NONE', ( #26561 ), #18246, .T. ) ;
#17015=CARTESIAN_POINT ( 'NONE',  ( -76.25760768171835480, 221.6666220619076739, -13.00000000000000000 ) ) ;
#17017=CARTESIAN_POINT ( 'NONE',  ( -220.5365384948384531, 71.33200643683619546, -21.30906822952401924 ) ) ;
#17023=CARTESIAN_POINT ( 'NONE',  ( 112.6399768800336005, 217.4434959555082116, -96.77053691278551639 ) ) ;
#17024=ORIENTED_EDGE ( 'NONE', *, *, #18181, .T. ) ;
#17026=CIRCLE ( 'NONE', #14296, 2.000000000000012879 ) ;
#17033=CIRCLE ( 'NONE', #20231, 30.00000000000000000 ) ;
#17034=EDGE_CURVE ( 'NONE', #20037, #11369, #4107, .T. ) ;
#17036=VERTEX_POINT ( 'NONE', #22554 ) ;
#17039=EDGE_LOOP ( 'NONE', ( #11080, #9123, #2735, #15358, #22808, #12948 ) ) ;
#17040=CARTESIAN_POINT ( 'NONE',  ( -86.54628362417027176, 136.4599498150971613, 13.48322064102051776 ) ) ;
#17042=VERTEX_POINT ( 'NONE', #4729 ) ;
#17045=CARTESIAN_POINT ( 'NONE',  ( -141.5841712291289127, 126.5472752318202936, -18.17431859372913294 ) ) ;
#17047=ADVANCED_FACE ( 'NONE', ( #8717 ), #93, .F. ) ;
#17049=CARTESIAN_POINT ( 'NONE',  ( -112.9218146637504674, 134.5565441768181074, -15.44239355050386564 ) ) ;
#17055=CARTESIAN_POINT ( 'NONE',  ( -216.2998406815053443, 86.35807036193234865, -20.83938377197658198 ) ) ;
#17058=DIRECTION ( 'NONE',  ( 1.000000000000000000, -0.000000000000000000, -0.000000000000000000 ) ) ;
#17062=CYLINDRICAL_SURFACE ( 'NONE', #22453, 41.00000000000000711 ) ;
#17067=EDGE_CURVE ( 'NONE', #26118, #17211, #10532, .T. ) ;
#17069=CARTESIAN_POINT ( 'NONE',  ( 87.50000000000029843, 230.0000000000000000, -15.95262490344447137 ) ) ;
#17072=AXIS2_PLACEMENT_3D ( 'NONE', #13238, #17528, #24427 ) ;
#17078=CARTESIAN_POINT ( 'NONE',  ( -210.7172313291012529, 103.7585653882801182, 15.00000000000000000 ) ) ;
#17079=EDGE_CURVE ( 'NONE', #27477, #10183, #20166, .T. ) ;
#17081=DIRECTION ( 'NONE',  ( 0.000000000000000000, 0.000000000000000000, 1.000000000000000000 ) ) ;
#17083=VECTOR ( 'NONE', #18228, 1000.000000000000000 ) ;
#17094=VECTOR ( 'NONE', #22615, 1000.000000000000000 ) ;
#17099=CARTESIAN_POINT ( 'NONE',  ( -231.2228484428727882, 90.30500068246439582, -15.11033134556762114 ) ) ;
#17100=ADVANCED_FACE ( 'NONE', ( #8856 ), #16947, .T. ) ;
#17102=EDGE_LOOP ( 'NONE', ( #23928, #16583, #18036, #1068 ) ) ;
#17104=EDGE_CURVE ( 'NONE', #7444, #27055, #15479, .T. ) ;
#17109=CARTESIAN_POINT ( 'NONE',  ( 90.17595424780135716, 111.7661400906778937, 100.0000000000108429 ) ) ;
#17111=ORIENTED_EDGE ( 'NONE', *, *, #2155, .T. ) ;
#17114=CARTESIAN_POINT ( 'NONE',  ( 88.58553289618420479, 111.2425746093144880, -99.99999999998921396 ) ) ;
#17116=CARTESIAN_POINT ( 'NONE',  ( 104.2818955975975541, 239.9330879431699657, 27.31284324272755271 ) ) ;
#17119=CARTESIAN_POINT ( 'NONE',  ( -225.0771096875090223, 87.16154696420846903, 16.52804872244989198 ) ) ;
#17120=EDGE_LOOP ( 'NONE', ( #10054, #11629 ) ) ;
#17121=FACE_OUTER_BOUND ( 'NONE', #408, .T. ) ;
#17126=ORIENTED_EDGE ( 'NONE', *, *, #4585, .T. ) ;
#17136=EDGE_CURVE ( 'NONE', #13809, #18951, #24091, .T. ) ;
#17138=DIRECTION ( 'NONE',  ( 0.000000000000000000, 0.000000000000000000, 1.000000000000000000 ) ) ;
#17142=EDGE_LOOP ( 'NONE', ( #66, #28390, #11208, #6674 ) ) ;
#17143=CARTESIAN_POINT ( 'NONE',  ( 65.00000000000000000, -120.0000000000000995, -76.02499999999999147 ) ) ;
#17144=CARTESIAN_POINT ( 'NONE',  ( -169.9564382400993168, 115.7522936420806445, -25.38211417480260579 ) ) ;
#17146=AXIS2_PLACEMENT_3D ( 'NONE', #26977, #704, #9474 ) ;
#17147=ORIENTED_EDGE ( 'NONE', *, *, #804, .T. ) ;
#17148=CARTESIAN_POINT ( 'NONE',  ( -112.3709231662415675, 70.58802258329811252, 82.86315325844958579 ) ) ;
#17155=CARTESIAN_POINT ( 'NONE',  ( -205.7061355896892678, 146.0477147645463845, -15.00000000000000000 ) ) ;
#17159=LINE ( 'NONE', #19034, #26872 ) ;
#17160=CARTESIAN_POINT ( 'NONE',  ( -233.3699482038443023, 66.30323757541319196, -6.318463073149253262 ) ) ;
#17164=CARTESIAN_POINT ( 'NONE',  ( -216.4421519707229891, 141.6000904446840707, -13.00000000000000000 ) ) ;
#17166=CARTESIAN_POINT ( 'NONE',  ( 113.0497540245546304, 214.9557400730136578, -97.19889357486846393 ) ) ;
#17172=EDGE_CURVE ( 'NONE', #16820, #18456, #13311, .T. ) ;
#17173=DIRECTION ( 'NONE',  ( 1.000000000000000000, -0.000000000000000000, -0.000000000000000000 ) ) ;
#17179=ORIENTED_EDGE ( 'NONE', *, *, #20845, .F. ) ;
#17180=FACE_OUTER_BOUND ( 'NONE', #19306, .T. ) ;
#17181=VERTEX_POINT ( 'NONE', #1085 ) ;
#17183=ORIENTED_EDGE ( 'NONE', *, *, #27848, .F. ) ;
#17186=ORIENTED_EDGE ( 'NONE', *, *, #10526, .T. ) ;
#17190=CARTESIAN_POINT ( 'NONE',  ( -77.57255112795054686, 134.6586583231760130, -15.47697172941245469 ) ) ;
#17192=CARTESIAN_POINT ( 'NONE',  ( -156.0897298158335786, 122.3430908625673794, -20.70325525780628695 ) ) ;
#17193=CIRCLE ( 'NONE', #8929, 7.500000000000007105 ) ;
#17194=EDGE_CURVE ( 'NONE', #10216, #13911, #18889, .T. ) ;
#17196=EDGE_CURVE ( 'NONE', #15348, #7126, #9642, .T. ) ;
#17197=LINE ( 'NONE', #10741, #27772 ) ;
#17198=CARTESIAN_POINT ( 'NONE',  ( -222.5626178033668623, 88.43593056344644765, -17.20029664898224198 ) ) ;
#17203=CARTESIAN_POINT ( 'NONE',  ( -160.0000000000000284, 59.99999999999994316, -100.0000000000000142 ) ) ;
#17207=DIRECTION ( 'NONE',  ( 0.000000000000000000, -1.000000000000000000, 0.000000000000000000 ) ) ;
#17208=TOROIDAL_SURFACE ( 'NONE', #11712, 60.90601976618767566, 2.000000000000000000 ) ;
#17211=VERTEX_POINT ( 'NONE', #9438 ) ;
#17213=CARTESIAN_POINT ( 'NONE',  ( 90.45806322832901003, 239.6644751351067271, -16.82109631826974905 ) ) ;
#17214=ORIENTED_EDGE ( 'NONE', *, *, #16942, .T. ) ;
#17216=AXIS2_PLACEMENT_3D ( 'NONE', #21338, #2938, #7256 ) ;
#17217=VERTEX_POINT ( 'NONE', #12016 ) ;
#17220=ORIENTED_EDGE ( 'NONE', *, *, #19066, .F. ) ;
#17231=CARTESIAN_POINT ( 'NONE',  ( -232.2321867067640824, 76.70661131974999591, -15.57447242055394199 ) ) ;
#17232=CARTESIAN_POINT ( 'NONE',  ( -27.00790996259407706, 129.1643630886944720, 15.68707935331008940 ) ) ;
#17233=CARTESIAN_POINT ( 'NONE',  ( -209.4684267455243116, 67.32361167506066124, 34.40574903147302877 ) ) ;
#17235=CARTESIAN_POINT ( 'NONE',  ( -76.25760768171836901, 154.8982798170083299, 12.99999999999999822 ) ) ;
#17236=EDGE_LOOP ( 'NONE', ( #11654, #8456, #7747, #13583 ) ) ;
#17237=CARTESIAN_POINT ( 'NONE',  ( -177.9077837340308008, 111.2757406836244627, 29.50435359264835000 ) ) ;
#17239=EDGE_CURVE ( 'NONE', #2614, #12013, #16966, .T. ) ;
#17245=VERTEX_POINT ( 'NONE', #22925 ) ;
#17252=CARTESIAN_POINT ( 'NONE',  ( 114.5273445118729541, 107.2595481030940761, -100.0000000000000142 ) ) ;
#17256=ORIENTED_EDGE ( 'NONE', *, *, #11713, .F. ) ;
#17257=CARTESIAN_POINT ( 'NONE',  ( -218.9526947977414579, 86.19408851467024135, 19.27252192978178513 ) ) ;
#17258=ORIENTED_EDGE ( 'NONE', *, *, #25574, .F. ) ;
#17259=CARTESIAN_POINT ( 'NONE',  ( -175.0000000000000000, -120.0000000000001847, -69.99999999999998579 ) ) ;
#17260=CARTESIAN_POINT ( 'NONE',  ( 157.4999999999998579, 220.0000000000000284, -100.0000000000000142 ) ) ;
#17261=CARTESIAN_POINT ( 'NONE',  ( -115.3221550338875971, 71.54464929955099706, 82.80879831960034210 ) ) ;
#17262=CIRCLE ( 'NONE', #9473, 5.000000000000000888 ) ;
#17264=ORIENTED_EDGE ( 'NONE', *, *, #3963, .F. ) ;
#17271=DIRECTION ( 'NONE',  ( 0.000000000000000000, 0.000000000000000000, 1.000000000000000000 ) ) ;
#17274=CARTESIAN_POINT ( 'NONE',  ( -178.0837196006577585, 111.1705890210531322, 28.96620944385036722 ) ) ;
#17275=CARTESIAN_POINT ( 'NONE',  ( -38.52381090778946060, 128.7773429936079310, -17.17645200753749180 ) ) ;
#17276=DIRECTION ( 'NONE',  ( 1.000000000000000000, 0.000000000000000000, 0.000000000000000000 ) ) ;
#17277=ORIENTED_EDGE ( 'NONE', *, *, #1563, .F. ) ;
#17278=CARTESIAN_POINT ( 'NONE',  ( 1.982541115402066017E-14, -150.0000000000000568, -100.0000000000000142 ) ) ;
#17281=CARTESIAN_POINT ( 'NONE',  ( -191.3917181558073253, 102.3917013931790478, -32.04925462112321100 ) ) ;
#17282=EDGE_LOOP ( 'NONE', ( #4760, #104, #9983, #483, #23649, #21063, #20165, #261 ) ) ;
#17286=ORIENTED_EDGE ( 'NONE', *, *, #17136, .T. ) ;
#17287=ORIENTED_EDGE ( 'NONE', *, *, #21976, .T. ) ;
#17292=EDGE_CURVE ( 'NONE', #24530, #20507, #11881, .T. ) ;
#17297=CARTESIAN_POINT ( 'NONE',  ( -223.9727688501994578, 61.67225750692603015, -20.13450274023890785 ) ) ;
#17298=ORIENTED_EDGE ( 'NONE', *, *, #9379, .T. ) ;
#17305=CARTESIAN_POINT ( 'NONE',  ( -215.7935364303658901, 60.28281843632711912, 13.31033261678752844 ) ) ;
#17308=CARTESIAN_POINT ( 'NONE',  ( 9.999999999999964473, 60.00000000000001421, 80.00000000000001421 ) ) ;
#17312=VERTEX_POINT ( 'NONE', #20625 ) ;
#17315=CARTESIAN_POINT ( 'NONE',  ( -254.3350114625770289, -91.18033988749901653, -16.36034929305424512 ) ) ;
#17316=ORIENTED_EDGE ( 'NONE', *, *, #19565, .F. ) ;
#17318=FACE_OUTER_BOUND ( 'NONE', #1497, .T. ) ;
#17320=ORIENTED_EDGE ( 'NONE', *, *, #25863, .F. ) ;
#17322=ORIENTED_EDGE ( 'NONE', *, *, #26341, .F. ) ;
#17323=DIRECTION ( 'NONE',  ( 1.000000000000000000, 0.000000000000000000, 0.000000000000000000 ) ) ;
#17325=CARTESIAN_POINT ( 'NONE',  ( -143.9457187202836792, 125.8028027456154234, -18.55619470350388411 ) ) ;
#17326=FACE_OUTER_BOUND ( 'NONE', #10972, .T. ) ;
#17327=ADVANCED_FACE ( 'NONE', ( #1226 ), #20643, .T. ) ;
#17329=CARTESIAN_POINT ( 'NONE',  ( -156.8436863811591593, 180.7779002010535407, -15.00000000000000000 ) ) ;
#17333=CARTESIAN_POINT ( 'NONE',  ( -231.9378824387723057, 93.53122965655593646, -12.99999999999999645 ) ) ;
#17337=LINE ( 'NONE', #11026, #17814 ) ;
#17338=DIRECTION ( 'NONE',  ( 0.000000000000000000, 0.000000000000000000, 1.000000000000000000 ) ) ;
#17341=CIRCLE ( 'NONE', #4953, 29.99999999999999645 ) ;
#17345=CARTESIAN_POINT ( 'NONE',  ( -270.1025481742786951, -91.18033988749901653, 14.95564396479129243 ) ) ;
#17346=ORIENTED_EDGE ( 'NONE', *, *, #14413, .F. ) ;
#17347=CARTESIAN_POINT ( 'NONE',  ( 92.84236432024516716, 239.7913859916932040, -17.77233924293991407 ) ) ;
#17349=CARTESIAN_POINT ( 'NONE',  ( 6.333949844049013400, 140.1907388332623725, -13.00000000000000355 ) ) ;
#17352=EDGE_CURVE ( 'NONE', #8916, #17036, #25497, .T. ) ;
#17354=EDGE_LOOP ( 'NONE', ( #17418, #6328, #7003, #3763, #3148, #8169 ) ) ;
#17355=EDGE_LOOP ( 'NONE', ( #16253, #8662, #13962, #2718 ) ) ;
#17358=EDGE_CURVE ( 'NONE', #21631, #10760, #9992, .T. ) ;
#17359=AXIS2_PLACEMENT_3D ( 'NONE', #28378, #3978, #15201 ) ;
#17362=LINE ( 'NONE', #4292, #4564 ) ;
#17364=CARTESIAN_POINT ( 'NONE',  ( -42.99650729631200363, 71.03850157808263077, 99.00000000000000000 ) ) ;
#17366=CARTESIAN_POINT ( 'NONE',  ( 49.56615429303207065, 203.2034914284457159, 12.99999999999999822 ) ) ;
#17367=DIRECTION ( 'NONE',  ( -0.000000000000000000, -0.000000000000000000, -1.000000000000000000 ) ) ;
#17369=DIRECTION ( 'NONE',  ( -0.000000000000000000, -0.000000000000000000, -1.000000000000000000 ) ) ;
#17371=PLANE ( 'NONE',  #7749 ) ;
#17373=DIRECTION ( 'NONE',  ( 0.000000000000000000, 0.000000000000000000, -1.000000000000000000 ) ) ;
#17375=VERTEX_POINT ( 'NONE', #23626 ) ;
#17376=EDGE_LOOP ( 'NONE', ( #25941, #2397, #26877, #17490, #14964 ) ) ;
#17377=CARTESIAN_POINT ( 'NONE',  ( -232.1441312129731500, 91.01446451744486410, -15.02668720701366212 ) ) ;
#17385=VERTEX_POINT ( 'NONE', #8117 ) ;
#17388=EDGE_CURVE ( 'NONE', #6791, #8829, #12724, .T. ) ;
#17389=CARTESIAN_POINT ( 'NONE',  ( -222.0211651016019516, 135.7213904098416890, -12.97555235349485869 ) ) ;
#17390=DIRECTION ( 'NONE',  ( -1.000000000000000000, 0.000000000000000000, 0.000000000000000000 ) ) ;
#17392=CARTESIAN_POINT ( 'NONE',  ( 89.77759941121082932, 81.13568025369244197, -100.0000000000000142 ) ) ;
#17398=CARTESIAN_POINT ( 'NONE',  ( -227.2146340703364160, 90.21260626941095495, 15.67423580940634231 ) ) ;
#17401=AXIS2_PLACEMENT_3D ( 'NONE', #19646, #12770, #28251 ) ;
#17403=CARTESIAN_POINT ( 'NONE',  ( -37.82257053376181233, 71.03850157808263077, 99.00000000000000000 ) ) ;
#17405=AXIS2_PLACEMENT_3D ( 'NONE', #22421, #6758, #18118 ) ;
#17408=CARTESIAN_POINT ( 'NONE',  ( 117.2377723979408017, 206.1768395233783338, 99.61817846761982764 ) ) ;
#17411=CARTESIAN_POINT ( 'NONE',  ( 33.10302365956999182, 221.6666220619077876, -15.00000000000000000 ) ) ;
#17413=EDGE_CURVE ( 'NONE', #18824, #7691, #3671, .T. ) ;
#17415=AXIS2_PLACEMENT_3D ( 'NONE', #25565, #20980, #19111 ) ;
#17417=CARTESIAN_POINT ( 'NONE',  ( -203.7125816754261791, 92.59027862332997927, 28.49518943040505192 ) ) ;
#17418=ORIENTED_EDGE ( 'NONE', *, *, #20728, .T. ) ;
#17419=ORIENTED_EDGE ( 'NONE', *, *, #3994, .F. ) ;
#17420=AXIS2_PLACEMENT_3D ( 'NONE', #8129, #21196, #3241 ) ;
#17423=CARTESIAN_POINT ( 'NONE',  ( -164.5307643740429455, 118.5035042282064097, -22.94257969500540995 ) ) ;
#17425=VERTEX_POINT ( 'NONE', #12443 ) ;
#17430=CARTESIAN_POINT ( 'NONE',  ( 1.569447331094923070, 135.1286268723246167, 15.37625018068031757 ) ) ;
#17432=ADVANCED_FACE ( 'NONE', ( #23483 ), #3937, .T. ) ;
#17433=AXIS2_PLACEMENT_3D ( 'NONE', #671, #6977, #945 ) ;
#17437=DIRECTION ( 'NONE',  ( 0.000000000000000000, 0.000000000000000000, -1.000000000000000000 ) ) ;
#17439=DIRECTION ( 'NONE',  ( -1.000000000000000000, -2.602085213965211135E-16, 0.000000000000000000 ) ) ;
#17445=ORIENTED_EDGE ( 'NONE', *, *, #6390, .F. ) ;
#17446=EDGE_CURVE ( 'NONE', #366, #17857, #3796, .T. ) ;
#17451=DIRECTION ( 'NONE',  ( -3.469446951953614189E-16, 1.000000000000000000, -0.000000000000000000 ) ) ;
#17453=ORIENTED_EDGE ( 'NONE', *, *, #24991, .T. ) ;
#17464=ORIENTED_EDGE ( 'NONE', *, *, #6943, .T. ) ;
#17469=DIRECTION ( 'NONE',  ( -0.000000000000000000, -0.000000000000000000, 1.000000000000000000 ) ) ;
#17473=CARTESIAN_POINT ( 'NONE',  ( -221.9298065274946339, 88.28604124582930979, -17.46722815149482599 ) ) ;
#17477=LINE ( 'NONE', #13615, #14763 ) ;
#17478=CARTESIAN_POINT ( 'NONE',  ( 179.9999999999999147, -150.0000000000000284, -100.0000000000000142 ) ) ;
#17479=CARTESIAN_POINT ( 'NONE',  ( 157.4999999999998579, 220.0000000000000284, -99.00000000000001421 ) ) ;
#17483=CARTESIAN_POINT ( 'NONE',  ( 110.2602732333167808, 140.0000000000000000, 92.61747884359283489 ) ) ;
#17488=CARTESIAN_POINT ( 'NONE',  ( 102.0190107526883310, 244.0003474240100161, -16.44012727446676791 ) ) ;
#17490=ORIENTED_EDGE ( 'NONE', *, *, #4944, .T. ) ;
#17491=ORIENTED_EDGE ( 'NONE', *, *, #10219, .F. ) ;
#17492=VECTOR ( 'NONE', #28377, 1000.000000000000000 ) ;
#17494=ORIENTED_EDGE ( 'NONE', *, *, #2804, .T. ) ;
#17502=CARTESIAN_POINT ( 'NONE',  ( -216.4559255058941289, 59.30400871604422264, 28.11406665935853866 ) ) ;
#17504=LINE ( 'NONE', #6596, #6228 ) ;
#17511=CARTESIAN_POINT ( 'NONE',  ( -38.50235330400180089, 128.7731110165481141, 17.17814592602437429 ) ) ;
#17512=DIRECTION ( 'NONE',  ( -0.000000000000000000, -0.000000000000000000, 1.000000000000000000 ) ) ;
#17514=ADVANCED_FACE ( 'NONE', ( #10171 ), #11494, .T. ) ;
#17517=ORIENTED_EDGE ( 'NONE', *, *, #2266, .T. ) ;
#17520=CARTESIAN_POINT ( 'NONE',  ( -178.5327134719260869, 110.5652120027505703, 30.30295336851717991 ) ) ;
#17521=EDGE_CURVE ( 'NONE', #17838, #11217, #1680, .T. ) ;
#17522=CIRCLE ( 'NONE', #12052, 2.000000000000000444 ) ;
#17527=EDGE_LOOP ( 'NONE', ( #27578, #14976, #19784, #3993 ) ) ;
#17528=DIRECTION ( 'NONE',  ( 0.000000000000000000, 0.000000000000000000, 1.000000000000000000 ) ) ;
#17534=CIRCLE ( 'NONE', #8823, 66.76834224489934400 ) ;
#17535=CARTESIAN_POINT ( 'NONE',  ( -203.1779787704217313, 93.05164332230201296, -28.77272332722132475 ) ) ;
#17537=CARTESIAN_POINT ( 'NONE',  ( -228.4379895967119012, 88.56164859814569468, 15.57174740462524909 ) ) ;
#17538=AXIS2_PLACEMENT_3D ( 'NONE', #17758, #11312, #26813 ) ;
#17544=EDGE_CURVE ( 'NONE', #16772, #25545, #15611, .T. ) ;
#17545=VERTEX_POINT ( 'NONE', #6562 ) ;
#17546=CARTESIAN_POINT ( 'NONE',  ( 119.1208832861755269, 204.0157960616585910, 100.0000000000002274 ) ) ;
#17549=LINE ( 'NONE', #611, #23591 ) ;
#17551=AXIS2_PLACEMENT_3D ( 'NONE', #16909, #19342, #25663 ) ;
#17555=DIRECTION ( 'NONE',  ( 1.850371707708594316E-16, -1.000000000000000000, 0.000000000000000000 ) ) ;
#17562=EDGE_CURVE ( 'NONE', #25296, #7114, #4532, .T. ) ;
#17564=CARTESIAN_POINT ( 'NONE',  ( -175.0822582904459921, 112.9350779648750489, -28.38028793360534507 ) ) ;
#17567=CARTESIAN_POINT ( 'NONE',  ( -115.3221550338875971, 71.54464929955099706, 82.80879831960034210 ) ) ;
#17572=DIRECTION ( 'NONE',  ( 1.000000000000000000, -0.000000000000000000, -0.000000000000000000 ) ) ;
#17573=AXIS2_PLACEMENT_3D ( 'NONE', #4472, #19712, #17699 ) ;
#17577=AXIS2_PLACEMENT_3D ( 'NONE', #22968, #7740, #14080 ) ;
#17581=ADVANCED_FACE ( 'NONE', ( #15768 ), #13610, .F. ) ;
#17583=CARTESIAN_POINT ( 'NONE',  ( 119.9999999999999005, 203.2294901687515960, -100.0000000000000142 ) ) ;
#17589=ORIENTED_EDGE ( 'NONE', *, *, #15870, .T. ) ;
#17590=DIRECTION ( 'NONE',  ( 0.000000000000000000, 0.000000000000000000, 1.000000000000000000 ) ) ;
#17592=FACE_OUTER_BOUND ( 'NONE', #6720, .T. ) ;
#17596=AXIS2_PLACEMENT_3D ( 'NONE', #25585, #23441, #21285 ) ;
#17598=VECTOR ( 'NONE', #4338, 1000.000000000000000 ) ;
#17599=CARTESIAN_POINT ( 'NONE',  ( -209.7480663293921452, 74.08843928001617485, 34.98546963098892348 ) ) ;
#17606=LINE ( 'NONE', #6407, #28247 ) ;
#17609=CARTESIAN_POINT ( 'NONE',  ( -224.0127348693837916, 134.1242697789051306, 15.11921763784017969 ) ) ;
#17611=CARTESIAN_POINT ( 'NONE',  ( 97.71630809606563162, 241.5330865364753095, 11.29444388666043331 ) ) ;
#17615=DIRECTION ( 'NONE',  ( 0.000000000000000000, 0.000000000000000000, -1.000000000000000000 ) ) ;
#17631=DIRECTION ( 'NONE',  ( -1.000000000000000000, -2.602085213965211135E-16, -0.000000000000000000 ) ) ;
#17635=EDGE_CURVE ( 'NONE', #20120, #9545, #5994, .T. ) ;
#17643=VECTOR ( 'NONE', #26103, 1000.000000000000000 ) ;
#17645=VERTEX_POINT ( 'NONE', #26088 ) ;
#17651=CARTESIAN_POINT ( 'NONE',  ( -213.1074610084667142, 72.43174512725488512, 29.09741138160865503 ) ) ;
#17653=DIRECTION ( 'NONE',  ( 0.000000000000000000, 0.000000000000000000, 1.000000000000000000 ) ) ;
#17656=EDGE_CURVE ( 'NONE', #2009, #4054, #18391, .T. ) ;
#17658=CARTESIAN_POINT ( 'NONE',  ( -222.5035551981610240, 71.60080523241312278, -19.89305531471348942 ) ) ;
#17666=CARTESIAN_POINT ( 'NONE',  ( -184.0370960732481365, 107.2191430342065956, 32.03030874554431051 ) ) ;
#17667=CARTESIAN_POINT ( 'NONE',  ( -205.2903385372944172, 91.43253450480416689, -27.40388414340571188 ) ) ;
#17671=B_SPLINE_CURVE_WITH_KNOTS ( 'NONE', 3,
 ( #27237, #5829, #5548, #10150, #12177, #25371, #7845, #7577, #5693, #10289, #14185, #18622, #14463, #8130, #3526, #1518, #23220, #20638 ),
 .UNSPECIFIED., .F., .F.,
 ( 4, 2, 2, 2, 2, 2, 2, 2, 4 ),
 ( 0.000000000000000000, 0.006294660581775916169, 0.009441990872663860376, 0.01101565601810783682, 0.01258932116355180979, 0.01888398174532769994, 0.02045764689077167117, 0.02203131203621564588, 0.02517864232710359182 ),
 .UNSPECIFIED. ) ;
#17673=CARTESIAN_POINT ( 'NONE',  ( -107.9485888623679983, 135.2281170464213744, 15.33484527251397722 ) ) ;
#17675=AXIS2_PLACEMENT_3D ( 'NONE', #20904, #1225, #18747 ) ;
#17678=CARTESIAN_POINT ( 'NONE',  ( 118.4313905927012343, 122.3304618272157569, -100.0000000000000142 ) ) ;
#17682=CARTESIAN_POINT ( 'NONE',  ( -221.8871453966669378, 88.28839002355613275, 15.46908442505722014 ) ) ;
#17685=EDGE_CURVE ( 'NONE', #7854, #26801, #22053, .T. ) ;
#17693=CARTESIAN_POINT ( 'NONE',  ( -227.8378063125350366, 130.6400894613935577, -15.00000000000000178 ) ) ;
#17695=CARTESIAN_POINT ( 'NONE',  ( 115.6411010564591777, 208.5333949359988139, -99.00000000000001421 ) ) ;
#17699=DIRECTION ( 'NONE',  ( 0.000000000000000000, 0.000000000000000000, -1.000000000000000000 ) ) ;
#17700=CARTESIAN_POINT ( 'NONE',  ( -139.6220413667664388, 71.47158950552817203, 82.81269952352197095 ) ) ;
#17704=DIRECTION ( 'NONE',  ( 0.000000000000000000, 0.000000000000000000, -1.000000000000000000 ) ) ;
#17705=CARTESIAN_POINT ( 'NONE',  ( -180.4477663358212851, 109.7449299953589303, -30.47011597699462726 ) ) ;
#17712=VERTEX_POINT ( 'NONE', #24802 ) ;
#17716=EDGE_CURVE ( 'NONE', #19657, #4881, #7562, .T. ) ;
#17717=EDGE_CURVE ( 'NONE', #14427, #1808, #2307, .T. ) ;
#17723=CARTESIAN_POINT ( 'NONE',  ( -209.1829230853339254, 69.04436975541815968, -36.49242910384992200 ) ) ;
#17729=CARTESIAN_POINT ( 'NONE',  ( -146.6428522700808230, 17.24192588826928585, 80.00000000000001421 ) ) ;
#17731=CARTESIAN_POINT ( 'NONE',  ( -217.3069758534620632, 60.48634897156495782, 12.43751791598376677 ) ) ;
#17745=DIRECTION ( 'NONE',  ( 3.469446951953614189E-16, -1.000000000000000000, 0.000000000000000000 ) ) ;
#17746=ORIENTED_EDGE ( 'NONE', *, *, #16876, .F. ) ;
#17748=ORIENTED_EDGE ( 'NONE', *, *, #15398, .T. ) ;
#17750=CARTESIAN_POINT ( 'NONE',  ( -221.1044245926502754, 138.9463871349997532, 14.97905406095742364 ) ) ;
#17751=CARTESIAN_POINT ( 'NONE',  ( 90.84405255074190677, 240.0000000000000284, 6.597066685410527320 ) ) ;
#17754=VECTOR ( 'NONE', #11401, 1000.000000000000000 ) ;
#17755=AXIS2_PLACEMENT_3D ( 'NONE', #23976, #269, #13073 ) ;
#17756=CARTESIAN_POINT ( 'NONE',  ( 134.9999999999998579, 220.0000000000000284, -105.0000000000000284 ) ) ;
#17758=CARTESIAN_POINT ( 'NONE',  ( 39.99999999999995737, 59.99999999999980105, 110.0000000000000284 ) ) ;
#17761=LINE ( 'NONE', #26374, #2997 ) ;
#17763=DIRECTION ( 'NONE',  ( 0.000000000000000000, 0.000000000000000000, 1.000000000000000000 ) ) ;
#17764=CARTESIAN_POINT ( 'NONE',  ( -201.8712871270307971, 91.53752412319903442, 28.77272332722129988 ) ) ;
#17773=ORIENTED_EDGE ( 'NONE', *, *, #13635, .F. ) ;
#17776=CIRCLE ( 'NONE', #8144, 1.000000000000000888 ) ;
#17779=VERTEX_POINT ( 'NONE', #9576 ) ;
#17783=FACE_OUTER_BOUND ( 'NONE', #27081, .T. ) ;
#17788=CARTESIAN_POINT ( 'NONE',  ( -200.3909388571092052, 61.22025098964192580, 27.25552298266466167 ) ) ;
#17792=EDGE_CURVE ( 'NONE', #24488, #23655, #11046, .T. ) ;
#17793=CYLINDRICAL_SURFACE ( 'NONE', #21377, 2.000000000000000000 ) ;
#17794=AXIS2_PLACEMENT_3D ( 'NONE', #19845, #13395, #12977 ) ;
#17797=CARTESIAN_POINT ( 'NONE',  ( 100.5794065449870942, 118.1137289701970872, 81.24999999968734699 ) ) ;
#17798=CARTESIAN_POINT ( 'NONE',  ( 6.407398492414470681, 140.2478795492215227, 14.93043396175051463 ) ) ;
#17802=ORIENTED_EDGE ( 'NONE', *, *, #26001, .F. ) ;
#17803=ORIENTED_EDGE ( 'NONE', *, *, #12210, .T. ) ;
#17808=CARTESIAN_POINT ( 'NONE',  ( -206.1354706573135616, 90.30607007072229919, -28.11841259107378121 ) ) ;
#17814=VECTOR ( 'NONE', #8724, 1000.000000000000000 ) ;
#17815=DIRECTION ( 'NONE',  ( -0.000000000000000000, -0.000000000000000000, 1.000000000000000000 ) ) ;
#17819=EDGE_CURVE ( 'NONE', #23293, #1808, #938, .T. ) ;
#17821=B_SPLINE_CURVE_WITH_KNOTS ( 'NONE', 3,
 ( #27914, #28057, #10556, #5815, #9995, #5681, #16745, #10278 ),
 .UNSPECIFIED., .F., .F.,
 ( 4, 2, 2, 4 ),
 ( 3.103167691559091397E-17, 0.003477520733619440373, 0.005216281100429154272, 0.006955041467238867736 ),
 .UNSPECIFIED. ) ;
#17823=DIRECTION ( 'NONE',  ( -0.000000000000000000, -0.000000000000000000, 1.000000000000000000 ) ) ;
#17824=VERTEX_POINT ( 'NONE', #14452 ) ;
#17831=CARTESIAN_POINT ( 'NONE',  ( -211.4394172367854594, 73.16162223722503199, -31.69164223701190153 ) ) ;
#17832=AXIS2_PLACEMENT_3D ( 'NONE', #21614, #1927, #23919 ) ;
#17833=ORIENTED_EDGE ( 'NONE', *, *, #6270, .T. ) ;
#17835=CARTESIAN_POINT ( 'NONE',  ( -237.3870311360069536, 121.7710280244218950, -15.00000000000000000 ) ) ;
#17837=CARTESIAN_POINT ( 'NONE',  ( 134.9999999999998579, -327.2004514666934369, 84.99999999999995737 ) ) ;
#17838=VERTEX_POINT ( 'NONE', #8118 ) ;
#17842=CARTESIAN_POINT ( 'NONE',  ( -140.9823852843819623, 70.97022185206886036, 82.84077254739482044 ) ) ;
#17845=EDGE_CURVE ( 'NONE', #11803, #2404, #16985, .T. ) ;
#17846=EDGE_CURVE ( 'NONE', #15188, #12495, #17821, .T. ) ;
#17848=AXIS2_PLACEMENT_3D ( 'NONE', #16718, #7951, #19710 ) ;
#17852=ORIENTED_EDGE ( 'NONE', *, *, #84, .F. ) ;
#17855=DIRECTION ( 'NONE',  ( 1.000000000000000000, 4.163336342344337027E-16, 0.000000000000000000 ) ) ;
#17856=ORIENTED_EDGE ( 'NONE', *, *, #15720, .F. ) ;
#17857=VERTEX_POINT ( 'NONE', #14731 ) ;
#17858=DIRECTION ( 'NONE',  ( 0.6140342761796236948, -0.7892793597178160425, 0.000000000000000000 ) ) ;
#17861=CARTESIAN_POINT ( 'NONE',  ( 179.9999999999999147, -150.0000000000000284, -84.99999999999997158 ) ) ;
#17863=CARTESIAN_POINT ( 'NONE',  ( -28.20803558630204222, 129.1553303067010177, -16.99816387164270637 ) ) ;
#17867=ORIENTED_EDGE ( 'NONE', *, *, #16567, .T. ) ;
#17868=AXIS2_PLACEMENT_3D ( 'NONE', #21925, #13044, #11019 ) ;
#17871=CIRCLE ( 'NONE', #5482, 10.00000000000000888 ) ;
#17877=AXIS2_PLACEMENT_3D ( 'NONE', #2787, #13438, #9119 ) ;
#17882=ORIENTED_EDGE ( 'NONE', *, *, #14133, .T. ) ;
#17889=CARTESIAN_POINT ( 'NONE',  ( -209.1748869478697088, 74.44636301937694611, 36.40700551438309418 ) ) ;
#17893=EDGE_LOOP ( 'NONE', ( #1447, #1802, #24707, #4907, #25539, #5246 ) ) ;
#17898=ORIENTED_EDGE ( 'NONE', *, *, #13555, .F. ) ;
#17900=CARTESIAN_POINT ( 'NONE',  ( 101.0213870967743333, 236.0005211361349780, 23.58009545579637489 ) ) ;
#17901=CIRCLE ( 'NONE', #6882, 5.000000000000000888 ) ;
#17906=CARTESIAN_POINT ( 'NONE',  ( 32.36067977499787673, 79.99999999999998579, 100.0000000000000142 ) ) ;
#17908=DIRECTION ( 'NONE',  ( 0.000000000000000000, 0.7071067811865476838, 0.7071067811865474617 ) ) ;
#17910=DIRECTION ( 'NONE',  ( 0.000000000000000000, 0.000000000000000000, 1.000000000000000000 ) ) ;
#17911=CARTESIAN_POINT ( 'NONE',  ( 39.99999999999996447, 59.99999999999981526, 110.0000000000000284 ) ) ;
#17913=LINE ( 'NONE', #6707, #8307 ) ;
#17915=TOROIDAL_SURFACE ( 'NONE', #15632, 30.49120955644046660, 2.000000000000000000 ) ;
#17918=DIRECTION ( 'NONE',  ( 1.000000000000000000, 9.114230653120950357E-16, 0.000000000000000000 ) ) ;
#17919=ORIENTED_EDGE ( 'NONE', *, *, #22787, .T. ) ;
#17921=CARTESIAN_POINT ( 'NONE',  ( 109.1380356258695343, 251.5976846382811516, -37.70750237628016066 ) ) ;
#17924=CARTESIAN_POINT ( 'NONE',  ( -31.54599830503473257, 129.2273688777865175, -15.65862693969986097 ) ) ;
#17928=VERTEX_POINT ( 'NONE', #3514 ) ;
#17935=DIRECTION ( 'NONE',  ( 1.000000000000000000, 0.000000000000000000, 0.000000000000000000 ) ) ;
#17936=CARTESIAN_POINT ( 'NONE',  ( -7.373779444602154065, 132.9034487326637475, 14.27965191563540515 ) ) ;
#17937=ADVANCED_FACE ( 'NONE', ( #16603 ), #15177, .T. ) ;
#17938=AXIS2_PLACEMENT_3D ( 'NONE', #12098, #20839, #5752 ) ;
#17939=CARTESIAN_POINT ( 'NONE',  ( -225.1304350307098900, 62.42764488596254324, 8.801787756205932567 ) ) ;
#17948=CARTESIAN_POINT ( 'NONE',  ( 46.79174272583949090, 194.0572550123460474, 12.99999999999999822 ) ) ;
#17950=CARTESIAN_POINT ( 'NONE',  ( -175.0522400338538205, 112.5415177721608444, 28.99059681523648280 ) ) ;
#17963=ADVANCED_FACE ( 'NONE', ( #10702 ), #19598, .F. ) ;
#17964=CARTESIAN_POINT ( 'NONE',  ( 9.999999999999749534, 90.00000000000001421, 80.00000000000001421 ) ) ;
#17966=CARTESIAN_POINT ( 'NONE',  ( -142.5060805677055384, 127.4527374505125010, 16.43452876723708300 ) ) ;
#17971=ORIENTED_EDGE ( 'NONE', *, *, #11146, .F. ) ;
#17972=CARTESIAN_POINT ( 'NONE',  ( -203.8339836453408509, 92.04912517899440161, 29.52897491471929570 ) ) ;
#17974=EDGE_CURVE ( 'NONE', #20507, #12401, #10840, .T. ) ;
#17978=CIRCLE ( 'NONE', #9271, 9.999999999999994671 ) ;
#17979=CARTESIAN_POINT ( 'NONE',  ( -189.8086322075389774, 92.49158130768422836, 12.99999999999999822 ) ) ;
#17980=CARTESIAN_POINT ( 'NONE',  ( -208.5235512171359176, 74.87362916051154116, -38.25286048366049840 ) ) ;
#17982=VERTEX_POINT ( 'NONE', #349 ) ;
#17983=CARTESIAN_POINT ( 'NONE',  ( 134.9999999999998579, 220.0000000000000284, -99.00000000000001421 ) ) ;
#17986=CARTESIAN_POINT ( 'NONE',  ( 112.4999999999998863, 220.0000000000000284, 99.00000000000001421 ) ) ;
#17987=CARTESIAN_POINT ( 'NONE',  ( 134.9999999999998579, 330.0000000000000000, 84.99999999999995737 ) ) ;
#17991=CARTESIAN_POINT ( 'NONE',  ( -115.3221550338875687, 66.54464929955099706, 83.00000000000001421 ) ) ;
#17994=( BOUNDED_SURFACE ( )  B_SPLINE_SURFACE ( 2, 3, ( 
 ( #14119, #5478, #9665, #11828, #24749, #7367, #14260, #20289, #11549, #3176, #13990, #15858, #23007, #24604, #9524, #4909, #13700, #18420, #1031, #27173, #621, #2907 ),
 ( #20569, #18282, #7510, #9384, #16134, #5343, #22870, #11966, #9803, #5763, #3739, #16691, #20988, #1448, #17109, #12813, #21273, #16828, #25442, #21555, #1866, #6188 ),
 ( #23152, #12676, #25865, #10223, #1728, #4023, #3597, #14536, #23716, #8203, #19260, #12250, #27581, #1311, #10082, #19119, #23291, #21413, #25301, #12392, #28006, #12530 ) ),
 .UNSPECIFIED., .F., .F., .F. ) 
 B_SPLINE_SURFACE_WITH_KNOTS ( ( 3, 3 ),
 ( 4, 2, 2, 2, 2, 2, 2, 2, 2, 2, 4 ),
 ( 0.000000000000000000, 1.000000000000000000 ),
 ( -0.000000000000000000, 0.009354143466934852422, 0.01870828693386970484, 0.02806243040080455553, 0.03741657386773940969, 0.04677071733467426384, 0.05612486080160911106, 0.06080193253507654161, 0.06547900426854397216, 0.07015607600201140270, 0.07483314773547881937 ),
 .UNSPECIFIED. ) 
 GEOMETRIC_REPRESENTATION_ITEM ( )  RATIONAL_B_SPLINE_SURFACE ( (
 ( 1.000000000000000000, 1.000000000000000000, 1.000000000000000000, 1.000000000000000000, 1.000000000000000000, 1.000000000000000000, 1.000000000000000000, 1.000000000000000000, 1.000000000000000000, 1.000000000000000000, 1.000000000000000000, 1.000000000000000000, 1.000000000000000000, 1.000000000000000000, 1.000000000000000000, 1.000000000000000000, 1.000000000000000000, 1.000000000000000000, 1.000000000000000000, 1.000000000000000000, 1.000000000000000000, 1.000000000000000000),
 ( 0.7071067811865480168, 0.7071067811865480168, 0.7071067811865475727, 0.7071067811865475727, 0.7071067811865475727, 0.7071067811865475727, 0.7071067811865475727, 0.7071067811865475727, 0.7071067811865475727, 0.7071067811865475727, 0.7071067811865475727, 0.7071067811865475727, 0.7071067811865475727, 0.7071067811865475727, 0.7071067811865475727, 0.7071067811865475727, 0.7071067811865475727, 0.7071067811865475727, 0.7071067811865475727, 0.7071067811865475727, 0.7071067811865475727, 0.7071067811865475727),
 ( 1.000000000000000000, 1.000000000000000000, 1.000000000000000000, 1.000000000000000000, 1.000000000000000000, 1.000000000000000000, 1.000000000000000000, 1.000000000000000000, 1.000000000000000000, 1.000000000000000000, 1.000000000000000000, 1.000000000000000000, 1.000000000000000000, 1.000000000000000000, 1.000000000000000000, 1.000000000000000000, 1.000000000000000000, 1.000000000000000000, 1.000000000000000000, 1.000000000000000000, 1.000000000000000000, 1.000000000000000000) ) ) 
 REPRESENTATION_ITEM ( '' )  SURFACE ( )  );
#17997=CARTESIAN_POINT ( 'NONE',  ( -210.0000000000000000, -150.0000000000002558, -100.0000000000000142 ) ) ;
#18000=CIRCLE ( 'NONE', #20292, 22.49999999999997868 ) ;
#18002=ORIENTED_EDGE ( 'NONE', *, *, #10927, .F. ) ;
#18009=CARTESIAN_POINT ( 'NONE',  ( -20.17488871844202691, 128.4067172797072089, 17.32976398448045430 ) ) ;
#18012=CARTESIAN_POINT ( 'NONE',  ( -11.10379413178596408, 130.1809569171891212, -16.64347988244048437 ) ) ;
#18016=CARTESIAN_POINT ( 'NONE',  ( -175.0000000000000000, -120.0000000000001705, 70.00000000000001421 ) ) ;
#18018=EDGE_LOOP ( 'NONE', ( #23587, #25947, #10469, #24000 ) ) ;
#18021=DIRECTION ( 'NONE',  ( 0.000000000000000000, 0.000000000000000000, 1.000000000000000000 ) ) ;
#18022=DIRECTION ( 'NONE',  ( -1.000000000000000000, 0.000000000000000000, 0.000000000000000000 ) ) ;
#18027=ORIENTED_EDGE ( 'NONE', *, *, #24162, .F. ) ;
#18028=DIRECTION ( 'NONE',  ( -0.000000000000000000, 1.000000000000000000, -1.387778780781445429E-16 ) ) ;
#18031=VERTEX_POINT ( 'NONE', #26196 ) ;
#18033=CARTESIAN_POINT ( 'NONE',  ( 0.000000000000000000, 0.000000000000000000, 100.0000000000000142 ) ) ;
#18035=CARTESIAN_POINT ( 'NONE',  ( -222.5164088840957106, 71.60334314582038928, 19.88449668098547818 ) ) ;
#18036=ORIENTED_EDGE ( 'NONE', *, *, #27229, .F. ) ;
#18042=ORIENTED_EDGE ( 'NONE', *, *, #10579, .T. ) ;
#18044=EDGE_CURVE ( 'NONE', #26678, #10678, #18827, .T. ) ;
#18047=CIRCLE ( 'NONE', #17577, 5.000000000000004441 ) ;
#18048=CARTESIAN_POINT ( 'NONE',  ( 87.49999999999990052, 230.0000000000000000, 15.95262490344436657 ) ) ;
#18049=CARTESIAN_POINT ( 'NONE',  ( -12.24491960465745599, -23.01420295945612082, 95.00000000000000000 ) ) ;
#18051=DIRECTION ( 'NONE',  ( 0.000000000000000000, 0.000000000000000000, 1.000000000000000000 ) ) ;
#18056=DIRECTION ( 'NONE',  ( 1.000000000000000000, 3.469446951953616161E-16, 0.000000000000000000 ) ) ;
#18057=EDGE_CURVE ( 'NONE', #5833, #14725, #22966, .T. ) ;
#18061=DIRECTION ( 'NONE',  ( 0.8314772792026879911, -0.5555587585212703461, 0.000000000000000000 ) ) ;
#18066=VECTOR ( 'NONE', #6789, 1000.000000000000000 ) ;
#18067=CARTESIAN_POINT ( 'NONE',  ( 51.56615429303207065, 203.2034914284457159, 12.99999999999999822 ) ) ;
#18068=CYLINDRICAL_SURFACE ( 'NONE', #11701, 30.00000000000000000 ) ;
#18072=CARTESIAN_POINT ( 'NONE',  ( 109.8202728674371258, 257.1791079646811795, -41.57776855483199085 ) ) ;
#18079=CARTESIAN_POINT ( 'NONE',  ( -40.40953891503691153, 36.92584315232891612, 100.0000000000000000 ) ) ;
#18082=CARTESIAN_POINT ( 'NONE',  ( -175.0000000000000000, -120.0000000000001705, 63.97500000000001563 ) ) ;
#18085=CARTESIAN_POINT ( 'NONE',  ( -97.85341642296334896, 136.0957921829576378, -13.54851073784648641 ) ) ;
#18088=CARTESIAN_POINT ( 'NONE',  ( -175.0000000000000000, -120.0000000000001705, 70.00000000000001421 ) ) ;
#18089=CARTESIAN_POINT ( 'NONE',  ( -224.3698807949987497, 62.17069777284014975, 9.096889663469543308 ) ) ;
#18095=DIRECTION ( 'NONE',  ( 0.000000000000000000, -1.000000000000000000, 0.000000000000000000 ) ) ;
#18098=CARTESIAN_POINT ( 'NONE',  ( -18.00535683072674686, 129.9863796852737892, 16.68487424884472858 ) ) ;
#18102=VERTEX_POINT ( 'NONE', #26776 ) ;
#18106=LINE ( 'NONE', #13515, #14363 ) ;
#18108=CIRCLE ( 'NONE', #13535, 1.999999999999989564 ) ;
#18110=EDGE_LOOP ( 'NONE', ( #22634, #15109, #18862, #22571, #1206, #3821, #11243, #8231, #589, #12880, #19619, #4416, #25802, #6371, #1689, #2874, #4845 ) ) ;
#18112=CARTESIAN_POINT ( 'NONE',  ( -122.9556538161509991, 132.7591345059635728, 14.33728725145604699 ) ) ;
#18116=CARTESIAN_POINT ( 'NONE',  ( 79.99999999999990052, 240.0000000000000284, -45.00000000000000000 ) ) ;
#18118=DIRECTION ( 'NONE',  ( 1.000000000000000000, 0.000000000000000000, 0.000000000000000000 ) ) ;
#18125=CARTESIAN_POINT ( 'NONE',  ( 119.9999999999999432, 2.220446049250311819E-14, 90.00000000000002842 ) ) ;
#18126=CARTESIAN_POINT ( 'NONE',  ( -212.5256769160680221, 72.66764018259178215, -29.94823517518663536 ) ) ;
#18129=ADVANCED_FACE ( 'NONE', ( #22323 ), #17915, .T. ) ;
#18136=DIRECTION ( 'NONE',  ( -0.000000000000000000, -0.000000000000000000, 1.000000000000000000 ) ) ;
#18142=TOROIDAL_SURFACE ( 'NONE', #24111, 39.99999999999999289, 9.999999999999996447 ) ;
#18145=DIRECTION ( 'NONE',  ( 0.000000000000000000, 0.000000000000000000, -1.000000000000000000 ) ) ;
#18152=CARTESIAN_POINT ( 'NONE',  ( 93.99999999999985789, 171.5103103742661972, 84.99999999999995737 ) ) ;
#18153=VERTEX_POINT ( 'NONE', #639 ) ;
#18157=DIRECTION ( 'NONE',  ( 0.000000000000000000, 0.000000000000000000, 1.000000000000000000 ) ) ;
#18158=CARTESIAN_POINT ( 'NONE',  ( -24.74149867490763910, 128.0498055069775774, -17.48283640895151692 ) ) ;
#18163=CARTESIAN_POINT ( 'NONE',  ( -207.6200036923385426, 75.24376343244314569, -44.43030099895754148 ) ) ;
#18169=CARTESIAN_POINT ( 'NONE',  ( -221.1044245926312328, 138.9463871349869066, 14.97905406095859604 ) ) ;
#18171=FACE_OUTER_BOUND ( 'NONE', #21388, .T. ) ;
#18172=ORIENTED_EDGE ( 'NONE', *, *, #13682, .F. ) ;
#18173=CYLINDRICAL_SURFACE ( 'NONE', #16488, 2.000000000000005329 ) ;
#18174=ORIENTED_EDGE ( 'NONE', *, *, #10219, .T. ) ;
#18181=EDGE_CURVE ( 'NONE', #5063, #24246, #5546, .T. ) ;
#18183=EDGE_LOOP ( 'NONE', ( #6957, #25512, #28192, #18777 ) ) ;
#18188=EDGE_CURVE ( 'NONE', #16453, #23965, #5093, .T. ) ;
#18195=AXIS2_PLACEMENT_3D ( 'NONE', #6842, #19638, #99 ) ;
#18197=CARTESIAN_POINT ( 'NONE',  ( 102.7763551498688628, 237.8836077948903096, 25.40199625706859621 ) ) ;
#18199=DIRECTION ( 'NONE',  ( 0.000000000000000000, 0.000000000000000000, 1.000000000000000000 ) ) ;
#18200=DIRECTION ( 'NONE',  ( 0.000000000000000000, 0.000000000000000000, 1.000000000000000000 ) ) ;
#18203=DIRECTION ( 'NONE',  ( 0.000000000000000000, 0.000000000000000000, -1.000000000000000000 ) ) ;
#18213=FACE_OUTER_BOUND ( 'NONE', #2153, .T. ) ;
#18215=CARTESIAN_POINT ( 'NONE',  ( 49.56615429303207065, 203.2034914284457159, -15.00000000000000000 ) ) ;
#18216=EDGE_LOOP ( 'NONE', ( #9526, #18806, #22449, #18908 ) ) ;
#18218=EDGE_CURVE ( 'NONE', #12991, #23195, #16568, .T. ) ;
#18219=ORIENTED_EDGE ( 'NONE', *, *, #6558, .F. ) ;
#18225=LINE ( 'NONE', #11632, #1256 ) ;
#18226=CIRCLE ( 'NONE', #22358, 6.000000000000005329 ) ;
#18228=DIRECTION ( 'NONE',  ( 0.000000000000000000, -1.000000000000000000, 0.000000000000000000 ) ) ;
#18229=CARTESIAN_POINT ( 'NONE',  ( -101.6720583589129063, 135.8104379926313072, -13.60266426008617913 ) ) ;
#18230=DIRECTION ( 'NONE',  ( 1.000000000000000000, -0.000000000000000000, -0.000000000000000000 ) ) ;
#18231=CARTESIAN_POINT ( 'NONE',  ( -213.3516035875686896, 56.48049070729076959, 40.70111258791201436 ) ) ;
#18232=DIRECTION ( 'NONE',  ( 1.000000000000000000, 0.000000000000000000, -0.000000000000000000 ) ) ;
#18236=FACE_OUTER_BOUND ( 'NONE', #12612, .T. ) ;
#18238=CARTESIAN_POINT ( 'NONE',  ( 98.15430812615089451, 116.0637945823775112, 78.75000000031268144 ) ) ;
#18239=DIRECTION ( 'NONE',  ( -0.000000000000000000, 1.000000000000000000, -1.387778780781445429E-16 ) ) ;
#18244=VERTEX_POINT ( 'NONE', #25322 ) ;
#18245=AXIS2_PLACEMENT_3D ( 'NONE', #28124, #4141, #10619 ) ;
#18246=CYLINDRICAL_SURFACE ( 'NONE', #5029, 10.00000000000000888 ) ;
#18251=ADVANCED_FACE ( 'NONE', ( #18854 ), #10243, .F. ) ;
#18252=FACE_OUTER_BOUND ( 'NONE', #1673, .T. ) ;
#18253=CARTESIAN_POINT ( 'NONE',  ( -134.7028785880233102, 128.5088468861839601, 17.28571157459903773 ) ) ;
#18254=EDGE_CURVE ( 'NONE', #12184, #12635, #1331, .T. ) ;
#18255=ORIENTED_EDGE ( 'NONE', *, *, #25753, .T. ) ;
#18265=PLANE ( 'NONE',  #5447 ) ;
#18266=CARTESIAN_POINT ( 'NONE',  ( -207.7463451706791773, 75.42136631982602069, -41.72512927420302020 ) ) ;
#18270=CARTESIAN_POINT ( 'NONE',  ( -175.0000000000000000, -150.0000000000000853, -69.99999999999998579 ) ) ;
#18276=CARTESIAN_POINT ( 'NONE',  ( -232.3018049223844912, 76.77033509349460871, 15.55816966298073112 ) ) ;
#18280=VERTEX_POINT ( 'NONE', #27602 ) ;
#18282=CARTESIAN_POINT ( 'NONE',  ( 109.9999999986357153, 137.0808454110858463, 100.0000000001515872 ) ) ;
#18283=CARTESIAN_POINT ( 'NONE',  ( 79.99999999999991473, 140.0000000000000000, 100.0000000000000142 ) ) ;
#18287=CYLINDRICAL_SURFACE ( 'NONE', #26935, 5.000000000000004441 ) ;
#18295=DIRECTION ( 'NONE',  ( 0.000000000000000000, 0.000000000000000000, 1.000000000000000000 ) ) ;
#18297=AXIS2_PLACEMENT_3D ( 'NONE', #23027, #22612, #12128 ) ;
#18300=CARTESIAN_POINT ( 'NONE',  ( -27.05717226057298319, 127.9652800447362893, -17.51969307522723796 ) ) ;
#18301=DIRECTION ( 'NONE',  ( -1.000000000000000000, 0.000000000000000000, 0.000000000000000000 ) ) ;
#18304=DIRECTION ( 'NONE',  ( 0.000000000000000000, 0.000000000000000000, 1.000000000000000000 ) ) ;
#18307=CARTESIAN_POINT ( 'NONE',  ( -216.4421519707229606, 141.6000904446840991, 15.00000000000000000 ) ) ;
#18311=CARTESIAN_POINT ( 'NONE',  ( -160.0000000000000284, 139.9999999999999716, -45.00000000000000000 ) ) ;
#18317=CARTESIAN_POINT ( 'NONE',  ( 39.99999999999996447, 59.99999999999981526, 80.00000000000001421 ) ) ;
#18322=CIRCLE ( 'NONE', #17832, 1.000000000000000888 ) ;
#18324=CARTESIAN_POINT ( 'NONE',  ( 94.61301761981503944, 240.5205114998973670, 8.728159109110571023 ) ) ;
#18325=VERTEX_POINT ( 'NONE', #12129 ) ;
#18328=CIRCLE ( 'NONE', #16482, 30.00000000000000000 ) ;
#18329=DIRECTION ( 'NONE',  ( 0.000000000000000000, 0.000000000000000000, 1.000000000000000000 ) ) ;
#18334=CARTESIAN_POINT ( 'NONE',  ( 109.9999999999999005, 259.4346755191849070, 44.02082925133874625 ) ) ;
#18337=AXIS2_PLACEMENT_3D ( 'NONE', #3048, #13855, #20441 ) ;
#18339=EDGE_CURVE ( 'NONE', #13911, #10408, #11535, .T. ) ;
#18340=CARTESIAN_POINT ( 'NONE',  ( 107.3061218092339715, 127.3934823308176760, -87.81249999970602005 ) ) ;
#18345=DIRECTION ( 'NONE',  ( 1.000000000000000000, 0.000000000000000000, 0.000000000000000000 ) ) ;
#18348=DIRECTION ( 'NONE',  ( 1.000000000000000000, 0.000000000000000000, 0.000000000000000000 ) ) ;
#18349=ORIENTED_EDGE ( 'NONE', *, *, #18828, .T. ) ;
#18351=EDGE_CURVE ( 'NONE', #27657, #26801, #13829, .T. ) ;
#18358=LINE ( 'NONE', #24959, #601 ) ;
#18365=CARTESIAN_POINT ( 'NONE',  ( -97.95444496743660068, 136.1562174567784496, 13.53396451897430985 ) ) ;
#18366=DIRECTION ( 'NONE',  ( 0.000000000000000000, 1.000000000000000000, 0.000000000000000000 ) ) ;
#18369=CARTESIAN_POINT ( 'NONE',  ( -24.75792395070879337, 129.2472835422605897, 15.64968610871202515 ) ) ;
#18370=CARTESIAN_POINT ( 'NONE',  ( -213.7829002709373754, 55.69945581370511434, 42.78690303009008034 ) ) ;
#18372=CARTESIAN_POINT ( 'NONE',  ( -101.6645475182762226, 135.8110788931456057, -13.60253974807226029 ) ) ;
#18373=AXIS2_PLACEMENT_3D ( 'NONE', #4961, #26948, #18199 ) ;
#18374=DIRECTION ( 'NONE',  ( -0.000000000000000000, 1.000000000000000000, -0.000000000000000000 ) ) ;
#18377=LINE ( 'NONE', #25257, #2329 ) ;
#18379=CARTESIAN_POINT ( 'NONE',  ( 94.38583646782731762, 113.6320904521816857, 75.15625000028097702 ) ) ;
#18385=ORIENTED_EDGE ( 'NONE', *, *, #19238, .T. ) ;
#18391=CIRCLE ( 'NONE', #11517, 30.00000000000000000 ) ;
#18392=CARTESIAN_POINT ( 'NONE',  ( -86.54521714544338806, 134.8061557207362000, 15.45301935095626611 ) ) ;
#18396=CARTESIAN_POINT ( 'NONE',  ( 144.9999999999998863, 220.0000000000000284, 99.00000000000001421 ) ) ;
#18397=LINE ( 'NONE', #7485, #18679 ) ;
#18401=CARTESIAN_POINT ( 'NONE',  ( 92.91656858538189567, 230.8754161317235400, -17.91819948002591190 ) ) ;
#18405=CARTESIAN_POINT ( 'NONE',  ( -209.5875676835875083, 74.18578632021306873, -35.35260769160358052 ) ) ;
#18408=EDGE_CURVE ( 'NONE', #7534, #1460, #26019, .T. ) ;
#18411=DIRECTION ( 'NONE',  ( 1.000000000000000000, 0.000000000000000000, 0.000000000000000000 ) ) ;
#18413=CARTESIAN_POINT ( 'NONE',  ( 110.9201389036588949, 220.0000000000000284, -84.99999999999997158 ) ) ;
#18414=AXIS2_PLACEMENT_3D ( 'NONE', #2716, #4440, #15524 ) ;
#18415=CARTESIAN_POINT ( 'NONE',  ( -234.1955688336202854, 78.70261838805045329, 15.19002172608710843 ) ) ;
#18420=CARTESIAN_POINT ( 'NONE',  ( 85.90765579575223398, 110.5723347142863702, 70.58593750014345858 ) ) ;
#18422=ORIENTED_EDGE ( 'NONE', *, *, #21976, .F. ) ;
#18424=DIRECTION ( 'NONE',  ( 0.000000000000000000, 0.000000000000000000, 1.000000000000000000 ) ) ;
#18432=AXIS2_PLACEMENT_3D ( 'NONE', #16725, #19015, #3777 ) ;
#18435=CIRCLE ( 'NONE', #6038, 66.76834224489934400 ) ;
#18437=CARTESIAN_POINT ( 'NONE',  ( -156.2917263574996127, 178.8555734514394828, -13.00000000000000000 ) ) ;
#18439=CARTESIAN_POINT ( 'NONE',  ( -0.3773123655229073670, 134.1569627555659849, -15.55970061581417241 ) ) ;
#18448=ORIENTED_EDGE ( 'NONE', *, *, #21024, .T. ) ;
#18453=DIRECTION ( 'NONE',  ( 1.000000000000000000, 0.000000000000000000, 0.000000000000000000 ) ) ;
#18456=VERTEX_POINT ( 'NONE', #19422 ) ;
#18458=LINE ( 'NONE', #12147, #23950 ) ;
#18462=CARTESIAN_POINT ( 'NONE',  ( 101.0658546243658407, 243.3257901681003261, 15.10247091754472493 ) ) ;
#18464=EDGE_LOOP ( 'NONE', ( #195, #12694, #17517, #16794 ) ) ;
#18471=EDGE_CURVE ( 'NONE', #14063, #7534, #5005, .T. ) ;
#18474=CARTESIAN_POINT ( 'NONE',  ( -56.48697296830715686, 1.968917815184006985E-15, 100.0000000000000000 ) ) ;
#18479=CARTESIAN_POINT ( 'NONE',  ( 65.00000000000000000, -120.0000000000000711, 76.02500000000001990 ) ) ;
#18484=LINE ( 'NONE', #20914, #1973 ) ;
#18487=ADVANCED_FACE ( 'NONE', ( #18236 ), #21721, .F. ) ;
#18494=CYLINDRICAL_SURFACE ( 'NONE', #14378, 10.00000000000000888 ) ;
#18495=VERTEX_POINT ( 'NONE', #11645 ) ;
#18500=AXIS2_PLACEMENT_3D ( 'NONE', #9562, #7551, #20471 ) ;
#18503=EDGE_LOOP ( 'NONE', ( #8573, #8345, #26286, #18219 ) ) ;
#18504=ORIENTED_EDGE ( 'NONE', *, *, #17717, .T. ) ;
#18506=CARTESIAN_POINT ( 'NONE',  ( -52.43880247855167909, 133.2613159911169021, 14.19473240045777374 ) ) ;
#18508=CARTESIAN_POINT ( 'NONE',  ( -37.82257053376181233, 71.03850157808263077, 99.00000000000000000 ) ) ;
#18509=CARTESIAN_POINT ( 'NONE',  ( -42.53273978471832351, 130.9733465240572343, -14.93735646117641558 ) ) ;
#18510=CARTESIAN_POINT ( 'NONE',  ( -28.13809330698875755, 129.1551964303678801, 15.69125710151050868 ) ) ;
#18512=DIRECTION ( 'NONE',  ( 0.000000000000000000, 0.000000000000000000, 1.000000000000000000 ) ) ;
#18516=CARTESIAN_POINT ( 'NONE',  ( -17.24491960465746132, 75.97823757117562593, 95.00000000000000000 ) ) ;
#18517=DIRECTION ( 'NONE',  ( 0.000000000000000000, 0.000000000000000000, 1.000000000000000000 ) ) ;
#18523=DIRECTION ( 'NONE',  ( -0.000000000000000000, 1.000000000000000000, -1.387778780781445429E-16 ) ) ;
#18524=CARTESIAN_POINT ( 'NONE',  ( 118.9718481642231609, 125.5986290015685398, -100.0000000000000142 ) ) ;
#18526=EDGE_LOOP ( 'NONE', ( #22381, #4062, #19583, #5469 ) ) ;
#18528=CARTESIAN_POINT ( 'NONE',  ( -12.24491960465745599, 24.64876300893806160, 95.00000000000000000 ) ) ;
#18531=ORIENTED_EDGE ( 'NONE', *, *, #1946, .T. ) ;
#18532=EDGE_LOOP ( 'NONE', ( #14472, #22784, #11766, #7196 ) ) ;
#18533=CIRCLE ( 'NONE', #18976, 19.68410787789781580 ) ;
#18536=EDGE_CURVE ( 'NONE', #12559, #6913, #18377, .T. ) ;
#18542=CARTESIAN_POINT ( 'NONE',  ( 109.9999999999999005, 3.816391647148972452E-14, 25.00000000000000000 ) ) ;
#18543=DIRECTION ( 'NONE',  ( 0.000000000000000000, 0.000000000000000000, -1.000000000000000000 ) ) ;
#18545=CARTESIAN_POINT ( 'NONE',  ( -211.5579651433048411, 73.08537964810861354, -31.40200346762902939 ) ) ;
#18548=DIRECTION ( 'NONE',  ( 1.000000000000000000, 0.000000000000000000, 0.000000000000000000 ) ) ;
#18550=AXIS2_PLACEMENT_3D ( 'NONE', #17837, #11539, #6919 ) ;
#18554=CARTESIAN_POINT ( 'NONE',  ( -227.4113622183683106, 63.29489605847815881, 7.985794955240776538 ) ) ;
#18555=DIRECTION ( 'NONE',  ( 1.000000000000000000, 0.000000000000000000, -0.000000000000000000 ) ) ;
#18559=DIRECTION ( 'NONE',  ( 0.8018642810807392607, 0.5975062131282562472, 5.456026535785215050E-16 ) ) ;
#18560=CARTESIAN_POINT ( 'NONE',  ( 79.99999999999990052, 240.0000000000000284, -5.000000000000004441 ) ) ;
#18561=ORIENTED_EDGE ( 'NONE', *, *, #11115, .T. ) ;
#18568=EDGE_CURVE ( 'NONE', #9863, #13271, #24345, .T. ) ;
#18574=CARTESIAN_POINT ( 'NONE',  ( -248.1546605714623013, -91.18033988749901653, -16.91094714394370158 ) ) ;
#18580=DIRECTION ( 'NONE',  ( 1.000000000000000000, 2.602085213965211135E-16, -0.000000000000000000 ) ) ;
#18581=ORIENTED_EDGE ( 'NONE', *, *, #6350, .F. ) ;
#18588=VERTEX_POINT ( 'NONE', #7461 ) ;
#18597=CARTESIAN_POINT ( 'NONE',  ( -122.3725384480337226, 131.4093997917716763, 16.24372036387202201 ) ) ;
#18598=EDGE_LOOP ( 'NONE', ( #16022, #6440, #5871, #20291, #26188, #14367, #13154, #10418, #6972, #21066, #10726, #10973, #9775, #26020, #14446 ) ) ;
#18616=CARTESIAN_POINT ( 'NONE',  ( -160.0000000000000568, 118.4170923319166775, -21.37420696376537776 ) ) ;
#18617=CARTESIAN_POINT ( 'NONE',  ( -160.0000000000000568, 90.00000000000001421, 80.00000000000001421 ) ) ;
#18619=DIRECTION ( 'NONE',  ( 1.321694076934710155E-16, -1.000000000000000000, 0.000000000000000000 ) ) ;
#18622=CARTESIAN_POINT ( 'NONE',  ( 15.75831141662812840, 89.44692362408399333, 98.47400872637959424 ) ) ;
#18630=ADVANCED_FACE ( 'NONE', ( #3977 ), #529, .F. ) ;
#18637=ORIENTED_EDGE ( 'NONE', *, *, #10526, .F. ) ;
#18638=ORIENTED_EDGE ( 'NONE', *, *, #22065, .T. ) ;
#18644=CARTESIAN_POINT ( 'NONE',  ( -90.20499964516722002, 136.4340600182870844, -13.48772813831959283 ) ) ;
#18645=VECTOR ( 'NONE', #4168, 1000.000000000000000 ) ;
#18646=CARTESIAN_POINT ( 'NONE',  ( -107.3221550338875687, 17.24192588826928585, 83.00000000000001421 ) ) ;
#18647=CARTESIAN_POINT ( 'NONE',  ( -214.2335385402416534, 55.09354448559309958, 44.71599978583095236 ) ) ;
#18649=CARTESIAN_POINT ( 'NONE',  ( -160.0000000000000284, 109.9999999999999432, 45.00000000000000000 ) ) ;
#18650=CARTESIAN_POINT ( 'NONE',  ( 79.99999999999997158, 95.03452022453005554, -96.03494797070611355 ) ) ;
#18651=CARTESIAN_POINT ( 'NONE',  ( -217.7945318781847845, 87.80073750458967652, -17.67178672655967375 ) ) ;
#18653=DIRECTION ( 'NONE',  ( 0.000000000000000000, 0.000000000000000000, 1.000000000000000000 ) ) ;
#18657=CARTESIAN_POINT ( 'NONE',  ( -39.33244318694370634, -19.07742562058452052, 99.88564812209577326 ) ) ;
#18658=DIRECTION ( 'NONE',  ( 0.000000000000000000, 0.000000000000000000, 1.000000000000000000 ) ) ;
#18670=CARTESIAN_POINT ( 'NONE',  ( -160.0000000000000284, 119.7660240611718905, -22.85081902853004721 ) ) ;
#18675=CARTESIAN_POINT ( 'NONE',  ( 103.3065774809911090, 238.5579845772719239, -26.03670454253122557 ) ) ;
#18676=LINE ( 'NONE', #27422, #21561 ) ;
#18679=VECTOR ( 'NONE', #24286, 1000.000000000000000 ) ;
#18680=CARTESIAN_POINT ( 'NONE',  ( -207.6571795319446210, 75.48633125953863043, -42.38064732172073690 ) ) ;
#18689=ADVANCED_FACE ( 'NONE', ( #4265 ), #8319, .T. ) ;
#18691=VERTEX_POINT ( 'NONE', #19500 ) ;
#18699=VERTEX_POINT ( 'NONE', #14630 ) ;
#18700=VECTOR ( 'NONE', #16634, 1000.000000000000000 ) ;
#18701=ORIENTED_EDGE ( 'NONE', *, *, #26246, .F. ) ;
#18703=CARTESIAN_POINT ( 'NONE',  ( 92.91655173479981045, 230.8754105999472301, 17.91819147207310792 ) ) ;
#18705=ORIENTED_EDGE ( 'NONE', *, *, #8022, .T. ) ;
#18706=EDGE_CURVE ( 'NONE', #10815, #3825, #27566, .T. ) ;
#18709=DIRECTION ( 'NONE',  ( -0.000000000000000000, -0.000000000000000000, 1.000000000000000000 ) ) ;
#18711=CARTESIAN_POINT ( 'NONE',  ( 119.9999999999999147, 140.0000000000000000, -100.0000000000000142 ) ) ;
#18715=CARTESIAN_POINT ( 'NONE',  ( -203.2481855153402250, 92.57460631283319685, -29.78692811926998729 ) ) ;
#18718=DIRECTION ( 'NONE',  ( 0.9960550913260672878, 1.086714821493799823E-17, 0.08873699929240111417 ) ) ;
#18724=EDGE_CURVE ( 'NONE', #7779, #19503, #17477, .T. ) ;
#18728=CYLINDRICAL_SURFACE ( 'NONE', #21248, 5.000000000000004441 ) ;
#18730=CARTESIAN_POINT ( 'NONE',  ( -273.6211430000234373, -91.18033988749901653, 14.64217782292691261 ) ) ;
#18731=ORIENTED_EDGE ( 'NONE', *, *, #3963, .T. ) ;
#18735=AXIS2_PLACEMENT_3D ( 'NONE', #1519, #3243, #10151 ) ;
#18736=CARTESIAN_POINT ( 'NONE',  ( 109.9737507963278773, 258.9420169438926678, 43.16738424200269719 ) ) ;
#18738=ORIENTED_EDGE ( 'NONE', *, *, #757, .T. ) ;
#18740=ORIENTED_EDGE ( 'NONE', *, *, #24717, .F. ) ;
#18743=VERTEX_POINT ( 'NONE', #24371 ) ;
#18746=EDGE_CURVE ( 'NONE', #12495, #11481, #18872, .T. ) ;
#18747=DIRECTION ( 'NONE',  ( 1.000000000000000000, 2.312964634635742957E-16, 0.000000000000000000 ) ) ;
#18749=DIRECTION ( 'NONE',  ( 1.000000000000000000, -0.000000000000000000, -0.000000000000000000 ) ) ;
#18750=CYLINDRICAL_SURFACE ( 'NONE', #27775, 10.00000000000000888 ) ;
#18753=DIRECTION ( 'NONE',  ( -1.000000000000000000, 0.000000000000000000, 0.000000000000000000 ) ) ;
#18755=DIRECTION ( 'NONE',  ( -0.9611633748070274041, -0.2759800118297804916, -0.000000000000000000 ) ) ;
#18757=CARTESIAN_POINT ( 'NONE',  ( -217.2892621185082760, 109.4029876883478352, -15.00000000000000000 ) ) ;
#18758=EDGE_LOOP ( 'NONE', ( #11296, #17186 ) ) ;
#18760=CARTESIAN_POINT ( 'NONE',  ( -8.284241264067754074, 132.5788630569019233, 15.89734390185955171 ) ) ;
#18763=CIRCLE ( 'NONE', #10052, 30.00000000000000355 ) ;
#18764=FACE_OUTER_BOUND ( 'NONE', #26424, .T. ) ;
#18768=ORIENTED_EDGE ( 'NONE', *, *, #28086, .F. ) ;
#18769=AXIS2_PLACEMENT_3D ( 'NONE', #5488, #25308, #16557 ) ;
#18777=ORIENTED_EDGE ( 'NONE', *, *, #17716, .T. ) ;
#18779=CARTESIAN_POINT ( 'NONE',  ( 114.1093725872595854, 228.3710704777231797, 98.08429852854952458 ) ) ;
#18782=CIRCLE ( 'NONE', #6392, 6.000000000000005329 ) ;
#18783=CARTESIAN_POINT ( 'NONE',  ( -148.7315380569646379, 124.1728174158764517, -19.50986539812211618 ) ) ;
#18784=AXIS2_PLACEMENT_3D ( 'NONE', #12085, #5319, #16529 ) ;
#18787=EDGE_CURVE ( 'NONE', #11545, #13481, #22365, .T. ) ;
#18790=CARTESIAN_POINT ( 'NONE',  ( -207.6837665628285663, 89.33788410654877055, 27.01424684382055830 ) ) ;
#18794=ORIENTED_EDGE ( 'NONE', *, *, #12535, .T. ) ;
#18795=AXIS2_PLACEMENT_3D ( 'NONE', #1858, #23854, #15528 ) ;
#18797=CARTESIAN_POINT ( 'NONE',  ( -34.12965183067004205, -18.01420295945611727, 100.0000000000000000 ) ) ;
#18799=VERTEX_POINT ( 'NONE', #9295 ) ;
#18806=ORIENTED_EDGE ( 'NONE', *, *, #11591, .T. ) ;
#18807=EDGE_LOOP ( 'NONE', ( #19017, #26261, #8202, #2652 ) ) ;
#18810=CARTESIAN_POINT ( 'NONE',  ( 33.10302365956999182, 203.2034914284457159, 12.99999999999999822 ) ) ;
#18813=CARTESIAN_POINT ( 'NONE',  ( 109.8052436612091469, 255.9788950837981645, -41.51592141934425229 ) ) ;
#18817=DIRECTION ( 'NONE',  ( 0.000000000000000000, 0.000000000000000000, 1.000000000000000000 ) ) ;
#18819=CARTESIAN_POINT ( 'NONE',  ( -214.2384622483376688, 55.08766841006207926, -45.11431866370089239 ) ) ;
#18821=CARTESIAN_POINT ( 'NONE',  ( -17.24491960465745777, 0.000000000000000000, 95.00000000000000000 ) ) ;
#18824=VERTEX_POINT ( 'NONE', #9007 ) ;
#18825=CARTESIAN_POINT ( 'NONE',  ( -196.7149000058354602, 98.38617570187021499, 31.27679534840562781 ) ) ;
#18827=CIRCLE ( 'NONE', #26612, 5.000000000000004441 ) ;
#18828=EDGE_CURVE ( 'NONE', #1725, #16686, #24367, .T. ) ;
#18829=DIRECTION ( 'NONE',  ( 0.000000000000000000, 1.000000000000000000, 0.000000000000000000 ) ) ;
#18836=DIRECTION ( 'NONE',  ( -0.000000000000000000, -0.000000000000000000, -1.000000000000000000 ) ) ;
#18837=ORIENTED_EDGE ( 'NONE', *, *, #2155, .F. ) ;
#18839=EDGE_CURVE ( 'NONE', #8538, #2906, #993, .T. ) ;
#18842=CARTESIAN_POINT ( 'NONE',  ( -146.6428522700808230, 17.24192588826928585, 80.00000000000001421 ) ) ;
#18846=ORIENTED_EDGE ( 'NONE', *, *, #3152, .T. ) ;
#18847=CARTESIAN_POINT ( 'NONE',  ( -63.57415822541634043, 29.64876300893806516, 100.0000000000000000 ) ) ;
#18848=AXIS2_PLACEMENT_3D ( 'NONE', #11565, #22467, #25049 ) ;
#18854=FACE_OUTER_BOUND ( 'NONE', #7106, .T. ) ;
#18855=CIRCLE ( 'NONE', #26191, 10.70611877156249214 ) ;
#18858=CARTESIAN_POINT ( 'NONE',  ( 134.9999999999998579, -150.0000000000000284, 84.99999999999995737 ) ) ;
#18862=ORIENTED_EDGE ( 'NONE', *, *, #27579, .F. ) ;
#18871=ORIENTED_EDGE ( 'NONE', *, *, #12122, .T. ) ;
#18872=CIRCLE ( 'NONE', #6483, 22.49999999999997868 ) ;
#18881=VERTEX_POINT ( 'NONE', #20057 ) ;
#18882=ORIENTED_EDGE ( 'NONE', *, *, #8931, .F. ) ;
#18883=AXIS2_PLACEMENT_3D ( 'NONE', #7096, #9404, #777 ) ;
#18886=CARTESIAN_POINT ( 'NONE',  ( 109.9999999999998863, 330.0000000000000000, 100.0000000000000142 ) ) ;
#18888=CARTESIAN_POINT ( 'NONE',  ( -71.37541315349507443, 150.2892445414773590, -5.000000000000004441 ) ) ;
#18889=B_SPLINE_CURVE_WITH_KNOTS ( 'NONE', 3,
 ( #9852, #20760, #14172, #24512, #16049, #24655, #4820, #20485, #26809 ),
 .UNSPECIFIED., .F., .F.,
 ( 4, 2, 1, 2, 4 ),
 ( 0.000000000000000000, 0.003993085574633946713, 0.007986171149267893427, 0.01197925672390184014, 0.01597234229853578685 ),
 .UNSPECIFIED. ) ;
#18892=DIRECTION ( 'NONE',  ( -0.000000000000000000, -0.000000000000000000, -1.000000000000000000 ) ) ;
#18893=CIRCLE ( 'NONE', #2374, 19.07743405327024888 ) ;
#18896=AXIS2_PLACEMENT_3D ( 'NONE', #24178, #13267, #22016 ) ;
#18902=CARTESIAN_POINT ( 'NONE',  ( 109.3254858558567122, 254.7367570746976639, -35.86634952330716430 ) ) ;
#18904=CARTESIAN_POINT ( 'NONE',  ( 134.9999999999998579, 220.0000000000000284, -99.00000000000001421 ) ) ;
#18908=ORIENTED_EDGE ( 'NONE', *, *, #8250, .F. ) ;
#18909=EDGE_CURVE ( 'NONE', #19721, #18983, #16139, .T. ) ;
#18914=CARTESIAN_POINT ( 'NONE',  ( -42.53273978471833061, 130.9733465240572343, 14.93735646117641913 ) ) ;
#18915=CIRCLE ( 'NONE', #14802, 16.36034929305424512 ) ;
#18919=AXIS2_PLACEMENT_3D ( 'NONE', #9292, #2521, #18056 ) ;
#18921=DIRECTION ( 'NONE',  ( 0.000000000000000000, -0.000000000000000000, 1.000000000000000000 ) ) ;
#18922=DIRECTION ( 'NONE',  ( 1.000000000000000000, 0.000000000000000000, 0.000000000000000000 ) ) ;
#18923=EDGE_CURVE ( 'NONE', #1393, #2012, #17026, .T. ) ;
#18926=EDGE_CURVE ( 'NONE', #14569, #10474, #22932, .T. ) ;
#18927=CARTESIAN_POINT ( 'NONE',  ( -137.3782106177114883, 129.0617887715208951, -17.02469355150050845 ) ) ;
#18928=DIRECTION ( 'NONE',  ( 0.000000000000000000, -1.000000000000000000, 0.000000000000000000 ) ) ;
#18929=CARTESIAN_POINT ( 'NONE',  ( -63.57415822541634043, 75.97823757117562593, 95.00000000000000000 ) ) ;
#18932=CARTESIAN_POINT ( 'NONE',  ( -107.3221550338875687, 69.54464929955099706, 83.00000000000001421 ) ) ;
#18934=FACE_OUTER_BOUND ( 'NONE', #5862, .T. ) ;
#18938=CIRCLE ( 'NONE', #4715, 2.000000000000000000 ) ;
#18941=AXIS2_PLACEMENT_3D ( 'NONE', #3516, #14175, #20488 ) ;
#18942=ORIENTED_EDGE ( 'NONE', *, *, #4470, .F. ) ;
#18951=VERTEX_POINT ( 'NONE', #18617 ) ;
#18953=ORIENTED_EDGE ( 'NONE', *, *, #26759, .T. ) ;
#18956=TOROIDAL_SURFACE ( 'NONE', #23086, 23.59849023212046859, 2.000000000000000000 ) ;
#18960=CARTESIAN_POINT ( 'NONE',  ( 109.9878487949967791, 258.9938397943334962, -44.12861322695685118 ) ) ;
#18961=CARTESIAN_POINT ( 'NONE',  ( -3.658769994963756211, 132.7364076050659492, -15.88886450207448853 ) ) ;
#18966=CYLINDRICAL_SURFACE ( 'NONE', #7754, 5.000000000000004441 ) ;
#18968=DIRECTION ( 'NONE',  ( -1.000000000000000000, 0.000000000000000000, 0.000000000000000000 ) ) ;
#18970=AXIS2_PLACEMENT_3D ( 'NONE', #17259, #19274, #28019 ) ;
#18974=ORIENTED_EDGE ( 'NONE', *, *, #6976, .F. ) ;
#18976=AXIS2_PLACEMENT_3D ( 'NONE', #10145, #14180, #20634 ) ;
#18977=VERTEX_POINT ( 'NONE', #16056 ) ;
#18978=VERTEX_POINT ( 'NONE', #24947 ) ;
#18983=VERTEX_POINT ( 'NONE', #16471 ) ;
#18985=CARTESIAN_POINT ( 'NONE',  ( 109.8052321039920685, 255.9787816365463016, 41.51582300832603067 ) ) ;
#18988=DIRECTION ( 'NONE',  ( 1.321694076934710155E-16, -1.000000000000000000, 0.000000000000000000 ) ) ;
#18989=ORIENTED_EDGE ( 'NONE', *, *, #25428, .F. ) ;
#18990=AXIS2_PLACEMENT_3D ( 'NONE', #18088, #16084, #22389 ) ;
#18995=DIRECTION ( 'NONE',  ( -0.8142945039115421224, -0.5804519453834706688, 0.000000000000000000 ) ) ;
#19002=CARTESIAN_POINT ( 'NONE',  ( 79.99999999999991473, 110.0000000000000142, 100.0000000000000000 ) ) ;
#19003=FACE_OUTER_BOUND ( 'NONE', #18598, .T. ) ;
#19008=DIRECTION ( 'NONE',  ( -0.000000000000000000, -0.000000000000000000, 1.000000000000000000 ) ) ;
#19011=DIRECTION ( 'NONE',  ( 1.000000000000000000, 1.530283246943720628E-16, 0.000000000000000000 ) ) ;
#19013=CARTESIAN_POINT ( 'NONE',  ( -223.7492756146818067, 88.78109556843006089, 14.68106835128092946 ) ) ;
#19015=DIRECTION ( 'NONE',  ( -1.000000000000000000, -0.000000000000000000, 0.000000000000000000 ) ) ;
#19017=ORIENTED_EDGE ( 'NONE', *, *, #19565, .T. ) ;
#19018=AXIS2_PLACEMENT_3D ( 'NONE', #25878, #27876, #8220 ) ;
#19019=FACE_OUTER_BOUND ( 'NONE', #11185, .T. ) ;
#19020=CARTESIAN_POINT ( 'NONE',  ( 109.9999999999999005, 260.0000000000000000, 45.00000000000000000 ) ) ;
#19021=VERTEX_POINT ( 'NONE', #6105 ) ;
#19022=ORIENTED_EDGE ( 'NONE', *, *, #830, .T. ) ;
#19027=DIRECTION ( 'NONE',  ( 0.000000000000000000, 0.000000000000000000, 1.000000000000000000 ) ) ;
#19034=CARTESIAN_POINT ( 'NONE',  ( -273.6211430000234373, -91.18033988749901653, 14.64217782292691261 ) ) ;
#19035=CARTESIAN_POINT ( 'NONE',  ( -231.1655399901031842, 65.02775169231905750, -6.844214734956196367 ) ) ;
#19041=ORIENTED_EDGE ( 'NONE', *, *, #24565, .T. ) ;
#19044=CARTESIAN_POINT ( 'NONE',  ( 109.5784524905024853, 255.7787112550930999, -37.67977400422613243 ) ) ;
#19048=ADVANCED_FACE ( 'NONE', ( #3807 ), #12730, .F. ) ;
#19056=AXIS2_PLACEMENT_3D ( 'NONE', #24806, #9720, #13907 ) ;
#19058=CARTESIAN_POINT ( 'NONE',  ( -97.96203580167062341, 136.1557472209292143, 13.53404630376955176 ) ) ;
#19062=DIRECTION ( 'NONE',  ( 0.000000000000000000, 0.000000000000000000, 1.000000000000000000 ) ) ;
#19063=CARTESIAN_POINT ( 'NONE',  ( -82.55893756888772828, 134.8282482779731595, -15.44913056569797050 ) ) ;
#19065=CARTESIAN_POINT ( 'NONE',  ( -12.24491960465745599, -18.01420295945611727, 100.0000000000000000 ) ) ;
#19066=EDGE_CURVE ( 'NONE', #10216, #6088, #20249, .T. ) ;
#19069=CARTESIAN_POINT ( 'NONE',  ( 17.29390901368054045, -49.11867374189763780, 98.58151313434788676 ) ) ;
#19070=CARTESIAN_POINT ( 'NONE',  ( -224.3725904250179610, 86.95501853435987982, -16.78161447753165092 ) ) ;
#19075=DIRECTION ( 'NONE',  ( -0.000000000000000000, -0.000000000000000000, 1.000000000000000000 ) ) ;
#19078=AXIS2_PLACEMENT_3D ( 'NONE', #22346, #20611, #26640 ) ;
#19080=CARTESIAN_POINT ( 'NONE',  ( -63.57415822541634043, -23.01420295945612082, 95.00000000000000000 ) ) ;
#19082=VECTOR ( 'NONE', #26846, 1000.000000000000000 ) ;
#19083=EDGE_LOOP ( 'NONE', ( #22740, #10323, #5056, #11426, #21335 ) ) ;
#19084=ORIENTED_EDGE ( 'NONE', *, *, #3536, .F. ) ;
#19087=CARTESIAN_POINT ( 'NONE',  ( 107.9865739111623242, 251.1735473298933812, -29.61538987306452952 ) ) ;
#19089=ORIENTED_EDGE ( 'NONE', *, *, #8809, .F. ) ;
#19091=ORIENTED_EDGE ( 'NONE', *, *, #28086, .T. ) ;
#19092=VERTEX_POINT ( 'NONE', #1374 ) ;
#19095=VECTOR ( 'NONE', #6754, 1000.000000000000000 ) ;
#19097=FACE_BOUND ( 'NONE', #5584, .T. ) ;
#19099=DIRECTION ( 'NONE',  ( 1.000000000000000000, 0.000000000000000000, 0.000000000000000000 ) ) ;
#19101=LINE ( 'NONE', #14656, #8475 ) ;
#19102=ADVANCED_BREP_SHAPE_REPRESENTATION ( '', ( #28156, #10637 ), #3285 ) ;
#19105=LINE ( 'NONE', #25429, #407 ) ;
#19106=CARTESIAN_POINT ( 'NONE',  ( 134.9999999999998579, 220.0000000000000284, -84.99999999999997158 ) ) ;
#19109=ORIENTED_EDGE ( 'NONE', *, *, #14841, .F. ) ;
#19110=CONICAL_SURFACE ( 'NONE', #5805, 18.91107291867258411, 0.08885387018394237668 ) ;
#19111=DIRECTION ( 'NONE',  ( -0.8516548651973804285, 0.5241030343220993704, 0.000000000000000000 ) ) ;
#19114=DIRECTION ( 'NONE',  ( -0.000000000000000000, -0.000000000000000000, 1.000000000000000000 ) ) ;
#19119=CARTESIAN_POINT ( 'NONE',  ( 96.76194576697650973, 83.89264379418858653, 100.0000000000000142 ) ) ;
#19124=CARTESIAN_POINT ( 'NONE',  ( -217.0264852877946566, -91.18033988749901653, -19.68410787789781580 ) ) ;
#19127=CARTESIAN_POINT ( 'NONE',  ( -519.6468271856125511, -175.5700023691478577, -9.184850993605147944E-16 ) ) ;
#19129=AXIS2_PLACEMENT_3D ( 'NONE', #18810, #21104, #11943 ) ;
#19131=AXIS2_PLACEMENT_3D ( 'NONE', #12613, #25388, #19062 ) ;
#19133=CARTESIAN_POINT ( 'NONE',  ( -38.16416761298290794, 129.9976787137582335, -15.32285261404498655 ) ) ;
#19138=VERTEX_POINT ( 'NONE', #15449 ) ;
#19139=DIRECTION ( 'NONE',  ( 0.000000000000000000, 0.000000000000000000, 1.000000000000000000 ) ) ;
#19143=ORIENTED_EDGE ( 'NONE', *, *, #406, .T. ) ;
#19150=( NAMED_UNIT ( * ) PLANE_ANGLE_UNIT ( ) SI_UNIT ( $, .RADIAN. ) );
#19153=CIRCLE ( 'NONE', #15501, 33.76444293738739333 ) ;
#19158=ORIENTED_EDGE ( 'NONE', *, *, #6700, .T. ) ;
#19170=EDGE_CURVE ( 'NONE', #7680, #6925, #20022, .T. ) ;
#19171=CARTESIAN_POINT ( 'NONE',  ( -225.5243807178691782, 62.25611586198358793, -19.08347035850416518 ) ) ;
#19173=CARTESIAN_POINT ( 'NONE',  ( 33.10302365956999182, 203.2034914284457159, 12.99999999999999822 ) ) ;
#19177=ORIENTED_EDGE ( 'NONE', *, *, #10039, .F. ) ;
#19181=DIRECTION ( 'NONE',  ( 1.000000000000000000, -8.326672684688676025E-16, 0.000000000000000000 ) ) ;
#19186=AXIS2_PLACEMENT_3D ( 'NONE', #24521, #11165, #20058 ) ;
#19194=ORIENTED_EDGE ( 'NONE', *, *, #27785, .F. ) ;
#19198=CARTESIAN_POINT ( 'NONE',  ( 113.5875366493125682, 213.0176248557028487, 97.68174538100568327 ) ) ;
#19206=VECTOR ( 'NONE', #498, 1000.000000000000000 ) ;
#19208=CARTESIAN_POINT ( 'NONE',  ( 25.98252322492246691, -45.47589623052219565, 99.52282825389700349 ) ) ;
#19209=CARTESIAN_POINT ( 'NONE',  ( -227.1071502729981830, 87.87580414022654907, -15.87121314882625889 ) ) ;
#19211=FACE_OUTER_BOUND ( 'NONE', #16137, .T. ) ;
#19212=AXIS2_PLACEMENT_3D ( 'NONE', #5290, #27530, #5713 ) ;
#19226=CARTESIAN_POINT ( 'NONE',  ( 91.66503723320899155, 240.0531355366297817, -6.981029948440879984 ) ) ;
#19231=AXIS2_PLACEMENT_3D ( 'NONE', #7743, #3846, #12490 ) ;
#19233=ORIENTED_EDGE ( 'NONE', *, *, #313, .T. ) ;
#19237=CARTESIAN_POINT ( 'NONE',  ( -412.2374841615667833, -120.0000000000002558, 100.0000000000000142 ) ) ;
#19238=EDGE_CURVE ( 'NONE', #2342, #22383, #18893, .T. ) ;
#19239=DIRECTION ( 'NONE',  ( 0.000000000000000000, 0.000000000000000000, -1.000000000000000000 ) ) ;
#19241=CARTESIAN_POINT ( 'NONE',  ( -17.24491960465747553, 24.64876300893806160, 100.0000000000000000 ) ) ;
#19244=LINE ( 'NONE', #21254, #27728 ) ;
#19246=CARTESIAN_POINT ( 'NONE',  ( -231.4535743690441905, 76.02244276923478594, -15.77072033396453499 ) ) ;
#19248=CARTESIAN_POINT ( 'NONE',  ( -43.02437977270766112, 129.7200458115293031, 16.81627168235288039 ) ) ;
#19250=DIRECTION ( 'NONE',  ( 1.000000000000000000, 0.000000000000000000, 0.000000000000000000 ) ) ;
#19251=DIRECTION ( 'NONE',  ( 1.000000000000000000, 0.000000000000000000, 0.000000000000000000 ) ) ;
#19253=CARTESIAN_POINT ( 'NONE',  ( -200.1276905507725985, 95.64193732372173429, 30.67736252160736399 ) ) ;
#19256=VERTEX_POINT ( 'NONE', #10846 ) ;
#19260=CARTESIAN_POINT ( 'NONE',  ( 109.6721745451680334, 96.60743919220468001, 100.0000000000000142 ) ) ;
#19263=B_SPLINE_CURVE_WITH_KNOTS ( 'NONE', 3,
 ( #25370, #14321, #14599, #19044, #18902, #3525, #27369, #7844, #5692, #21056, #20773, #12598, #16478, #12176, #1381, #14462, #10006, #7576, #21337, #7988, #10288, #1657, #22937, #12314, #14184, #20917, #1097, #23219 ),
 .UNSPECIFIED., .F., .F.,
 ( 4, 2, 2, 2, 2, 2, 2, 2, 2, 2, 2, 2, 2, 4 ),
 ( -4.016943939060031455E-05, 0.006308104419754258403, 0.01265637827889911672, 0.01900465213804397591, 0.02217878906761640637, 0.02535292599718883336, 0.03170119985633366305, 0.03487533678590611086, 0.03804947371547856561, 0.04122361064505101341, 0.04281067910983723385, 0.04439774757462346122, 0.04757188450419585352, 0.05074602143376824581 ),
 .UNSPECIFIED. ) ;
#19265=VERTEX_POINT ( 'NONE', #63 ) ;
#19266=CARTESIAN_POINT ( 'NONE',  ( 108.2273028577067322, 129.5338070840588216, -100.0000000000000142 ) ) ;
#19268=DIRECTION ( 'NONE',  ( -0.000000000000000000, 1.000000000000000000, -1.387778780781445429E-16 ) ) ;
#19271=EDGE_CURVE ( 'NONE', #22091, #20823, #9264, .T. ) ;
#19272=CARTESIAN_POINT ( 'NONE',  ( -230.9997220956770150, 90.08100258884712730, 15.10258885251132455 ) ) ;
#19273=VERTEX_POINT ( 'NONE', #26780 ) ;
#19274=DIRECTION ( 'NONE',  ( -0.000000000000000000, 1.000000000000000000, -1.387778780781445429E-16 ) ) ;
#19276=EDGE_CURVE ( 'NONE', #17217, #17245, #19481, .T. ) ;
#19288=CARTESIAN_POINT ( 'NONE',  ( -119.0030847931093518, 214.2064521616283059, -15.00000000000000000 ) ) ;
#19291=DIRECTION ( 'NONE',  ( -6.938893903907227392E-16, -1.000000000000000000, 0.000000000000000000 ) ) ;
#19294=DIRECTION ( 'NONE',  ( 1.000000000000000000, 0.000000000000000000, 0.000000000000000000 ) ) ;
#19295=ORIENTED_EDGE ( 'NONE', *, *, #17521, .T. ) ;
#19296=CYLINDRICAL_SURFACE ( 'NONE', #11584, 5.999999999999991118 ) ;
#19297=CARTESIAN_POINT ( 'NONE',  ( -178.6577177197984270, 110.8366912208841200, -29.80435504473049591 ) ) ;
#19298=EDGE_LOOP ( 'NONE', ( #8450, #18871, #4919, #24795 ) ) ;
#19301=ADVANCED_FACE ( 'NONE', ( #20594 ), #23034, .T. ) ;
#19306=EDGE_LOOP ( 'NONE', ( #14394, #5868, #27976 ) ) ;
#19311=DIRECTION ( 'NONE',  ( -0.000000000000000000, 0.000000000000000000, 1.000000000000000000 ) ) ;
#19319=DIRECTION ( 'NONE',  ( 1.000000000000000000, 0.000000000000000000, 0.000000000000000000 ) ) ;
#19326=FACE_OUTER_BOUND ( 'NONE', #3455, .T. ) ;
#19329=VERTEX_POINT ( 'NONE', #2929 ) ;
#19330=AXIS2_PLACEMENT_3D ( 'NONE', #16346, #11760, #20776 ) ;
#19331=CYLINDRICAL_SURFACE ( 'NONE', #11156, 22.49999999999999289 ) ;
#19335=VERTEX_POINT ( 'NONE', #16158 ) ;
#19338=ORIENTED_EDGE ( 'NONE', *, *, #7121, .F. ) ;
#19340=DIRECTION ( 'NONE',  ( 0.000000000000000000, 0.000000000000000000, -1.000000000000000000 ) ) ;
#19341=CARTESIAN_POINT ( 'NONE',  ( -122.3728877774221644, 131.4092382197305255, -16.24378286920686421 ) ) ;
#19342=DIRECTION ( 'NONE',  ( 0.000000000000000000, -1.000000000000000000, -0.000000000000000000 ) ) ;
#19343=CARTESIAN_POINT ( 'NONE',  ( -144.5013834658754206, 126.7803687903472820, -18.02807566880128931 ) ) ;
#19345=VECTOR ( 'NONE', #19471, 1000.000000000000000 ) ;
#19349=CARTESIAN_POINT ( 'NONE',  ( -225.8617995309101047, 89.52870790985693361, -13.92929402531509098 ) ) ;
#19351=EDGE_CURVE ( 'NONE', #17645, #18325, #2832, .T. ) ;
#19353=CARTESIAN_POINT ( 'NONE',  ( -229.0059842468561442, 88.86886271388162584, 15.45135540806963448 ) ) ;
#19360=DIRECTION ( 'NONE',  ( 0.000000000000000000, 1.000000000000000000, -1.224646799147353207E-16 ) ) ;
#19364=EDGE_CURVE ( 'NONE', #25296, #2640, #14011, .T. ) ;
#19366=CARTESIAN_POINT ( 'NONE',  ( 105.1668099567758077, 241.3986356328212821, -28.65150506302982336 ) ) ;
#19367=ORIENTED_EDGE ( 'NONE', *, *, #27028, .F. ) ;
#19374=ORIENTED_EDGE ( 'NONE', *, *, #20746, .F. ) ;
#19375=ORIENTED_EDGE ( 'NONE', *, *, #7432, .T. ) ;
#19380=VECTOR ( 'NONE', #27668, 1000.000000000000114 ) ;
#19381=DIRECTION ( 'NONE',  ( 0.000000000000000000, -1.000000000000000000, 0.000000000000000000 ) ) ;
#19385=AXIS2_PLACEMENT_3D ( 'NONE', #28275, #8619, #21399 ) ;
#19386=CARTESIAN_POINT ( 'NONE',  ( -214.3828916364065833, 175.2783111443768576, -15.00000000000000000 ) ) ;
#19394=CARTESIAN_POINT ( 'NONE',  ( -184.3146016691900684, 107.2832362814925773, 31.16566266176597821 ) ) ;
#19395=CARTESIAN_POINT ( 'NONE',  ( 134.9999999999998579, 220.0000000000000284, 90.00000000000002842 ) ) ;
#19397=SHAPE_DEFINITION_REPRESENTATION ( #8194, #24038 ) ;
#19405=CARTESIAN_POINT ( 'NONE',  ( -254.4816742664885965, 103.7585653882801182, 15.00000000000000000 ) ) ;
#19410=CARTESIAN_POINT ( 'NONE',  ( 99.60675733924797726, 85.63108538499818678, -100.0000000000000284 ) ) ;
#19412=CARTESIAN_POINT ( 'NONE',  ( 179.9999999999999147, 0.000000000000000000, -84.99999999999997158 ) ) ;
#19415=CARTESIAN_POINT ( 'NONE',  ( -212.5733778118419082, 87.16562594403421826, 23.37021847070533553 ) ) ;
#19416=ORIENTED_EDGE ( 'NONE', *, *, #11827, .T. ) ;
#19422=CARTESIAN_POINT ( 'NONE',  ( -244.5479615644635771, 75.99513337129096158, -5.000000000000004441 ) ) ;
#19424=CIRCLE ( 'NONE', #3341, 30.00000000000000000 ) ;
#19427=CARTESIAN_POINT ( 'NONE',  ( 79.99999999999994316, -100.0000000000000284, 70.00000000000001421 ) ) ;
#19431=CARTESIAN_POINT ( 'NONE',  ( 184.9999999999999432, -327.2004514666934369, 84.99999999999995737 ) ) ;
#19434=LINE ( 'NONE', #15282, #9880 ) ;
#19436=CARTESIAN_POINT ( 'NONE',  ( -146.6428522700808230, 17.24192588826928585, 83.00000000000001421 ) ) ;
#19440=CARTESIAN_POINT ( 'NONE',  ( 179.9999999999999147, 0.000000000000000000, -100.0000000000000142 ) ) ;
#19442=CARTESIAN_POINT ( 'NONE',  ( -183.8717786033620882, 107.3112658120104470, -31.96029808677420547 ) ) ;
#19455=CARTESIAN_POINT ( 'NONE',  ( 89.99999999999988631, 230.0000000000000000, 6.270166537925822681 ) ) ;
#19458=CARTESIAN_POINT ( 'NONE',  ( -243.5753208290373948, 74.80993601159312334, -14.84129168368860796 ) ) ;
#19465=VECTOR ( 'NONE', #14003, 1000.000000000000000 ) ;
#19471=DIRECTION ( 'NONE',  ( -0.000000000000000000, -1.000000000000000000, -0.000000000000000000 ) ) ;
#19476=FACE_OUTER_BOUND ( 'NONE', #27830, .T. ) ;
#19480=ORIENTED_EDGE ( 'NONE', *, *, #26431, .F. ) ;
#19481=B_SPLINE_CURVE_WITH_KNOTS ( 'NONE', 3,
 ( #13868, #25185, #27058, #1058, #24627, #18169, #11851, #12136, #18307 ),
 .UNSPECIFIED., .F., .F.,
 ( 4, 2, 1, 2, 4 ),
 ( 0.000000000000000000, 0.003993085574633965795, 0.007986171149267931590, 0.01197925672390189739, 0.01597234229853586318 ),
 .UNSPECIFIED. ) ;
#19487=DIRECTION ( 'NONE',  ( -1.000000000000000000, 0.000000000000000000, -0.000000000000000000 ) ) ;
#19488=VECTOR ( 'NONE', #18543, 1000.000000000000000 ) ;
#19489=CARTESIAN_POINT ( 'NONE',  ( -112.5606509705656464, 133.0497573896584811, -15.80384718330080140 ) ) ;
#19496=CARTESIAN_POINT ( 'NONE',  ( -231.9378824387722773, 93.53122965655592225, -14.99999999999998757 ) ) ;
#19497=DIRECTION ( 'NONE',  ( 0.000000000000000000, 0.000000000000000000, 1.000000000000000000 ) ) ;
#19498=CARTESIAN_POINT ( 'NONE',  ( 110.9201389036588949, 220.0000000000000284, 84.99999999999995737 ) ) ;
#19500=CARTESIAN_POINT ( 'NONE',  ( -175.0000000000000000, -120.0250000000001904, -63.99999999999998579 ) ) ;
#19503=VERTEX_POINT ( 'NONE', #1750 ) ;
#19512=CARTESIAN_POINT ( 'NONE',  ( 97.71630809605208867, 241.5330865364702504, -11.29444388665504562 ) ) ;
#19515=CARTESIAN_POINT ( 'NONE',  ( 79.99999999999991473, 140.0000000000000000, -45.00000000000000000 ) ) ;
#19518=ORIENTED_EDGE ( 'NONE', *, *, #20317, .T. ) ;
#19523=CARTESIAN_POINT ( 'NONE',  ( -12.24491960465745599, -18.01420295945611727, 95.00000000000000000 ) ) ;
#19525=AXIS2_PLACEMENT_3D ( 'NONE', #2060, #22174, #15300 ) ;
#19535=FACE_OUTER_BOUND ( 'NONE', #15817, .T. ) ;
#19542=CARTESIAN_POINT ( 'NONE',  ( -170.0203570005763822, 115.7187005978582590, 25.41133611931261527 ) ) ;
#19548=EDGE_LOOP ( 'NONE', ( #10335, #411, #12351, #12112 ) ) ;
#19549=EDGE_CURVE ( 'NONE', #12684, #18977, #9738, .T. ) ;
#19551=DIRECTION ( 'NONE',  ( -0.000000000000000000, 0.000000000000000000, 1.000000000000000000 ) ) ;
#19555=CARTESIAN_POINT ( 'NONE',  ( 90.92319367349371362, 112.0484670279546435, -100.0000000000000142 ) ) ;
#19556=CARTESIAN_POINT ( 'NONE',  ( -175.2983697824313083, 112.8108207344445333, -27.79681538115707085 ) ) ;
#19557=ORIENTED_EDGE ( 'NONE', *, *, #124, .F. ) ;
#19558=CARTESIAN_POINT ( 'NONE',  ( -219.2326573687354880, 87.85061497978375655, 16.80038353493895897 ) ) ;
#19559=ORIENTED_EDGE ( 'NONE', *, *, #3905, .F. ) ;
#19564=VECTOR ( 'NONE', #14578, 1000.000000000000000 ) ;
#19565=EDGE_CURVE ( 'NONE', #12401, #12426, #20712, .T. ) ;
#19574=ORIENTED_EDGE ( 'NONE', *, *, #20436, .F. ) ;
#19576=CARTESIAN_POINT ( 'NONE',  ( 79.99999999999990052, 140.0000000000000000, 45.00000000000000000 ) ) ;
#19577=CARTESIAN_POINT ( 'NONE',  ( -228.0469991721728036, 90.67060700717054544, 13.41267718625879724 ) ) ;
#19580=EDGE_LOOP ( 'NONE', ( #2057, #4627, #7103, #15474 ) ) ;
#19582=CARTESIAN_POINT ( 'NONE',  ( -169.6922851464237567, 115.8923280138696157, -26.07704740418152767 ) ) ;
#19583=ORIENTED_EDGE ( 'NONE', *, *, #6653, .T. ) ;
#19585=AXIS2_PLACEMENT_3D ( 'NONE', #23269, #1569, #25551 ) ;
#19586=ORIENTED_EDGE ( 'NONE', *, *, #15186, .T. ) ;
#19590=ORIENTED_EDGE ( 'NONE', *, *, #1286, .F. ) ;
#19592=CARTESIAN_POINT ( 'NONE',  ( -23.60339304038094710, 128.1103613223097284, 17.45643390080418911 ) ) ;
#19593=CARTESIAN_POINT ( 'NONE',  ( -225.7036482868739427, -91.18033988749901653, 18.91107291867258766 ) ) ;
#19594=CARTESIAN_POINT ( 'NONE',  ( -160.0000000000000284, 79.99999999999994316, -100.0000000000000142 ) ) ;
#19595=DIRECTION ( 'NONE',  ( 0.9682458365518546994, -0.000000000000000000, 0.2499999999999989453 ) ) ;
#19598=CYLINDRICAL_SURFACE ( 'NONE', #9205, 166.0121251338587172 ) ;
#19600=CARTESIAN_POINT ( 'NONE',  ( -225.5840809296905149, 72.49952595022725177, -18.07266724760468080 ) ) ;
#19602=DIRECTION ( 'NONE',  ( -0.5975062131282553590, 0.8018642810807399268, 0.000000000000000000 ) ) ;
#19605=CARTESIAN_POINT ( 'NONE',  ( 114.6860526936810487, 229.7243539224658093, -98.48425370696855907 ) ) ;
#19615=CARTESIAN_POINT ( 'NONE',  ( 115.6411010564592061, 231.4666050640012998, 99.00000000000001421 ) ) ;
#19616=ORIENTED_EDGE ( 'NONE', *, *, #7014, .T. ) ;
#19619=ORIENTED_EDGE ( 'NONE', *, *, #7580, .F. ) ;
#19621=CARTESIAN_POINT ( 'NONE',  ( -221.3650667873343139, -91.18033988749901653, 19.29759039828519818 ) ) ;
#19626=CARTESIAN_POINT ( 'NONE',  ( -217.6530384384126080, 140.9974917369520426, 15.00000000000000000 ) ) ;
#19627=AXIS2_PLACEMENT_3D ( 'NONE', #6869, #11771, #2550 ) ;
#19628=CARTESIAN_POINT ( 'NONE',  ( -107.6076100521348877, 133.6773311915829936, -15.67055231630294010 ) ) ;
#19630=CYLINDRICAL_SURFACE ( 'NONE', #1816, 30.00000000000002842 ) ;
#19631=EDGE_CURVE ( 'NONE', #24933, #1342, #18915, .T. ) ;
#19636=CARTESIAN_POINT ( 'NONE',  ( -212.5754918423282618, 87.16543701462498461, -23.36890611379539706 ) ) ;
#19638=DIRECTION ( 'NONE',  ( 0.000000000000000000, 1.000000000000000000, 0.000000000000000000 ) ) ;
#19639=DIRECTION ( 'NONE',  ( -0.000000000000000000, -0.000000000000000000, 1.000000000000000000 ) ) ;
#19641=CARTESIAN_POINT ( 'NONE',  ( -140.1213116003368668, 122.5384136796733827, 12.99999999999999822 ) ) ;
#19644=VECTOR ( 'NONE', #19075, 1000.000000000000000 ) ;
#19646=CARTESIAN_POINT ( 'NONE',  ( -141.6428522700808230, 22.24192588826928585, 83.00000000000001421 ) ) ;
#19649=EDGE_LOOP ( 'NONE', ( #11223, #17111, #12046, #13538 ) ) ;
#19650=CARTESIAN_POINT ( 'NONE',  ( 92.49170488791030209, 239.7529794472836215, -17.61766721977555505 ) ) ;
#19652=CARTESIAN_POINT ( 'NONE',  ( -20.35978069378271726, 129.6268764493030687, -15.48139849003159618 ) ) ;
#19657=VERTEX_POINT ( 'NONE', #24169 ) ;
#19658=ORIENTED_EDGE ( 'NONE', *, *, #7639, .F. ) ;
#19666=CARTESIAN_POINT ( 'NONE',  ( -226.0190876347067785, 72.67478414371682049, 17.85134081709900755 ) ) ;
#19668=FACE_OUTER_BOUND ( 'NONE', #26002, .T. ) ;
#19669=ADVANCED_FACE ( 'NONE', ( #13542 ), #25334, .T. ) ;
#19670=LINE ( 'NONE', #4432, #19082 ) ;
#19672=CARTESIAN_POINT ( 'NONE',  ( 79.99999999999992895, 230.0000000000000000, 5.000000000000002665 ) ) ;
#19677=CARTESIAN_POINT ( 'NONE',  ( -209.9813605129777159, 61.38896102042362912, 24.60123923356250586 ) ) ;
#19678=CARTESIAN_POINT ( 'NONE',  ( -210.0000000000000000, -150.0000000000001990, 100.0000000000000142 ) ) ;
#19682=CARTESIAN_POINT ( 'NONE',  ( -169.7566311317153236, 115.8586538395105237, 26.10480086864442839 ) ) ;
#19683=AXIS2_PLACEMENT_3D ( 'NONE', #3808, #10847, #19319 ) ;
#19686=ORIENTED_EDGE ( 'NONE', *, *, #25815, .F. ) ;
#19689=ORIENTED_EDGE ( 'NONE', *, *, #8874, .T. ) ;
#19691=DIRECTION ( 'NONE',  ( 0.000000000000000000, 0.000000000000000000, -1.000000000000000000 ) ) ;
#19693=CARTESIAN_POINT ( 'NONE',  ( 119.9999999999999147, 140.0000000000000000, -100.0000000000000142 ) ) ;
#19696=DIRECTION ( 'NONE',  ( -0.000000000000000000, -0.000000000000000000, 1.000000000000000000 ) ) ;
#19698=CARTESIAN_POINT ( 'NONE',  ( -211.8433833244381503, 88.46778497223422733, 21.92823303506064292 ) ) ;
#19710=DIRECTION ( 'NONE',  ( 1.000000000000000000, 0.000000000000000000, 0.000000000000000000 ) ) ;
#19712=DIRECTION ( 'NONE',  ( 0.000000000000000000, -1.000000000000000000, 0.000000000000000000 ) ) ;
#19713=CARTESIAN_POINT ( 'NONE',  ( -180.0000000000000284, -2.775557561562891982E-14, -100.0000000000000142 ) ) ;
#19716=ADVANCED_FACE ( 'NONE', ( #1020 ), #27295, .F. ) ;
#19717=AXIS2_PLACEMENT_3D ( 'NONE', #19746, #2353, #8274 ) ;
#19718=ADVANCED_FACE ( 'NONE', ( #7066, #7635 ), #25147, .T. ) ;
#19720=CARTESIAN_POINT ( 'NONE',  ( -186.8149004422502912, 105.6021380271806436, -32.12667098497705354 ) ) ;
#19721=VERTEX_POINT ( 'NONE', #17986 ) ;
#19723=DIRECTION ( 'NONE',  ( 0.6787614006938652578, 0.7343588774761984350, 0.000000000000000000 ) ) ;
#19725=EDGE_CURVE ( 'NONE', #17425, #16662, #21208, .T. ) ;
#19726=ORIENTED_EDGE ( 'NONE', *, *, #25863, .T. ) ;
#19728=CARTESIAN_POINT ( 'NONE',  ( -28.22105481086200385, 127.9579655952397275, 17.52291750101008105 ) ) ;
#19730=CARTESIAN_POINT ( 'NONE',  ( -160.0000000000000284, 59.99999999999994316, 70.00000000000001421 ) ) ;
#19733=DIRECTION ( 'NONE',  ( 0.000000000000000000, 0.000000000000000000, 1.000000000000000000 ) ) ;
#19735=CIRCLE ( 'NONE', #27085, 19.68410787789781580 ) ;
#19746=CARTESIAN_POINT ( 'NONE',  ( -63.57415822541634043, 75.97823757117562593, 95.00000000000000000 ) ) ;
#19753=ORIENTED_EDGE ( 'NONE', *, *, #508, .T. ) ;
#19755=VERTEX_POINT ( 'NONE', #3027 ) ;
#19756=EDGE_CURVE ( 'NONE', #7140, #27404, #2393, .T. ) ;
#19762=ORIENTED_EDGE ( 'NONE', *, *, #21141, .T. ) ;
#19764=CARTESIAN_POINT ( 'NONE',  ( -225.9729034214342676, 132.4331356209129638, 12.99353264123212526 ) ) ;
#19765=CARTESIAN_POINT ( 'NONE',  ( 96.93828241645127264, 232.7455409703985936, 20.22303902613926851 ) ) ;
#19773=FACE_OUTER_BOUND ( 'NONE', #13038, .T. ) ;
#19782=DIRECTION ( 'NONE',  ( 0.000000000000000000, -0.000000000000000000, -1.000000000000000000 ) ) ;
#19783=DIRECTION ( 'NONE',  ( -0.000000000000000000, -0.000000000000000000, -1.000000000000000000 ) ) ;
#19784=ORIENTED_EDGE ( 'NONE', *, *, #5128, .T. ) ;
#19787=CARTESIAN_POINT ( 'NONE',  ( -7.443569385156187046, 132.8772577174391643, -14.28756630290005525 ) ) ;
#19788=ORIENTED_EDGE ( 'NONE', *, *, #866, .T. ) ;
#19795=VERTEX_POINT ( 'NONE', #14108 ) ;
#19798=AXIS2_PLACEMENT_3D ( 'NONE', #3071, #9270, #13879 ) ;
#19800=AXIS2_PLACEMENT_3D ( 'NONE', #3985, #25825, #12491 ) ;
#19802=UNCERTAINTY_MEASURE_WITH_UNIT (LENGTH_MEASURE( 1.000000000000000082E-05 ), #6958, 'distance_accuracy_value', 'NONE');
#19803=DIRECTION ( 'NONE',  ( 0.000000000000000000, 0.000000000000000000, -1.000000000000000000 ) ) ;
#19804=CARTESIAN_POINT ( 'NONE',  ( -220.9458266506729842, 71.36862438102525630, 20.99673689147903843 ) ) ;
#19807=DIRECTION ( 'NONE',  ( -0.8018642810807398158, -0.5975062131282554700, 0.000000000000000000 ) ) ;
#19808=DIRECTION ( 'NONE',  ( 0.000000000000000000, 0.000000000000000000, -1.000000000000000000 ) ) ;
#19810=CARTESIAN_POINT ( 'NONE',  ( 33.10302365956999182, 221.6666220619077876, 15.00000000000000000 ) ) ;
#19812=CARTESIAN_POINT ( 'NONE',  ( -40.77177304839534600, 129.1844851112595904, 17.01161629403331688 ) ) ;
#19813=CARTESIAN_POINT ( 'NONE',  ( -209.9947863080667787, 60.75003584150559988, 22.65371792907697568 ) ) ;
#19816=VECTOR ( 'NONE', #21310, 1000.000000000000000 ) ;
#19817=ORIENTED_EDGE ( 'NONE', *, *, #1538, .F. ) ;
#19819=CARTESIAN_POINT ( 'NONE',  ( -175.1909440597360117, 112.8732459110917006, 28.42595730244120134 ) ) ;
#19822=ADVANCED_FACE ( 'NONE', ( #1300 ), #6177, .F. ) ;
#19823=CARTESIAN_POINT ( 'NONE',  ( -205.5903157496420022, 91.23080130178013292, -28.02187135762362757 ) ) ;
#19824=ORIENTED_EDGE ( 'NONE', *, *, #22541, .T. ) ;
#19829=CARTESIAN_POINT ( 'NONE',  ( -113.0182548846454011, 134.5412002400303209, 13.86291542401011156 ) ) ;
#19833=VECTOR ( 'NONE', #17855, 1000.000000000000000 ) ;
#19834=CARTESIAN_POINT ( 'NONE',  ( 100.8904249506145874, 86.57652225509636423, -100.0000000000000142 ) ) ;
#19837=VERTEX_POINT ( 'NONE', #6032 ) ;
#19838=CARTESIAN_POINT ( 'NONE',  ( -224.3954463207928711, 86.96133147683917741, 16.77313708869839104 ) ) ;
#19839=AXIS2_PLACEMENT_3D ( 'NONE', #9997, #11749, #22793 ) ;
#19841=AXIS2_PLACEMENT_3D ( 'NONE', #5726, #859, #14503 ) ;
#19845=CARTESIAN_POINT ( 'NONE',  ( -270.1025481742786951, -91.18033988749901653, 0.000000000000000000 ) ) ;
#19850=CIRCLE ( 'NONE', #11120, 30.00000000000002842 ) ;
#19855=CARTESIAN_POINT ( 'NONE',  ( -160.0000000000000568, 230.0000000000000000, -15.00000000000000000 ) ) ;
#19858=AXIS2_PLACEMENT_3D ( 'NONE', #9619, #2996, #13946 ) ;
#19861=CARTESIAN_POINT ( 'NONE',  ( -196.6299573648443868, 98.19963181860228474, -32.16283524453812959 ) ) ;
#19863=ORIENTED_EDGE ( 'NONE', *, *, #19351, .F. ) ;
#19867=EDGE_LOOP ( 'NONE', ( #13873, #16514, #12047, #6611 ) ) ;
#19869=AXIS2_PLACEMENT_3D ( 'NONE', #26611, #17572, #26331 ) ;
#19870=CARTESIAN_POINT ( 'NONE',  ( 134.9999999999998579, 220.0000000000000284, -100.0000000000000142 ) ) ;
#19879=SPHERICAL_SURFACE ( 'NONE', #26567, 5.000000000000000000 ) ;
#19881=ADVANCED_FACE ( 'NONE', ( #3586 ), #10203, .T. ) ;
#19882=CARTESIAN_POINT ( 'NONE',  ( -68.57415822541635464, -18.01420295945611727, 95.00000000000000000 ) ) ;
#19884=CARTESIAN_POINT ( 'NONE',  ( 79.99999999999994316, 80.00000000000001421, 100.0000000000000142 ) ) ;
#19888=ORIENTED_EDGE ( 'NONE', *, *, #7646, .F. ) ;
#19891=CARTESIAN_POINT ( 'NONE',  ( -221.9128906662286340, 61.41899577391678378, -10.11264670733106463 ) ) ;
#19896=TOROIDAL_SURFACE ( 'NONE', #6520, 11.00000000000001066, 1.000000000000000000 ) ;
#19902=ORIENTED_EDGE ( 'NONE', *, *, #10522, .T. ) ;
#19905=ADVANCED_FACE ( 'NONE', ( #7773 ), #21118, .F. ) ;
#19908=CARTESIAN_POINT ( 'NONE',  ( -227.3657730843038109, 133.9833936510421211, 14.99191580167116733 ) ) ;
#19909=CARTESIAN_POINT ( 'NONE',  ( 103.7569845406553668, 245.1294976011697884, 26.47883977338666739 ) ) ;
#19914=DIRECTION ( 'NONE',  ( 1.000000000000000000, 0.000000000000000000, 0.000000000000000000 ) ) ;
#19916=CARTESIAN_POINT ( 'NONE',  ( -63.57415822541634043, 75.97823757117562593, 100.0000000000000000 ) ) ;
#19917=DIRECTION ( 'NONE',  ( -0.000000000000000000, -0.000000000000000000, 1.000000000000000000 ) ) ;
#19919=DIRECTION ( 'NONE',  ( -1.000000000000000000, 0.000000000000000000, 0.000000000000000000 ) ) ;
#19922=EDGE_CURVE ( 'NONE', #17211, #26118, #1481, .T. ) ;
#19925=EDGE_CURVE ( 'NONE', #25545, #6472, #17534, .T. ) ;
#19926=CARTESIAN_POINT ( 'NONE',  ( 109.9999999999999147, 140.0000000000000000, 90.00000000000002842 ) ) ;
#19929=LINE ( 'NONE', #9017, #26665 ) ;
#19935=CIRCLE ( 'NONE', #9853, 1.999999999999989564 ) ;
#19936=ORIENTED_EDGE ( 'NONE', *, *, #5364, .F. ) ;
#19940=AXIS2_PLACEMENT_3D ( 'NONE', #16204, #255, #9452 ) ;
#19941=ORIENTED_EDGE ( 'NONE', *, *, #804, .F. ) ;
#19945=CARTESIAN_POINT ( 'NONE',  ( 0.000000000000000000, 75.97823757117562593, 95.00000000000000000 ) ) ;
#19947=CARTESIAN_POINT ( 'NONE',  ( -209.7310389751728508, 59.98715598645322444, 17.47553936828792587 ) ) ;
#19958=CARTESIAN_POINT ( 'NONE',  ( -8.311916932730307295, 131.0476075684319994, 16.36633293656888810 ) ) ;
#19962=ORIENTED_EDGE ( 'NONE', *, *, #24395, .F. ) ;
#19964=CARTESIAN_POINT ( 'NONE',  ( -161.8971216350977329, 118.9700043538931737, 23.57800815686201190 ) ) ;
#19966=DIRECTION ( 'NONE',  ( 0.000000000000000000, -1.000000000000000000, 0.000000000000000000 ) ) ;
#19973=ORIENTED_EDGE ( 'NONE', *, *, #8286, .F. ) ;
#19975=AXIS2_PLACEMENT_3D ( 'NONE', #3657, #4079, #14732 ) ;
#19978=CARTESIAN_POINT ( 'NONE',  ( -201.5823348103256478, 94.41654411267251135, -29.50230888136551854 ) ) ;
#19980=CARTESIAN_POINT ( 'NONE',  ( -207.8757358334619312, 89.94749888897153767, 26.37785067087564883 ) ) ;
#19981=CIRCLE ( 'NONE', #5743, 60.59270260175150469 ) ;
#19982=CARTESIAN_POINT ( 'NONE',  ( 39.99999999999995737, 59.99999999999980105, 80.00000000000001421 ) ) ;
#19985=ADVANCED_FACE ( 'NONE', ( #12800 ), #20758, .F. ) ;
#19991=DIRECTION ( 'NONE',  ( -1.000000000000000000, 0.000000000000000000, 0.000000000000000000 ) ) ;
#19995=PLANE ( 'NONE',  #5458 ) ;
#19997=DIRECTION ( 'NONE',  ( -0.000000000000000000, 1.000000000000000000, -1.387778780781445429E-16 ) ) ;
#20002=CARTESIAN_POINT ( 'NONE',  ( -202.4550896089758112, 93.28604070817037552, -30.13616383332644588 ) ) ;
#20004=VERTEX_POINT ( 'NONE', #13089 ) ;
#20008=EDGE_LOOP ( 'NONE', ( #7804, #26675, #22520, #18740 ) ) ;
#20009=CIRCLE ( 'NONE', #27797, 22.49999999999999289 ) ;
#20010=DIRECTION ( 'NONE',  ( -0.000000000000000000, 1.000000000000000000, -1.387778780781445429E-16 ) ) ;
#20012=DIRECTION ( 'NONE',  ( -0.000000000000000000, -0.000000000000000000, 1.000000000000000000 ) ) ;
#20014=CARTESIAN_POINT ( 'NONE',  ( -8.492276074956963683, 132.4970898450557399, -14.40628465233269218 ) ) ;
#20016=CARTESIAN_POINT ( 'NONE',  ( -119.0030847931093518, 214.2064521616282775, 15.00000000000000000 ) ) ;
#20022=LINE ( 'NONE', #4642, #10629 ) ;
#20028=ADVANCED_FACE ( 'NONE', ( #4012 ), #12067, .T. ) ;
#20029=DIRECTION ( 'NONE',  ( -0.000000000000000000, -0.000000000000000000, 1.000000000000000000 ) ) ;
#20031=FACE_OUTER_BOUND ( 'NONE', #10515, .T. ) ;
#20037=VERTEX_POINT ( 'NONE', #22116 ) ;
#20039=VERTEX_POINT ( 'NONE', #1856 ) ;
#20040=ADVANCED_FACE ( 'NONE', ( #10918 ), #27196, .T. ) ;
#20041=ORIENTED_EDGE ( 'NONE', *, *, #11827, .F. ) ;
#20046=CARTESIAN_POINT ( 'NONE',  ( 88.62124187924879948, 239.8086506234586750, 16.24979138471424989 ) ) ;
#20050=VECTOR ( 'NONE', #13672, 1000.000000000000000 ) ;
#20054=CARTESIAN_POINT ( 'NONE',  ( 9.999999999999964473, 60.00000000000001421, 110.0000000000000284 ) ) ;
#20057=CARTESIAN_POINT ( 'NONE',  ( -37.82257053376181233, 71.03850157808263077, 100.0000000000000000 ) ) ;
#20058=DIRECTION ( 'NONE',  ( 1.000000000000000000, 0.000000000000000000, 0.000000000000000000 ) ) ;
#20062=EDGE_CURVE ( 'NONE', #10685, #5551, #11150, .T. ) ;
#20069=CARTESIAN_POINT ( 'NONE',  ( -112.3221550338875687, 74.54464929955099706, 83.00000000000001421 ) ) ;
#20074=ORIENTED_EDGE ( 'NONE', *, *, #21247, .T. ) ;
#20079=EDGE_LOOP ( 'NONE', ( #20365, #23017, #26719, #25867 ) ) ;
#20080=FACE_OUTER_BOUND ( 'NONE', #19580, .T. ) ;
#20087=CARTESIAN_POINT ( 'NONE',  ( -222.4720504096164007, 61.14635810690615614, 21.27434031932121172 ) ) ;
#20090=DIRECTION ( 'NONE',  ( -0.000000000000000000, -0.000000000000000000, -1.000000000000000000 ) ) ;
#20095=LINE ( 'NONE', #3130, #13216 ) ;
#20097=CARTESIAN_POINT ( 'NONE',  ( -4.127814339125048804, 134.2316681395303988, 15.51991914718412779 ) ) ;
#20098=DIRECTION ( 'NONE',  ( 0.000000000000000000, 0.000000000000000000, 1.000000000000000000 ) ) ;
#20104=AXIS2_PLACEMENT_3D ( 'NONE', #26527, #9023, #4695 ) ;
#20107=VERTEX_POINT ( 'NONE', #15525 ) ;
#20109=ORIENTED_EDGE ( 'NONE', *, *, #22259, .F. ) ;
#20111=AXIS2_PLACEMENT_3D ( 'NONE', #4828, #17763, #682 ) ;
#20120=VERTEX_POINT ( 'NONE', #9487 ) ;
#20121=CARTESIAN_POINT ( 'NONE',  ( -206.1571879782320309, 90.87865330178034640, 27.62915181265775644 ) ) ;
#20124=DIRECTION ( 'NONE',  ( -0.000000000000000000, -0.000000000000000000, 1.000000000000000000 ) ) ;
#20125=DIRECTION ( 'NONE',  ( 0.000000000000000000, 1.000000000000000000, 0.000000000000000000 ) ) ;
#20126=CARTESIAN_POINT ( 'NONE',  ( -217.4092282431682577, 59.59925738963638508, -26.62835594396155869 ) ) ;
#20127=ORIENTED_EDGE ( 'NONE', *, *, #4707, .T. ) ;
#20128=DIRECTION ( 'NONE',  ( 1.000000000000000000, 8.673617379884036705E-17, -0.000000000000000000 ) ) ;
#20131=DIRECTION ( 'NONE',  ( -1.224646799147353207E-16, 1.000000000000000000, 0.000000000000000000 ) ) ;
#20132=CARTESIAN_POINT ( 'NONE',  ( -17.24491960465745777, 0.000000000000000000, 100.0000000000000000 ) ) ;
#20139=ORIENTED_EDGE ( 'NONE', *, *, #26721, .T. ) ;
#20141=ORIENTED_EDGE ( 'NONE', *, *, #21657, .F. ) ;
#20144=CARTESIAN_POINT ( 'NONE',  ( -201.6498696902538939, 93.99348885415903965, -30.47085302539461438 ) ) ;
#20145=ORIENTED_EDGE ( 'NONE', *, *, #7378, .F. ) ;
#20161=CARTESIAN_POINT ( 'NONE',  ( -33.82412182304897641, 129.4067652227780343, -16.89984886922910334 ) ) ;
#20163=DIRECTION ( 'NONE',  ( 0.000000000000000000, 0.000000000000000000, 1.000000000000000000 ) ) ;
#20165=ORIENTED_EDGE ( 'NONE', *, *, #15619, .F. ) ;
#20166=CIRCLE ( 'NONE', #7783, 53.86582179324592090 ) ;
#20169=LINE ( 'NONE', #210, #19206 ) ;
#20170=CARTESIAN_POINT ( 'NONE',  ( -40.40953891503691153, 71.03850157808263077, 99.00000000000000000 ) ) ;
#20171=ORIENTED_EDGE ( 'NONE', *, *, #13712, .F. ) ;
#20172=CARTESIAN_POINT ( 'NONE',  ( -210.0000000000000284, 59.99999999999994316, 17.29233506344265336 ) ) ;
#20175=DIRECTION ( 'NONE',  ( 0.000000000000000000, 0.000000000000000000, 1.000000000000000000 ) ) ;
#20176=DIRECTION ( 'NONE',  ( 1.000000000000000000, 0.000000000000000000, 0.000000000000000000 ) ) ;
#20180=DIRECTION ( 'NONE',  ( -0.5555587585212703461, -0.8314772792026879911, 1.901657040880024000E-15 ) ) ;
#20184=CARTESIAN_POINT ( 'NONE',  ( -227.3172910872899024, 73.27388443547883412, 17.24020071796984155 ) ) ;
#20188=ORIENTED_EDGE ( 'NONE', *, *, #20807, .F. ) ;
#20189=DIRECTION ( 'NONE',  ( 1.000000000000000000, 0.000000000000000000, 0.000000000000000000 ) ) ;
#20191=VECTOR ( 'NONE', #18928, 1000.000000000000000 ) ;
#20194=ORIENTED_EDGE ( 'NONE', *, *, #25406, .F. ) ;
#20195=CARTESIAN_POINT ( 'NONE',  ( 91.45931183162105071, 239.6823639898985050, 17.19464119471847852 ) ) ;
#20200=DIRECTION ( 'NONE',  ( 0.7343588774761952154, -0.6787614006938686995, 0.000000000000000000 ) ) ;
#20203=CARTESIAN_POINT ( 'NONE',  ( 112.4999999999998863, 220.0000000000000284, -105.0000000000000284 ) ) ;
#20206=LINE ( 'NONE', #2673, #16456 ) ;
#20208=EDGE_LOOP ( 'NONE', ( #24203, #8805, #9802, #11472, #20251 ) ) ;
#20213=DIRECTION ( 'NONE',  ( 0.000000000000000000, 0.000000000000000000, 1.000000000000000000 ) ) ;
#20215=AXIS2_PLACEMENT_3D ( 'NONE', #14699, #9299, #27749 ) ;
#20219=VERTEX_POINT ( 'NONE', #3000 ) ;
#20223=CARTESIAN_POINT ( 'NONE',  ( -113.0087222755475267, 134.5426160695832607, 13.86259311301067854 ) ) ;
#20224=DIRECTION ( 'NONE',  ( 0.000000000000000000, 0.000000000000000000, 1.000000000000000000 ) ) ;
#20227=VECTOR ( 'NONE', #23171, 1000.000000000000000 ) ;
#20228=ADVANCED_FACE ( 'NONE', ( #20669 ), #12529, .F. ) ;
#20229=DIRECTION ( 'NONE',  ( -1.000000000000000000, 0.000000000000000000, -0.000000000000000000 ) ) ;
#20231=AXIS2_PLACEMENT_3D ( 'NONE', #11816, #9652, #18548 ) ;
#20232=CARTESIAN_POINT ( 'NONE',  ( -218.1276041038539972, 59.80742093790405534, 25.66002785713338952 ) ) ;
#20235=DIRECTION ( 'NONE',  ( 0.000000000000000000, 0.000000000000000000, -1.000000000000000000 ) ) ;
#20239=CARTESIAN_POINT ( 'NONE',  ( 96.92716526683047107, 115.1868982021512124, 77.49999999971905140 ) ) ;
#20240=EDGE_CURVE ( 'NONE', #28220, #2342, #24453, .T. ) ;
#20241=ADVANCED_FACE ( 'NONE', ( #24414 ), #27269, .F. ) ;
#20242=FACE_OUTER_BOUND ( 'NONE', #20008, .T. ) ;
#20243=DIRECTION ( 'NONE',  ( 1.000000000000000000, 2.602085213965211135E-16, 0.000000000000000000 ) ) ;
#20249=CIRCLE ( 'NONE', #7443, 2.000000000000004885 ) ;
#20251=ORIENTED_EDGE ( 'NONE', *, *, #19271, .F. ) ;
#20253=AXIS2_PLACEMENT_3D ( 'NONE', #7681, #5374, #8099 ) ;
#20254=VERTEX_POINT ( 'NONE', #9766 ) ;
#20257=CARTESIAN_POINT ( 'NONE',  ( -157.8382221595611270, 120.6940372157653485, 22.00304971980720481 ) ) ;
#20258=ORIENTED_EDGE ( 'NONE', *, *, #27218, .T. ) ;
#20273=CARTESIAN_POINT ( 'NONE',  ( -216.4559255058941289, 59.30400871604184232, -28.11406665935971461 ) ) ;
#20275=VERTEX_POINT ( 'NONE', #5438 ) ;
#20277=CARTESIAN_POINT ( 'NONE',  ( -216.4421519707229891, 141.6000904446840707, -15.00000000000000178 ) ) ;
#20279=CARTESIAN_POINT ( 'NONE',  ( -140.1213116003368668, 122.5384136796733827, -13.00000000000000000 ) ) ;
#20282=CARTESIAN_POINT ( 'NONE',  ( -123.8208147886770121, 198.8605305197760913, 12.99999999999999822 ) ) ;
#20284=CARTESIAN_POINT ( 'NONE',  ( -254.3350114625770289, -91.18033988749901653, 16.36034929305424512 ) ) ;
#20289=CARTESIAN_POINT ( 'NONE',  ( 101.7779539749746931, 119.2876405404125393, 82.50000000030260594 ) ) ;
#20291=ORIENTED_EDGE ( 'NONE', *, *, #2082, .T. ) ;
#20292=AXIS2_PLACEMENT_3D ( 'NONE', #2016, #15678, #13522 ) ;
#20294=CARTESIAN_POINT ( 'NONE',  ( -141.6428522700808230, 69.54464929955099706, 83.00000000000001421 ) ) ;
#20295=VECTOR ( 'NONE', #15821, 1000.000000000000000 ) ;
#20297=EDGE_LOOP ( 'NONE', ( #903, #10925 ) ) ;
#20298=CARTESIAN_POINT ( 'NONE',  ( -205.1370039499190625, 144.1304017549904586, 12.99999999999999822 ) ) ;
#20299=ORIENTED_EDGE ( 'NONE', *, *, #600, .T. ) ;
#20302=CARTESIAN_POINT ( 'NONE',  ( -5.209541383816244320, 133.7633409757595757, -15.61671784922240214 ) ) ;
#20303=CARTESIAN_POINT ( 'NONE',  ( -175.0000000000000000, -120.0250000000001904, -69.99999999999998579 ) ) ;
#20307=ORIENTED_EDGE ( 'NONE', *, *, #1286, .T. ) ;
#20308=AXIS2_PLACEMENT_3D ( 'NONE', #21769, #8273, #23779 ) ;
#20310=EDGE_CURVE ( 'NONE', #22340, #25311, #1055, .T. ) ;
#20313=LINE ( 'NONE', #15737, #16688 ) ;
#20314=ORIENTED_EDGE ( 'NONE', *, *, #19066, .T. ) ;
#20317=EDGE_CURVE ( 'NONE', #23684, #7444, #1947, .T. ) ;
#20320=DIRECTION ( 'NONE',  ( 0.000000000000000000, 0.000000000000000000, -1.000000000000000000 ) ) ;
#20321=DIRECTION ( 'NONE',  ( 0.000000000000000000, 0.000000000000000000, 1.000000000000000000 ) ) ;
#20322=DIRECTION ( 'NONE',  ( 0.000000000000000000, -0.000000000000000000, -1.000000000000000000 ) ) ;
#20325=FACE_OUTER_BOUND ( 'NONE', #888, .T. ) ;
#20327=CARTESIAN_POINT ( 'NONE',  ( -97.69448315145120887, 134.5322016254652056, 15.49925189408050841 ) ) ;
#20328=ORIENTED_EDGE ( 'NONE', *, *, #2266, .F. ) ;
#20331=VECTOR ( 'NONE', #28193, 1000.000000000000000 ) ;
#20333=CARTESIAN_POINT ( 'NONE',  ( 134.9999999999998579, 220.0000000000000284, 90.00000000000002842 ) ) ;
#20339=CARTESIAN_POINT ( 'NONE',  ( 99.67744569820828815, 242.4823527582436498, 13.37113024292247054 ) ) ;
#20340=DIRECTION ( 'NONE',  ( -1.000000000000000000, -8.673617379884036705E-17, 0.000000000000000000 ) ) ;
#20342=B_SPLINE_CURVE_WITH_KNOTS ( 'NONE', 3,
 ( #23671, #25256, #7873, #10176, #16643, #8155, #18790, #10314, #6143, #12627, #20945, #27535, #21083, #12763, #27678, #23382, #21366, #16918, #8015, #16782, #12484, #27817, #21225, #23526, #3976, #19353, #5853, #14629, #1549, #27956 ),
 .UNSPECIFIED., .F., .F.,
 ( 4, 2, 2, 2, 2, 2, 2, 2, 2, 2, 2, 2, 2, 2, 4 ),
 ( 0.000000000000000000, 0.002307319121158361939, 0.004614638242316723878, 0.006921957363475085383, 0.009229276484633447755, 0.01384391472695016383, 0.01615123384810852533, 0.01845855296926688857, 0.02307319121158360464, 0.02538051033274192972, 0.02768782945390025133, 0.02999514857505857987, 0.03114880813563770945, 0.03230246769621684250, 0.03691710593853337469 ),
 .UNSPECIFIED. ) ;
#20343=CARTESIAN_POINT ( 'NONE',  ( 98.15430812615089451, 116.0637945823775112, -78.75000000033432457 ) ) ;
#20346=CARTESIAN_POINT ( 'NONE',  ( 79.99999999999994316, -100.0000000000000284, 70.00000000000001421 ) ) ;
#20350=CARTESIAN_POINT ( 'NONE',  ( -24.33210486176665910, 0.000000000000000000, 99.00000000000000000 ) ) ;
#20356=AXIS2_PLACEMENT_3D ( 'NONE', #15851, #4194, #12985 ) ;
#20358=DIRECTION ( 'NONE',  ( -0.5241030343220994814, -0.8516548651973804285, -0.000000000000000000 ) ) ;
#20359=FACE_OUTER_BOUND ( 'NONE', #22940, .T. ) ;
#20364=CARTESIAN_POINT ( 'NONE',  ( 109.9999999999998863, 260.0000000000000000, -45.00000000000000000 ) ) ;
#20365=ORIENTED_EDGE ( 'NONE', *, *, #26185, .T. ) ;
#20366=ORIENTED_EDGE ( 'NONE', *, *, #5684, .F. ) ;
#20373=CARTESIAN_POINT ( 'NONE',  ( 91.50131282131302157, 230.4711573898007373, 17.28742291603535364 ) ) ;
#20374=CARTESIAN_POINT ( 'NONE',  ( -67.45409458357327992, 135.5144413978513001, -13.65941681365853277 ) ) ;
#20377=CARTESIAN_POINT ( 'NONE',  ( -208.5235512171359176, 74.87362916051154116, 38.25286048366049840 ) ) ;
#20380=CARTESIAN_POINT ( 'NONE',  ( 12.13064872364015123, -50.00000000000007105, 98.28427124746193044 ) ) ;
#20382=DIRECTION ( 'NONE',  ( -1.000000000000000000, 0.000000000000000000, 0.000000000000000000 ) ) ;
#20385=CARTESIAN_POINT ( 'NONE',  ( -210.0000000000000284, -40.00000000000005684, 70.00000000000001421 ) ) ;
#20386=CARTESIAN_POINT ( 'NONE',  ( -20.22836655706693776, 129.6440146278404768, 16.81209664567878548 ) ) ;
#20389=CARTESIAN_POINT ( 'NONE',  ( 109.9999999999999574, -120.0000000000000711, -70.00000000000001421 ) ) ;
#20394=CARTESIAN_POINT ( 'NONE',  ( -220.0118810049154661, 86.25235459150694339, -18.72563439332759216 ) ) ;
#20400=CARTESIAN_POINT ( 'NONE',  ( -138.7249983104375133, 128.6417097633065225, 17.20246859800720429 ) ) ;
#20401=VERTEX_POINT ( 'NONE', #10428 ) ;
#20407=CARTESIAN_POINT ( 'NONE',  ( -68.57415822541635464, -23.01420295945612082, 80.00000000000001421 ) ) ;
#20410=EDGE_CURVE ( 'NONE', #1799, #21665, #27928, .T. ) ;
#20413=DIRECTION ( 'NONE',  ( 1.530283246943720875E-16, -1.000000000000000000, 0.000000000000000000 ) ) ;
#20414=CARTESIAN_POINT ( 'NONE',  ( -216.1549772618016334, 59.20708407665082262, -28.62293862808999734 ) ) ;
#20419=ORIENTED_EDGE ( 'NONE', *, *, #12791, .F. ) ;
#20427=AXIS2_PLACEMENT_3D ( 'NONE', #11601, #808, #20340 ) ;
#20429=CIRCLE ( 'NONE', #11252, 80.00000000000000000 ) ;
#20432=DIRECTION ( 'NONE',  ( -1.000000000000000000, 0.000000000000000000, -0.000000000000000000 ) ) ;
#20434=AXIS2_PLACEMENT_3D ( 'NONE', #23999, #19966, #26564 ) ;
#20436=EDGE_CURVE ( 'NONE', #20107, #20401, #18938, .T. ) ;
#20441=DIRECTION ( 'NONE',  ( -1.000000000000000000, 0.000000000000000000, -0.000000000000000000 ) ) ;
#20442=ORIENTED_EDGE ( 'NONE', *, *, #12133, .T. ) ;
#20444=EDGE_CURVE ( 'NONE', #12189, #17779, #28085, .T. ) ;
#20446=CIRCLE ( 'NONE', #13567, 22.49999999999997868 ) ;
#20448=CARTESIAN_POINT ( 'NONE',  ( -160.0000000000000284, 221.6666220619077876, -15.00000000000000000 ) ) ;
#20449=CARTESIAN_POINT ( 'NONE',  ( -1.286094456368339189, 135.5506476309248569, -13.59701399039920844 ) ) ;
#20452=AXIS2_PLACEMENT_3D ( 'NONE', #6928, #22596, #476 ) ;
#20461=ORIENTED_EDGE ( 'NONE', *, *, #16804, .T. ) ;
#20464=CARTESIAN_POINT ( 'NONE',  ( 134.9999999999998579, 220.0000000000000284, -90.00000000000002842 ) ) ;
#20466=FACE_OUTER_BOUND ( 'NONE', #4846, .T. ) ;
#20469=PLANE ( 'NONE',  #26234 ) ;
#20471=DIRECTION ( 'NONE',  ( 1.000000000000000000, 0.000000000000000000, 0.000000000000000000 ) ) ;
#20476=CARTESIAN_POINT ( 'NONE',  ( -17.24491960465745777, -18.01420295945611727, 100.0000000000000000 ) ) ;
#20482=CARTESIAN_POINT ( 'NONE',  ( 109.8651760759796332, 256.6126121035342749, 42.06544492438914773 ) ) ;
#20483=ADVANCED_FACE ( 'NONE', ( #24204 ), #13299, .F. ) ;
#20485=CARTESIAN_POINT ( 'NONE',  ( -228.3260857049913284, 133.0445111367241680, -15.00000000000000355 ) ) ;
#20488=DIRECTION ( 'NONE',  ( -0.8314772792026874360, 0.5555587585212711232, 0.000000000000000000 ) ) ;
#20491=CARTESIAN_POINT ( 'NONE',  ( 113.4999999999998863, 220.0000000000000284, 99.00000000000001421 ) ) ;
#20493=DIRECTION ( 'NONE',  ( 0.000000000000000000, 0.000000000000000000, -1.000000000000000000 ) ) ;
#20501=DIRECTION ( 'NONE',  ( -0.000000000000000000, -0.000000000000000000, 1.000000000000000000 ) ) ;
#20507=VERTEX_POINT ( 'NONE', #4509 ) ;
#20517=CARTESIAN_POINT ( 'NONE',  ( -77.62792406888256380, 134.6615905559135058, -15.47644436303202653 ) ) ;
#20518=CARTESIAN_POINT ( 'NONE',  ( -38.15943738855941803, 129.9964879898109587, 15.32333988264501556 ) ) ;
#20519=CARTESIAN_POINT ( 'NONE',  ( -207.4994891700685002, 75.60264349980251097, 44.78213549412046746 ) ) ;
#20521=CARTESIAN_POINT ( 'NONE',  ( -108.0012317229447376, 135.2240360019066259, -13.71905899893544145 ) ) ;
#20522=CARTESIAN_POINT ( 'NONE',  ( -12.24491960465745599, -23.01420295945612082, 100.0000000000000000 ) ) ;
#20526=CARTESIAN_POINT ( 'NONE',  ( 90.92319367352486381, 112.0484670279021771, 72.65625000014701129 ) ) ;
#20528=CARTESIAN_POINT ( 'NONE',  ( 82.91040908012101340, 80.00000000661717081, -100.0000000000000142 ) ) ;
#20530=ORIENTED_EDGE ( 'NONE', *, *, #14545, .F. ) ;
#20532=VECTOR ( 'NONE', #4990, 1000.000000000000000 ) ;
#20533=CARTESIAN_POINT ( 'NONE',  ( -209.3667759261723234, 88.45076432448455250, -25.75869258754447699 ) ) ;
#20536=EDGE_LOOP ( 'NONE', ( #20442, #536, #14921, #27432 ) ) ;
#20540=CARTESIAN_POINT ( 'NONE',  ( -62.71494712997262155, 133.3675451889207864, 15.73174655005644595 ) ) ;
#20541=ORIENTED_EDGE ( 'NONE', *, *, #14015, .F. ) ;
#20542=EDGE_LOOP ( 'NONE', ( #4240, #1768, #15330, #8372, #10664 ) ) ;
#20543=CARTESIAN_POINT ( 'NONE',  ( -163.8236447719811224, 118.1194741415192482, -24.35161506463292724 ) ) ;
#20545=AXIS2_PLACEMENT_3D ( 'NONE', #19386, #15518, #15379 ) ;
#20548=DIRECTION ( 'NONE',  ( 0.000000000000000000, 0.000000000000000000, 1.000000000000000000 ) ) ;
#20550=CARTESIAN_POINT ( 'NONE',  ( 20.92655468430566756, 155.3461090732848220, -13.00000000000000000 ) ) ;
#20551=DIRECTION ( 'NONE',  ( 1.000000000000000000, 2.602085213965211135E-16, -0.000000000000000000 ) ) ;
#20552=CARTESIAN_POINT ( 'NONE',  ( -208.5306448315634213, 60.03373823553869926, -18.45924612779791474 ) ) ;
#20553=CIRCLE ( 'NONE', #5422, 5.000000000000004441 ) ;
#20554=CARTESIAN_POINT ( 'NONE',  ( 112.4999999999998863, 220.0000000000000284, -84.99999999999997158 ) ) ;
#20561=CARTESIAN_POINT ( 'NONE',  ( -235.8599852676175601, 67.86969485656919687, 15.13802962878585490 ) ) ;
#20566=ORIENTED_EDGE ( 'NONE', *, *, #28115, .T. ) ;
#20568=EDGE_CURVE ( 'NONE', #26119, #24246, #9118, .T. ) ;
#20569=CARTESIAN_POINT ( 'NONE',  ( 109.9999999999999289, 140.0000000000000000, 100.0000000000000142 ) ) ;
#20570=DIRECTION ( 'NONE',  ( 1.000000000000000000, 0.000000000000000000, 0.000000000000000000 ) ) ;
#20575=VECTOR ( 'NONE', #21689, 1000.000000000000000 ) ;
#20577=VERTEX_POINT ( 'NONE', #6535 ) ;
#20578=CARTESIAN_POINT ( 'NONE',  ( 109.9999999999999432, 2.035408878479452500E-14, -90.00000000000004263 ) ) ;
#20580=CARTESIAN_POINT ( 'NONE',  ( -59.48697296830715686, 2.336311854928212824E-15, 99.00000000000000000 ) ) ;
#20583=EDGE_CURVE ( 'NONE', #15830, #26119, #7022, .T. ) ;
#20587=CARTESIAN_POINT ( 'NONE',  ( -33.95367337125702534, 128.1958190094148620, -17.41813228564776139 ) ) ;
#20589=VECTOR ( 'NONE', #19696, 1000.000000000000000 ) ;
#20594=FACE_OUTER_BOUND ( 'NONE', #21616, .T. ) ;
#20598=DIRECTION ( 'NONE',  ( 0.000000000000000000, 0.000000000000000000, -1.000000000000000000 ) ) ;
#20600=EDGE_CURVE ( 'NONE', #17312, #9431, #9797, .T. ) ;
#20603=DIRECTION ( 'NONE',  ( 1.000000000000000000, 0.000000000000000000, 0.000000000000000000 ) ) ;
#20607=LINE ( 'NONE', #9836, #11588 ) ;
#20608=ORIENTED_EDGE ( 'NONE', *, *, #26745, .T. ) ;
#20610=CARTESIAN_POINT ( 'NONE',  ( 134.9999999999998579, 171.5103103742661688, 84.99999999999995737 ) ) ;
#20611=DIRECTION ( 'NONE',  ( 0.000000000000000000, -1.000000000000000000, 0.000000000000000000 ) ) ;
#20614=AXIS2_PLACEMENT_3D ( 'NONE', #19945, #6447, #4565 ) ;
#20621=VECTOR ( 'NONE', #10495, 1000.000000000000000 ) ;
#20625=CARTESIAN_POINT ( 'NONE',  ( -175.0000000000000000, -120.0250000000001762, 64.00000000000001421 ) ) ;
#20634=DIRECTION ( 'NONE',  ( 0.000000000000000000, 0.000000000000000000, -1.000000000000000000 ) ) ;
#20638=CARTESIAN_POINT ( 'NONE',  ( 9.999999999999749534, 90.00000000000001421, 98.28427124746191623 ) ) ;
#20643=TOROIDAL_SURFACE ( 'NONE', #4125, 79.71075545852265520, 9.999999999999996447 ) ;
#20648=VERTEX_POINT ( 'NONE', #5086 ) ;
#20650=VERTEX_POINT ( 'NONE', #13875 ) ;
#20652=CARTESIAN_POINT ( 'NONE',  ( -85.26706196341493182, 136.4560777204422948, 13.48389049418808661 ) ) ;
#20654=DIRECTION ( 'NONE',  ( -1.850371707708594316E-16, 1.000000000000000000, 0.000000000000000000 ) ) ;
#20661=CARTESIAN_POINT ( 'NONE',  ( 79.99999999999992895, 110.0000000000000000, -70.00000000000001421 ) ) ;
#20662=CARTESIAN_POINT ( 'NONE',  ( -229.5850194865393519, 91.64208065330865338, -13.15559042349177687 ) ) ;
#20663=DIRECTION ( 'NONE',  ( -0.000000000000000000, 1.000000000000000000, -0.000000000000000000 ) ) ;
#20666=CARTESIAN_POINT ( 'NONE',  ( 65.00000000000000000, -120.0250000000000625, 70.00000000000001421 ) ) ;
#20667=LINE ( 'NONE', #27401, #14766 ) ;
#20669=FACE_OUTER_BOUND ( 'NONE', #10731, .T. ) ;
#20670=ORIENTED_EDGE ( 'NONE', *, *, #25248, .T. ) ;
#20676=VERTEX_POINT ( 'NONE', #1065 ) ;
#20678=AXIS2_PLACEMENT_3D ( 'NONE', #18016, #13718, #20163 ) ;
#20682=CARTESIAN_POINT ( 'NONE',  ( -528.3536063663644882, -163.3555848104747383, 0.000000000000000000 ) ) ;
#20684=CARTESIAN_POINT ( 'NONE',  ( 9.345921402568901470, 140.0000000000000000, 13.00000000000000000 ) ) ;
#20685=CARTESIAN_POINT ( 'NONE',  ( 100.0424356845176135, 235.0879599625497463, -22.67299618748800327 ) ) ;
#20690=ADVANCED_FACE ( 'NONE', ( #22628 ), #18956, .T. ) ;
#20691=ADVANCED_FACE ( 'NONE', ( #22768 ), #22901, .F. ) ;
#20692=AXIS2_PLACEMENT_3D ( 'NONE', #23383, #3693, #15773 ) ;
#20697=ORIENTED_EDGE ( 'NONE', *, *, #3278, .T. ) ;
#20701=ADVANCED_FACE ( 'NONE', ( #11996 ), #18728, .T. ) ;
#20702=CARTESIAN_POINT ( 'NONE',  ( -232.3551040745953458, 65.57906652092701449, 15.97735746865810214 ) ) ;
#20704=EDGE_LOOP ( 'NONE', ( #17320, #15031, #11482, #10458 ) ) ;
#20707=DIRECTION ( 'NONE',  ( -0.5975062131282562472, 0.8018642810807392607, 0.000000000000000000 ) ) ;
#20709=EDGE_LOOP ( 'NONE', ( #4139, #6865, #2116, #4506 ) ) ;
#20710=ORIENTED_EDGE ( 'NONE', *, *, #9191, .F. ) ;
#20712=CIRCLE ( 'NONE', #28038, 30.00000000000000000 ) ;
#20715=ORIENTED_EDGE ( 'NONE', *, *, #3143, .F. ) ;
#20725=CYLINDRICAL_SURFACE ( 'NONE', #18297, 5.999999999999991118 ) ;
#20727=LINE ( 'NONE', #7667, #21671 ) ;
#20728=EDGE_CURVE ( 'NONE', #7226, #14597, #3493, .T. ) ;
#20736=AXIS2_PLACEMENT_3D ( 'NONE', #3488, #10812, #13122 ) ;
#20737=DIRECTION ( 'NONE',  ( 1.000000000000000000, 0.000000000000000000, 0.000000000000000000 ) ) ;
#20746=EDGE_CURVE ( 'NONE', #19335, #17217, #15299, .T. ) ;
#20748=CARTESIAN_POINT ( 'NONE',  ( 109.5784832860911422, 255.7788523555518054, 37.68001940528806415 ) ) ;
#20749=ORIENTED_EDGE ( 'NONE', *, *, #9503, .F. ) ;
#20752=ORIENTED_EDGE ( 'NONE', *, *, #27368, .F. ) ;
#20753=EDGE_LOOP ( 'NONE', ( #17298, #7006, #5250, #11151 ) ) ;
#20758=CONICAL_SURFACE ( 'NONE', #22132, 6.025000000000002132, 0.7853981633974482790 ) ;
#20760=CARTESIAN_POINT ( 'NONE',  ( -217.6530433929989101, 140.9974892713794645, -15.00000000000000000 ) ) ;
#20764=CARTESIAN_POINT ( 'NONE',  ( 109.5756401952514523, 134.3783162855169451, -89.68749999975639753 ) ) ;
#20766=ADVANCED_FACE ( 'NONE', ( #10116 ), #155, .T. ) ;
#20767=PLANE ( 'NONE',  #19839 ) ;
#20773=CARTESIAN_POINT ( 'NONE',  ( 106.1556986643225002, 248.1950218616640598, -24.28466094498536165 ) ) ;
#20776=DIRECTION ( 'NONE',  ( 0.000000000000000000, 0.000000000000000000, -1.000000000000000000 ) ) ;
#20784=DIRECTION ( 'NONE',  ( -0.7730186417261847298, -0.6343833064826063239, 0.000000000000000000 ) ) ;
#20787=ORIENTED_EDGE ( 'NONE', *, *, #866, .F. ) ;
#20789=EDGE_LOOP ( 'NONE', ( #121, #4728, #9878, #11319, #27714, #8740 ) ) ;
#20792=DIRECTION ( 'NONE',  ( 1.000000000000000000, 0.000000000000000000, 0.000000000000000000 ) ) ;
#20798=DIRECTION ( 'NONE',  ( 0.000000000000000000, 1.000000000000000000, -0.000000000000000000 ) ) ;
#20801=CARTESIAN_POINT ( 'NONE',  ( -196.2821818994568162, 62.43869624199520985, 34.70549414534111321 ) ) ;
#20803=CARTESIAN_POINT ( 'NONE',  ( -77.52393792358382996, 136.3037775726609482, -13.50824672331413723 ) ) ;
#20804=VECTOR ( 'NONE', #2317, 1000.000000000000000 ) ;
#20805=CYLINDRICAL_SURFACE ( 'NONE', #16792, 22.49999999999999289 ) ;
#20807=EDGE_CURVE ( 'NONE', #2640, #22383, #27892, .T. ) ;
#20808=AXIS2_PLACEMENT_3D ( 'NONE', #20170, #7248, #11129 ) ;
#20813=FACE_OUTER_BOUND ( 'NONE', #2528, .T. ) ;
#20814=CARTESIAN_POINT ( 'NONE',  ( 106.3487426207649236, 91.82653269718771583, -100.0000000000000142 ) ) ;
#20818=CARTESIAN_POINT ( 'NONE',  ( 79.99999999999992895, 110.0000000000000000, 45.00000000000000000 ) ) ;
#20820=ORIENTED_EDGE ( 'NONE', *, *, #11348, .T. ) ;
#20822=AXIS2_PLACEMENT_3D ( 'NONE', #21605, #20798, #10554 ) ;
#20823=VERTEX_POINT ( 'NONE', #28032 ) ;
#20830=CARTESIAN_POINT ( 'NONE',  ( 101.0134753670012913, 235.9904216347473778, -23.57078716685460407 ) ) ;
#20831=ADVANCED_FACE ( 'NONE', ( #1895 ), #25474, .F. ) ;
#20833=CARTESIAN_POINT ( 'NONE',  ( -71.37541315349507443, 150.2892445414773590, -15.00000000000000000 ) ) ;
#20834=LINE ( 'NONE', #1153, #7585 ) ;
#20839=DIRECTION ( 'NONE',  ( -1.000000000000000000, 0.000000000000000000, 0.000000000000000000 ) ) ;
#20844=CARTESIAN_POINT ( 'NONE',  ( -230.8916957670046486, 130.8330661503598833, 15.00000000000000000 ) ) ;
#20845=EDGE_CURVE ( 'NONE', #2835, #26591, #2310, .T. ) ;
#20846=DIRECTION ( 'NONE',  ( -0.9611633748070274041, -0.2759800118297804916, 1.182005470438334537E-13 ) ) ;
#20852=EDGE_CURVE ( 'NONE', #22331, #3239, #1523, .T. ) ;
#20862=CARTESIAN_POINT ( 'NONE',  ( -230.9048883912569181, 92.57784203868951067, 15.03157938458457998 ) ) ;
#20863=EDGE_LOOP ( 'NONE', ( #402, #24860, #1408, #15849 ) ) ;
#20867=ADVANCED_FACE ( 'NONE', ( #2179 ), #26316, .F. ) ;
#20873=CARTESIAN_POINT ( 'NONE',  ( -184.0582905406964471, 107.1919238267117720, -32.00588097399845111 ) ) ;
#20877=LINE ( 'NONE', #25598, #13354 ) ;
#20880=ORIENTED_EDGE ( 'NONE', *, *, #9784, .F. ) ;
#20885=CARTESIAN_POINT ( 'NONE',  ( -175.0000000000000000, -120.0000000000001847, -63.97499999999998721 ) ) ;
#20889=AXIS2_PLACEMENT_3D ( 'NONE', #22481, #24783, #218 ) ;
#20903=EDGE_CURVE ( 'NONE', #23690, #4054, #6641, .T. ) ;
#20904=CARTESIAN_POINT ( 'NONE',  ( -180.0000000000000284, -40.00000000000004974, -70.00000000000001421 ) ) ;
#20907=CARTESIAN_POINT ( 'NONE',  ( -112.3221550338875687, 69.54464929955099706, 80.00000000000001421 ) ) ;
#20910=EDGE_CURVE ( 'NONE', #7297, #25488, #15779, .T. ) ;
#20914=CARTESIAN_POINT ( 'NONE',  ( -210.0000000000000000, -120.0000000000001705, 100.0000000000000142 ) ) ;
#20916=CARTESIAN_POINT ( 'NONE',  ( -11.61682370180709079, 131.4608765202114853, 14.74855702008673397 ) ) ;
#20917=CARTESIAN_POINT ( 'NONE',  ( 91.94651231017051884, 240.0740382701074225, -7.116185459647595302 ) ) ;
#20921=DIRECTION ( 'NONE',  ( -1.000000000000000000, -0.000000000000000000, -0.000000000000000000 ) ) ;
#20922=ORIENTED_EDGE ( 'NONE', *, *, #20942, .T. ) ;
#20928=( BOUNDED_SURFACE ( )  B_SPLINE_SURFACE ( 2, 3, ( 
 ( #9945, #25305, #27312, #23157, #27446, #7788, #14403, #12255, #6757, #10796, #8921, #13242, #6477, #21710, #23720, #21560, #28011, #25869, #26007, #1733, #10936, #21418 ),
 ( #12957, #21987, #10508, #8354, #4029, #2295, #17114, #13109, #19555, #15400, #160, #6194, #2021, #6620, #6329, #28295, #15256, #21855, #19266, #15111, #12817, #8639 ),
 ( #3891, #10650, #11077, #17392, #2159, #14970, #1871, #19410, #19834, #26297, #28155, #26153, #8497, #24011, #17252, #24156, #4454, #17678, #4171, #26430, #4318, #19693 ) ),
 .UNSPECIFIED., .F., .F., .T. ) 
 B_SPLINE_SURFACE_WITH_KNOTS ( ( 3, 3 ),
 ( 4, 2, 2, 2, 2, 2, 2, 2, 2, 2, 4 ),
 ( 0.000000000000000000, 1.000000000000000000 ),
 ( 0.000000000000000000, 0.004677071733467426211, 0.009354143466934852422, 0.01403121520040227777, 0.01870828693386970484, 0.02806243040080455553, 0.03741657386773940969, 0.04677071733467426384, 0.05612486080160911106, 0.06547900426854397216, 0.07483314773547881937 ),
 .UNSPECIFIED. ) 
 GEOMETRIC_REPRESENTATION_ITEM ( )  RATIONAL_B_SPLINE_SURFACE ( (
 ( 1.000000000000000000, 1.000000000000000000, 1.000000000000000000, 1.000000000000000000, 1.000000000000000000, 1.000000000000000000, 1.000000000000000000, 1.000000000000000000, 1.000000000000000000, 1.000000000000000000, 1.000000000000000000, 1.000000000000000000, 1.000000000000000000, 1.000000000000000000, 1.000000000000000000, 1.000000000000000000, 1.000000000000000000, 1.000000000000000000, 1.000000000000000000, 1.000000000000000000, 1.000000000000000000, 1.000000000000000000),
 ( 0.7071067811865475727, 0.7071067811865475727, 0.7071067811865476838, 0.7071067811865476838, 0.7071067811865473507, 0.7071067811865473507, 0.7071067811865473507, 0.7071067811865473507, 0.7071067811865474617, 0.7071067811865474617, 0.7071067811865476838, 0.7071067811865476838, 0.7071067811865477948, 0.7071067811865477948, 0.7071067811865473507, 0.7071067811865473507, 0.7071067811865475727, 0.7071067811865475727, 0.7071067811865475727, 0.7071067811865475727, 0.7071067811865484609, 0.7071067811865484609),
 ( 1.000000000000000000, 1.000000000000000000, 1.000000000000000000, 1.000000000000000000, 1.000000000000000000, 1.000000000000000000, 1.000000000000000000, 1.000000000000000000, 1.000000000000000000, 1.000000000000000000, 1.000000000000000000, 1.000000000000000000, 1.000000000000000000, 1.000000000000000000, 1.000000000000000000, 1.000000000000000000, 1.000000000000000000, 1.000000000000000000, 1.000000000000000000, 1.000000000000000000, 1.000000000000000000, 1.000000000000000000) ) ) 
 REPRESENTATION_ITEM ( '' )  SURFACE ( )  );
#20931=EDGE_CURVE ( 'NONE', #11179, #18978, #19424, .T. ) ;
#20935=CYLINDRICAL_SURFACE ( 'NONE', #2639, 5.000000000000004441 ) ;
#20937=CARTESIAN_POINT ( 'NONE',  ( -157.8317677482887973, 120.6968079807819407, -22.00051853850753147 ) ) ;
#20941=CARTESIAN_POINT ( 'NONE',  ( -156.3854698478411649, 122.2179277774955466, -19.69657316895759536 ) ) ;
#20942=EDGE_CURVE ( 'NONE', #9382, #7691, #10818, .T. ) ;
#20945=CARTESIAN_POINT ( 'NONE',  ( -212.2904188450821152, 87.25517758443818650, 23.57528053420220360 ) ) ;
#20946=AXIS2_PLACEMENT_3D ( 'NONE', #16607, #12447, #7980 ) ;
#20951=CARTESIAN_POINT ( 'NONE',  ( -38.27121137906592452, -18.98690351477092619, 99.90775530369607793 ) ) ;
#20952=CARTESIAN_POINT ( 'NONE',  ( 100.8904249506145874, 86.57652225509636423, -100.0000000000000142 ) ) ;
#20962=ORIENTED_EDGE ( 'NONE', *, *, #25091, .F. ) ;
#20966=VERTEX_POINT ( 'NONE', #13547 ) ;
#20967=FACE_OUTER_BOUND ( 'NONE', #27977, .T. ) ;
#20970=CARTESIAN_POINT ( 'NONE',  ( 1.554977376564339764, 135.1207837442669870, -15.37741204235645931 ) ) ;
#20971=DIRECTION ( 'NONE',  ( 1.850371707708594316E-16, -1.000000000000000000, -0.000000000000000000 ) ) ;
#20973=CARTESIAN_POINT ( 'NONE',  ( -194.2306746384193730, 63.21821459927384979, -44.70951427402087575 ) ) ;
#20974=VECTOR ( 'NONE', #698, 1000.000000000000000 ) ;
#20979=ORIENTED_EDGE ( 'NONE', *, *, #708, .T. ) ;
#20980=DIRECTION ( 'NONE',  ( 0.5241030343220994814, 0.8516548651973804285, -0.000000000000000000 ) ) ;
#20981=LINE ( 'NONE', #25023, #23190 ) ;
#20982=ORIENTED_EDGE ( 'NONE', *, *, #2120, .F. ) ;
#20988=CARTESIAN_POINT ( 'NONE',  ( 93.07270601806959576, 112.9533406969986231, 99.99999999997838529 ) ) ;
#20993=CARTESIAN_POINT ( 'NONE',  ( 109.9999999999999432, 259.1952685963541967, 44.30308214094263519 ) ) ;
#21010=CARTESIAN_POINT ( 'NONE',  ( -180.0000000000000284, -40.00000000000004974, 100.0000000000000142 ) ) ;
#21013=ORIENTED_EDGE ( 'NONE', *, *, #4124, .T. ) ;
#21016=CARTESIAN_POINT ( 'NONE',  ( -189.7025054116240881, 103.6028096261271259, 32.02907974114463485 ) ) ;
#21017=FACE_OUTER_BOUND ( 'NONE', #9463, .T. ) ;
#21021=DIRECTION ( 'NONE',  ( 0.000000000000000000, 0.000000000000000000, -1.000000000000000000 ) ) ;
#21024=EDGE_CURVE ( 'NONE', #1063, #7087, #22592, .T. ) ;
#21025=EDGE_CURVE ( 'NONE', #22340, #1342, #26894, .T. ) ;
#21027=ADVANCED_FACE ( 'NONE', ( #616 ), #9380, .F. ) ;
#21033=CIRCLE ( 'NONE', #1304, 2.000000000000000000 ) ;
#21037=ORIENTED_EDGE ( 'NONE', *, *, #25248, .F. ) ;
#21038=CARTESIAN_POINT ( 'NONE',  ( 109.9999999999459703, 259.2933449746407746, 44.14322629295149625 ) ) ;
#21042=DIRECTION ( 'NONE',  ( 1.000000000000000000, 0.000000000000000000, 0.000000000000000000 ) ) ;
#21044=VECTOR ( 'NONE', #20128, 1000.000000000000000 ) ;
#21045=DIRECTION ( 'NONE',  ( 0.000000000000000000, 0.000000000000000000, -1.000000000000000000 ) ) ;
#21056=CARTESIAN_POINT ( 'NONE',  ( 106.4996638054810489, 248.6817669671922317, -25.16380096945068345 ) ) ;
#21058=DIRECTION ( 'NONE',  ( -1.000000000000000000, 0.000000000000000000, 0.000000000000000000 ) ) ;
#21063=ORIENTED_EDGE ( 'NONE', *, *, #12775, .F. ) ;
#21064=ADVANCED_FACE ( 'NONE', ( #9660 ), #10107, .T. ) ;
#21066=ORIENTED_EDGE ( 'NONE', *, *, #4448, .T. ) ;
#21068=CARTESIAN_POINT ( 'NONE',  ( -82.72863776448107842, 136.4212039060443828, 15.16706508184716462 ) ) ;
#21070=CIRCLE ( 'NONE', #28391, 41.00000000000000711 ) ;
#21072=ORIENTED_EDGE ( 'NONE', *, *, #3680, .T. ) ;
#21075=CARTESIAN_POINT ( 'NONE',  ( -273.6211430000234373, -91.18033988749901653, -14.64217782292691261 ) ) ;
#21076=CIRCLE ( 'NONE', #8694, 19.07743405327024888 ) ;
#21081=CARTESIAN_POINT ( 'NONE',  ( -124.9781469243919076, 222.2250949724356985, -5.000000000000004441 ) ) ;
#21083=CARTESIAN_POINT ( 'NONE',  ( -214.7594651349411379, 86.63962098186175353, 21.86053752875909240 ) ) ;
#21090=DIRECTION ( 'NONE',  ( -0.000000000000000000, -0.000000000000000000, 1.000000000000000000 ) ) ;
#21094=CIRCLE ( 'NONE', #3183, 30.00000000000000000 ) ;
#21100=EDGE_CURVE ( 'NONE', #15024, #15785, #10721, .T. ) ;
#21104=DIRECTION ( 'NONE',  ( 0.000000000000000000, 0.000000000000000000, 1.000000000000000000 ) ) ;
#21105=VECTOR ( 'NONE', #6096, 1000.000000000000000 ) ;
#21110=CARTESIAN_POINT ( 'NONE',  ( -24.83510602130289513, 128.0375039002065023, -17.48817921712931067 ) ) ;
#21113=PLANE ( 'NONE',  #22435 ) ;
#21114=LINE ( 'NONE', #7904, #1950 ) ;
#21118=PLANE ( 'NONE',  #4225 ) ;
#21121=AXIS2_PLACEMENT_3D ( 'NONE', #12444, #18749, #1777 ) ;
#21131=DIRECTION ( 'NONE',  ( 0.000000000000000000, 0.000000000000000000, -1.000000000000000000 ) ) ;
#21132=ORIENTED_EDGE ( 'NONE', *, *, #16504, .F. ) ;
#21138=CARTESIAN_POINT ( 'NONE',  ( 119.9999999999999147, 140.0000000000000000, 100.0000000000000142 ) ) ;
#21140=CARTESIAN_POINT ( 'NONE',  ( -71.37541315349507443, 229.9999999999999716, 5.000000000000002665 ) ) ;
#21141=EDGE_CURVE ( 'NONE', #28035, #16979, #4482, .T. ) ;
#21143=DIRECTION ( 'NONE',  ( 0.000000000000000000, 0.000000000000000000, 1.000000000000000000 ) ) ;
#21146=DIRECTION ( 'NONE',  ( 0.000000000000000000, 0.000000000000000000, 1.000000000000000000 ) ) ;
#21151=ORIENTED_EDGE ( 'NONE', *, *, #7748, .T. ) ;
#21159=ORIENTED_EDGE ( 'NONE', *, *, #8054, .F. ) ;
#21160=CARTESIAN_POINT ( 'NONE',  ( -186.1065741236299402, 106.0956363990103029, 31.60904046745896423 ) ) ;
#21161=DIRECTION ( 'NONE',  ( 0.000000000000000000, 0.7071067811865476838, 0.7071067811865474617 ) ) ;
#21175=CIRCLE ( 'NONE', #27143, 6.000000000000005329 ) ;
#21179=DIRECTION ( 'NONE',  ( 0.000000000000000000, 0.000000000000000000, -1.000000000000000000 ) ) ;
#21180=EDGE_CURVE ( 'NONE', #11217, #10760, #15717, .T. ) ;
#21181=DIRECTION ( 'NONE',  ( 1.000000000000000000, 0.000000000000000000, 0.000000000000000000 ) ) ;
#21185=CARTESIAN_POINT ( 'NONE',  ( -222.4720504096164291, 61.14635810691093099, -21.27434031931761993 ) ) ;
#21187=ADVANCED_FACE ( 'NONE', ( #480 ), #21749, .F. ) ;
#21193=ORIENTED_EDGE ( 'NONE', *, *, #16901, .T. ) ;
#21194=DIRECTION ( 'NONE',  ( 1.000000000000000000, 0.000000000000000000, 0.000000000000000000 ) ) ;
#21196=DIRECTION ( 'NONE',  ( -0.000000000000000000, -0.000000000000000000, 1.000000000000000000 ) ) ;
#21198=CARTESIAN_POINT ( 'NONE',  ( -219.2467648448761395, 139.5102435001769265, -15.00000000000000000 ) ) ;
#21205=VECTOR ( 'NONE', #27029, 1000.000000000000227 ) ;
#21207=CARTESIAN_POINT ( 'NONE',  ( -47.90498801636491066, 130.8804178995914071, 16.39302846298827276 ) ) ;
#21208=CIRCLE ( 'NONE', #12044, 1.000000000000000888 ) ;
#21213=CARTESIAN_POINT ( 'NONE',  ( 112.5876798426282619, 222.0498046809461812, 96.71269508460407849 ) ) ;
#21217=CARTESIAN_POINT ( 'NONE',  ( -144.7212326927123627, 126.7045300270324759, -16.81628189632150239 ) ) ;
#21220=DIRECTION ( 'NONE',  ( 0.000000000000000000, 0.000000000000000000, -1.000000000000000000 ) ) ;
#21221=CARTESIAN_POINT ( 'NONE',  ( 21.29940527161770092, -47.79570116690157988, 98.97008483812450663 ) ) ;
#21222=CARTESIAN_POINT ( 'NONE',  ( -230.9605477664340185, 90.10120975743322447, -15.13325285068605730 ) ) ;
#21223=ADVANCED_FACE ( 'NONE', ( #6512 ), #13895, .T. ) ;
#21225=CARTESIAN_POINT ( 'NONE',  ( -226.9685481008362160, 87.85634458782620015, 15.93431596749161905 ) ) ;
#21235=EDGE_LOOP ( 'NONE', ( #23335, #24643 ) ) ;
#21238=CARTESIAN_POINT ( 'NONE',  ( 102.0697454929915295, 243.6045995028978837, -24.40655498894130915 ) ) ;
#21246=LINE ( 'NONE', #3572, #27385 ) ;
#21247=EDGE_CURVE ( 'NONE', #6227, #17385, #15293, .T. ) ;
#21248=AXIS2_PLACEMENT_3D ( 'NONE', #14429, #5370, #3210 ) ;
#21250=TOROIDAL_SURFACE ( 'NONE', #12557, 60.59270260175150469, 2.000000000000000000 ) ;
#21251=FACE_OUTER_BOUND ( 'NONE', #18807, .T. ) ;
#21254=CARTESIAN_POINT ( 'NONE',  ( 109.9999999999999432, -100.0000000000000142, 25.00000000000000711 ) ) ;
#21256=CARTESIAN_POINT ( 'NONE',  ( -214.5110300873075460, 71.95898175746583547, -27.23319810813256581 ) ) ;
#21259=FACE_OUTER_BOUND ( 'NONE', #2730, .T. ) ;
#21261=DIRECTION ( 'NONE',  ( 1.000000000000000000, 0.000000000000000000, 0.000000000000000000 ) ) ;
#21262=ORIENTED_EDGE ( 'NONE', *, *, #27825, .T. ) ;
#21264=CARTESIAN_POINT ( 'NONE',  ( -191.5097490750847555, 102.3060819963840231, 32.04619225362230139 ) ) ;
#21267=ORIENTED_EDGE ( 'NONE', *, *, #7378, .T. ) ;
#21273=CARTESIAN_POINT ( 'NONE',  ( 87.74278500254594348, 111.0010834410967959, 100.0000000000108429 ) ) ;
#21280=CARTESIAN_POINT ( 'NONE',  ( -185.5167513424577237, 106.4752583619456914, -31.41993102962858231 ) ) ;
#21281=ORIENTED_EDGE ( 'NONE', *, *, #24, .F. ) ;
#21282=CARTESIAN_POINT ( 'NONE',  ( -231.9378824387731299, 93.53122965655670384, 13.00000000000000000 ) ) ;
#21285=DIRECTION ( 'NONE',  ( -1.000000000000000000, 0.000000000000000000, 0.000000000000000000 ) ) ;
#21290=CARTESIAN_POINT ( 'NONE',  ( -229.2498027451138967, 132.0565166830976978, -13.00000000000000000 ) ) ;
#21292=ORIENTED_EDGE ( 'NONE', *, *, #22126, .F. ) ;
#21296=DIRECTION ( 'NONE',  ( 1.000000000000000000, 0.000000000000000000, 0.000000000000000000 ) ) ;
#21310=DIRECTION ( 'NONE',  ( 0.000000000000000000, 1.000000000000000000, 0.000000000000000000 ) ) ;
#21313=VECTOR ( 'NONE', #10891, 1000.000000000000000 ) ;
#21317=ORIENTED_EDGE ( 'NONE', *, *, #26745, .F. ) ;
#21320=ORIENTED_EDGE ( 'NONE', *, *, #8426, .F. ) ;
#21327=FACE_BOUND ( 'NONE', #20297, .T. ) ;
#21328=CARTESIAN_POINT ( 'NONE',  ( -243.4193540313403901, 74.61988491600907025, -4.999999999761307379 ) ) ;
#21333=DIRECTION ( 'NONE',  ( 0.000000000000000000, 0.000000000000000000, 1.000000000000000000 ) ) ;
#21335=ORIENTED_EDGE ( 'NONE', *, *, #5735, .T. ) ;
#21336=DIRECTION ( 'NONE',  ( 0.000000000000000000, 0.000000000000000000, -1.000000000000000000 ) ) ;
#21337=CARTESIAN_POINT ( 'NONE',  ( 98.49253114489452798, 241.8754259314115416, -12.06625762472412333 ) ) ;
#21338=CARTESIAN_POINT ( 'NONE',  ( -68.57415822541635464, 80.97823757117562593, 100.0000000000000000 ) ) ;
#21347=EDGE_CURVE ( 'NONE', #8966, #16772, #16247, .T. ) ;
#21349=VECTOR ( 'NONE', #12203, 1000.000000000000000 ) ;
#21356=CARTESIAN_POINT ( 'NONE',  ( 112.4997598733875606, 220.5042645990800168, 96.61410599988441561 ) ) ;
#21357=CARTESIAN_POINT ( 'NONE',  ( -148.6329411077882980, 124.2076589707419316, -19.48823061374897847 ) ) ;
#21359=CARTESIAN_POINT ( 'NONE',  ( -155.6066793474805934, 121.6020800752544773, -21.27933238366888347 ) ) ;
#21362=CARTESIAN_POINT ( 'NONE',  ( -76.25760768171835480, 221.6666220619076739, -15.00000000000000000 ) ) ;
#21363=CARTESIAN_POINT ( 'NONE',  ( -230.3334077407527900, 89.66896290591726881, -15.21539592855700107 ) ) ;
#21366=CARTESIAN_POINT ( 'NONE',  ( -220.0112564482956827, 86.21625987271094971, 18.70212642463580011 ) ) ;
#21373=ADVANCED_FACE ( 'NONE', ( #5061 ), #19896, .T. ) ;
#21375=DIRECTION ( 'NONE',  ( 1.000000000000000000, 0.000000000000000000, -0.000000000000000000 ) ) ;
#21377=AXIS2_PLACEMENT_3D ( 'NONE', #26408, #23986, #20235 ) ;
#21380=CARTESIAN_POINT ( 'NONE',  ( 95.55652878160884711, 240.7834791927022593, -9.443977278911061646 ) ) ;
#21384=EDGE_LOOP ( 'NONE', ( #27613, #23792, #4418, #4792 ) ) ;
#21388=EDGE_LOOP ( 'NONE', ( #6966, #11011, #8391, #6034 ) ) ;
#21393=CARTESIAN_POINT ( 'NONE',  ( -270.1025481742786951, -91.18033988749901653, -14.95564396479129243 ) ) ;
#21396=DIRECTION ( 'NONE',  ( 1.541976423090495387E-16, -1.000000000000000000, 0.000000000000000000 ) ) ;
#21398=DIRECTION ( 'NONE',  ( 0.000000000000000000, 0.000000000000000000, -1.000000000000000000 ) ) ;
#21399=DIRECTION ( 'NONE',  ( 1.000000000000000000, 0.000000000000000000, 0.000000000000000000 ) ) ;
#21400=CARTESIAN_POINT ( 'NONE',  ( -180.0000000000000284, -40.00000000000004974, 80.00000000000001421 ) ) ;
#21402=DIRECTION ( 'NONE',  ( 0.000000000000000000, 0.000000000000000000, -1.000000000000000000 ) ) ;
#21405=AXIS2_PLACEMENT_3D ( 'NONE', #8534, #28189, #15433 ) ;
#21406=CARTESIAN_POINT ( 'NONE',  ( -201.7499912683865091, 94.28702343169450728, 30.02677094166775973 ) ) ;
#21407=ADVANCED_FACE ( 'NONE', ( #9670 ), #25036, .F. ) ;
#21413=CARTESIAN_POINT ( 'NONE',  ( 91.70829090827390928, 81.72138244997330503, 100.0000000000000142 ) ) ;
#21416=VERTEX_POINT ( 'NONE', #14682 ) ;
#21417=ORIENTED_EDGE ( 'NONE', *, *, #17656, .T. ) ;
#21418=CARTESIAN_POINT ( 'NONE',  ( 109.9999999999999147, 140.0000000000000000, -90.00000000000004263 ) ) ;
#21420=FACE_OUTER_BOUND ( 'NONE', #14371, .T. ) ;
#21421=CARTESIAN_POINT ( 'NONE',  ( -194.9019931824072671, 99.79035201896546425, -31.71427557561374400 ) ) ;
#21423=FACE_OUTER_BOUND ( 'NONE', #20863, .T. ) ;
#21429=DIRECTION ( 'NONE',  ( 0.000000000000000000, -0.000000000000000000, -1.000000000000000000 ) ) ;
#21442=CARTESIAN_POINT ( 'NONE',  ( -215.3193997209569091, 87.88581180658771075, 19.30547682902748718 ) ) ;
#21444=DIRECTION ( 'NONE',  ( 2.602085213965211135E-16, -1.000000000000000000, 0.000000000000000000 ) ) ;
#21446=AXIS2_PLACEMENT_3D ( 'NONE', #8606, #21529, #8467 ) ;
#21448=CARTESIAN_POINT ( 'NONE',  ( -194.9552809774316984, 99.75015356803743316, -32.14979201052287294 ) ) ;
#21449=VERTEX_POINT ( 'NONE', #19124 ) ;
#21450=EDGE_LOOP ( 'NONE', ( #23681, #17445, #3179 ) ) ;
#21453=EDGE_CURVE ( 'NONE', #23180, #18280, #3893, .T. ) ;
#21456=EDGE_LOOP ( 'NONE', ( #4732, #17919, #22974, #9907, #1450 ) ) ;
#21458=CIRCLE ( 'NONE', #25135, 30.00000000000000000 ) ;
#21462=DIRECTION ( 'NONE',  ( -0.000000000000000000, -0.000000000000000000, 1.000000000000000000 ) ) ;
#21463=ADVANCED_FACE ( 'NONE', ( #21420 ), #8209, .F. ) ;
#21465=CARTESIAN_POINT ( 'NONE',  ( 119.9999999999999432, 2.220446049250311819E-14, -90.00000000000004263 ) ) ;
#21466=CARTESIAN_POINT ( 'NONE',  ( -240.4233474261315564, 71.57180907112889656, -14.67903078147014462 ) ) ;
#21467=ORIENTED_EDGE ( 'NONE', *, *, #17656, .F. ) ;
#21468=EDGE_CURVE ( 'NONE', #5857, #11653, #2260, .T. ) ;
#21471=DIRECTION ( 'NONE',  ( 1.000000000000000000, 2.602085213965211135E-16, -0.000000000000000000 ) ) ;
#21477=LINE ( 'NONE', #8696, #6863 ) ;
#21487=ORIENTED_EDGE ( 'NONE', *, *, #4797, .F. ) ;
#21490=EDGE_CURVE ( 'NONE', #17312, #23965, #26975, .T. ) ;
#21493=PLANE ( 'NONE',  #10427 ) ;
#21494=CARTESIAN_POINT ( 'NONE',  ( -100.1083977795999687, 134.3105318853753829, -15.54432045859607214 ) ) ;
#21497=CARTESIAN_POINT ( 'NONE',  ( -136.9828056817498805, 127.8991175801959486, -17.53799436710524873 ) ) ;
#21501=CARTESIAN_POINT ( 'NONE',  ( -223.1974999251100940, 88.61692301512375991, -14.90038877616663093 ) ) ;
#21509=ORIENTED_EDGE ( 'NONE', *, *, #24362, .T. ) ;
#21512=CIRCLE ( 'NONE', #6829, 24.07986109634097005 ) ;
#21513=CARTESIAN_POINT ( 'NONE',  ( -2.862293735361731706E-14, 109.9999999999999858, 45.00000000000000000 ) ) ;
#21514=DIRECTION ( 'NONE',  ( -1.000000000000000000, 6.752478448789676648E-18, 0.000000000000000000 ) ) ;
#21515=EDGE_CURVE ( 'NONE', #13234, #1913, #11338, .T. ) ;
#21516=CARTESIAN_POINT ( 'NONE',  ( -180.0000000000000284, -70.00000000000004263, 100.0000000000000142 ) ) ;
#21517=ORIENTED_EDGE ( 'NONE', *, *, #11410, .T. ) ;
#21520=CARTESIAN_POINT ( 'NONE',  ( 96.65725945967911059, 241.1367295422510040, -10.34535073431741026 ) ) ;
#21527=EDGE_LOOP ( 'NONE', ( #17126, #6854, #7365, #6192 ) ) ;
#21529=DIRECTION ( 'NONE',  ( -0.000000000000000000, 1.000000000000000000, -0.000000000000000000 ) ) ;
#21530=AXIS2_PLACEMENT_3D ( 'NONE', #1572, #6166, #6021 ) ;
#21531=DIRECTION ( 'NONE',  ( 0.8018642810807399268, 0.5975062131282553590, -0.000000000000000000 ) ) ;
#21532=CARTESIAN_POINT ( 'NONE',  ( 105.9597133717324482, 242.8246303622935613, -29.94432334375205684 ) ) ;
#21539=CARTESIAN_POINT ( 'NONE',  ( -226.4322288603291611, 72.85292568147782788, -17.64883888685613655 ) ) ;
#21548=CARTESIAN_POINT ( 'NONE',  ( -177.6132461524688324, 111.0955659291485205, 29.96501893502363956 ) ) ;
#21555=CARTESIAN_POINT ( 'NONE',  ( 82.68942924491597068, 110.0997128792283917, 100.0000000000000142 ) ) ;
#21560=CARTESIAN_POINT ( 'NONE',  ( 104.1118574119011555, 122.0584436052145918, -84.84374999967577935 ) ) ;
#21561=VECTOR ( 'NONE', #27560, 1000.000000000000000 ) ;
#21565=CARTESIAN_POINT ( 'NONE',  ( -220.2843281297837734, 86.23357641588329159, 18.56285956431874595 ) ) ;
#21567=DIRECTION ( 'NONE',  ( 0.000000000000000000, 0.000000000000000000, -1.000000000000000000 ) ) ;
#21576=CARTESIAN_POINT ( 'NONE',  ( -37.82257053376181233, 36.92584315232891612, 100.0000000000000000 ) ) ;
#21583=AXIS2_PLACEMENT_3D ( 'NONE', #16714, #12414, #12273 ) ;
#21589=DIRECTION ( 'NONE',  ( -0.000000000000000000, -0.000000000000000000, 1.000000000000000000 ) ) ;
#21590=EDGE_LOOP ( 'NONE', ( #26074, #3676, #11288, #20109 ) ) ;
#21591=CARTESIAN_POINT ( 'NONE',  ( -144.0897808543928704, 125.7560339784919705, 18.58146195516149390 ) ) ;
#21592=CARTESIAN_POINT ( 'NONE',  ( -169.2805883261569306, 115.5450669606412220, -26.60823203878023691 ) ) ;
#21593=ORIENTED_EDGE ( 'NONE', *, *, #19238, .F. ) ;
#21595=DIRECTION ( 'NONE',  ( -0.8142945039115421224, -0.5804519453834706688, 0.000000000000000000 ) ) ;
#21601=CARTESIAN_POINT ( 'NONE',  ( 7.470826767499499255, 138.6324086774095576, 14.99999999999999822 ) ) ;
#21605=CARTESIAN_POINT ( 'NONE',  ( -180.0000000000000284, -40.00000000000004974, -70.00000000000001421 ) ) ;
#21609=CARTESIAN_POINT ( 'NONE',  ( -235.5733620266657340, 80.43390826602529842, -15.03591609561508946 ) ) ;
#21611=DIRECTION ( 'NONE',  ( 2.602085213965211135E-16, -1.000000000000000000, 0.000000000000000000 ) ) ;
#21614=CARTESIAN_POINT ( 'NONE',  ( 123.9999999999998579, 220.0000000000000284, -99.00000000000001421 ) ) ;
#21616=EDGE_LOOP ( 'NONE', ( #22048, #453, #10953, #27630 ) ) ;
#21629=ORIENTED_EDGE ( 'NONE', *, *, #14537, .T. ) ;
#21631=VERTEX_POINT ( 'NONE', #15938 ) ;
#21633=ORIENTED_EDGE ( 'NONE', *, *, #1695, .F. ) ;
#21635=B_SPLINE_CURVE_WITH_KNOTS ( 'NONE', 3,
 ( #26974, #11770, #24829, #835, #27250, #25103, #7591, #5138, #1113, #13928, #22531, #3113, #16358, #20223, #9604, #18365, #555, #2695, #20652, #27384, #971, #24967, #5284, #14066, #24684, #18506, #15795, #5417 ),
 .UNSPECIFIED., .F., .F.,
 ( 4, 2, 2, 2, 2, 2, 2, 2, 2, 2, 2, 2, 2, 4 ),
 ( 3.469446951953614189E-18, 0.007613765012984346874, 0.01522753002596869028, 0.02284129503895303281, 0.02664817754544523271, 0.03045506005193743260, 0.04568259007790598236, 0.06091012010387453213, 0.07613765012984308189, 0.07994453263633524709, 0.08375141514282739841, 0.09136518015581171492, 0.1065927101817803480, 0.1218202402077489810 ),
 .UNSPECIFIED. ) ;
#21643=CARTESIAN_POINT ( 'NONE',  ( 134.9999999999998579, 220.0000000000000284, -99.00000000000001421 ) ) ;
#21649=CARTESIAN_POINT ( 'NONE',  ( -229.6379567168639539, 91.66739380564841611, -13.14213637420301062 ) ) ;
#21655=EDGE_LOOP ( 'NONE', ( #8105, #1272 ) ) ;
#21656=ADVANCED_FACE ( 'NONE', ( #7450 ), #27253, .F. ) ;
#21657=EDGE_CURVE ( 'NONE', #15640, #1333, #22955, .T. ) ;
#21658=DIRECTION ( 'NONE',  ( -0.000000000000000000, 1.000000000000000000, -1.387778780781445429E-16 ) ) ;
#21663=CARTESIAN_POINT ( 'NONE',  ( 107.1040180392036518, 249.6169203092518103, -26.84244457534687101 ) ) ;
#21664=ORIENTED_EDGE ( 'NONE', *, *, #1773, .F. ) ;
#21665=VERTEX_POINT ( 'NONE', #5710 ) ;
#21667=ADVANCED_FACE ( 'NONE', ( #8009 ), #16775, .F. ) ;
#21671=VECTOR ( 'NONE', #18580, 1000.000000000000000 ) ;
#21672=EDGE_LOOP ( 'NONE', ( #12078, #17179, #13519, #12981 ) ) ;
#21678=EDGE_CURVE ( 'NONE', #23617, #11481, #1116, .T. ) ;
#21679=CARTESIAN_POINT ( 'NONE',  ( -248.1546605714623013, -91.18033988749901653, 0.000000000000000000 ) ) ;
#21682=DIRECTION ( 'NONE',  ( 1.000000000000000000, 0.000000000000000000, 0.000000000000000000 ) ) ;
#21685=CIRCLE ( 'NONE', #9312, 43.76444293738737912 ) ;
#21688=VECTOR ( 'NONE', #6683, 1000.000000000000000 ) ;
#21689=DIRECTION ( 'NONE',  ( 1.000000000000000000, -0.000000000000000000, -0.000000000000000000 ) ) ;
#21694=ORIENTED_EDGE ( 'NONE', *, *, #1662, .F. ) ;
#21696=CARTESIAN_POINT ( 'NONE',  ( -181.2851160895673104, 108.9255553334400588, 31.23174333049976426 ) ) ;
#21700=ORIENTED_EDGE ( 'NONE', *, *, #22342, .T. ) ;
#21702=ORIENTED_EDGE ( 'NONE', *, *, #28314, .F. ) ;
#21707=AXIS2_PLACEMENT_3D ( 'NONE', #17203, #3979, #1966 ) ;
#21710=CARTESIAN_POINT ( 'NONE',  ( 100.5794065449870942, 118.1137289701970872, -81.24999999966573228 ) ) ;
#21712=CARTESIAN_POINT ( 'NONE',  ( 88.54392178150615678, 230.0000000000000284, 16.22216434841215360 ) ) ;
#21713=CARTESIAN_POINT ( 'NONE',  ( -168.1663021066853787, 116.6858039761555119, -24.56336007714330449 ) ) ;
#21715=CARTESIAN_POINT ( 'NONE',  ( -227.1642097121179233, 90.19069637679466211, 13.60986389833546717 ) ) ;
#21716=ORIENTED_EDGE ( 'NONE', *, *, #13897, .F. ) ;
#21721=PLANE ( 'NONE',  #47 ) ;
#21724=CARTESIAN_POINT ( 'NONE',  ( 134.9999999999998579, 220.0000000000000284, -105.0000000000000284 ) ) ;
#21726=CARTESIAN_POINT ( 'NONE',  ( -42.99650729631200363, 71.03850157808263077, 100.0000000000000000 ) ) ;
#21732=ADVANCED_FACE ( 'NONE', ( #24970 ), #14342, .F. ) ;
#21733=DIRECTION ( 'NONE',  ( -2.312964634635742464E-16, 1.000000000000000000, 0.000000000000000000 ) ) ;
#21734=CARTESIAN_POINT ( 'NONE',  ( -17.24491960465746132, 75.97823757117562593, 80.00000000000001421 ) ) ;
#21739=LINE ( 'NONE', #28320, #27593 ) ;
#21740=CARTESIAN_POINT ( 'NONE',  ( -160.8326600028555617, 120.2355194873574789, -21.37420696376538842 ) ) ;
#21741=ORIENTED_EDGE ( 'NONE', *, *, #10039, .T. ) ;
#21744=VERTEX_POINT ( 'NONE', #18508 ) ;
#21749=PLANE ( 'NONE',  #7045 ) ;
#21753=AXIS2_PLACEMENT_3D ( 'NONE', #14779, #24876, #18411 ) ;
#21756=CARTESIAN_POINT ( 'NONE',  ( 134.9999999999998579, 220.0000000000000284, -100.0000000000000142 ) ) ;
#21758=CARTESIAN_POINT ( 'NONE',  ( -63.57415822541634043, 75.97823757117562593, 95.00000000000000000 ) ) ;
#21760=CARTESIAN_POINT ( 'NONE',  ( -239.3181950532627980, 70.57797675263729786, -14.71337737011382352 ) ) ;
#21764=FACE_OUTER_BOUND ( 'NONE', #13575, .T. ) ;
#21769=CARTESIAN_POINT ( 'NONE',  ( -141.6428522700808230, 69.54464929955099706, 80.00000000000001421 ) ) ;
#21776=ADVANCED_FACE ( 'NONE', ( #17326 ), #8437, .T. ) ;
#21777=DIRECTION ( 'NONE',  ( 1.000000000000000000, 0.000000000000000000, 0.000000000000000000 ) ) ;
#21785=ORIENTED_EDGE ( 'NONE', *, *, #21025, .F. ) ;
#21786=CARTESIAN_POINT ( 'NONE',  ( -219.9212092885508980, 137.1730549828704682, 15.11921763785538886 ) ) ;
#21792=DIRECTION ( 'NONE',  ( 1.000000000000000000, -0.000000000000000000, -0.000000000000000000 ) ) ;
#21796=CARTESIAN_POINT ( 'NONE',  ( -227.1514737387478817, 90.13265483295766956, -13.57967572479353180 ) ) ;
#21797=FACE_OUTER_BOUND ( 'NONE', #1451, .T. ) ;
#21801=FACE_OUTER_BOUND ( 'NONE', #14190, .T. ) ;
#21802=ORIENTED_EDGE ( 'NONE', *, *, #22266, .F. ) ;
#21809=VECTOR ( 'NONE', #11024, 1000.000000000000000 ) ;
#21811=CARTESIAN_POINT ( 'NONE',  ( 101.4665947576622216, 243.5985648160965980, -15.64809332290144006 ) ) ;
#21812=ORIENTED_EDGE ( 'NONE', *, *, #20240, .T. ) ;
#21815=EDGE_LOOP ( 'NONE', ( #10759, #15505, #12965, #2980 ) ) ;
#21816=ORIENTED_EDGE ( 'NONE', *, *, #7646, .T. ) ;
#21817=ORIENTED_EDGE ( 'NONE', *, *, #18787, .F. ) ;
#21825=VECTOR ( 'NONE', #9425, 1000.000000000000000 ) ;
#21827=CARTESIAN_POINT ( 'NONE',  ( -218.5620487852697522, 71.28382977987227775, 22.94473774458083071 ) ) ;
#21829=DIRECTION ( 'NONE',  ( 1.000000000000000000, 0.000000000000000000, 0.000000000000000000 ) ) ;
#21831=CARTESIAN_POINT ( 'NONE',  ( 39.99999999999995026, -3.469446951953624838E-15, 100.0000000000000142 ) ) ;
#21833=CARTESIAN_POINT ( 'NONE',  ( 79.99999999999991473, 140.0000000000000000, -45.00000000000000000 ) ) ;
#21837=CARTESIAN_POINT ( 'NONE',  ( -175.8417606860892874, 246.9430296707336652, -13.00000000000000000 ) ) ;
#21842=CARTESIAN_POINT ( 'NONE',  ( -162.7079589413399106, 119.3768178259787049, 22.14987655455460214 ) ) ;
#21850=FACE_OUTER_BOUND ( 'NONE', #5163, .T. ) ;
#21851=LINE ( 'NONE', #23717, #18645 ) ;
#21853=( BOUNDED_SURFACE ( )  B_SPLINE_SURFACE ( 3, 2, ( 
 ( #26888, #17693, #746 ),
 ( #22145, #22001, #15696 ),
 ( #7212, #322, #9076 ),
 ( #4464, #462, #13257 ),
 ( #7065, #11240, #26588 ),
 ( #24447, #2311, #24738 ),
 ( #22294, #15846, #11091 ),
 ( #26441, #22582, #24591 ),
 ( #24301, #4899, #13689 ),
 ( #20277, #9372, #3447 ) ),
 .UNSPECIFIED., .F., .F., .F. ) 
 B_SPLINE_SURFACE_WITH_KNOTS ( ( 4, 2, 2, 2, 4 ),
 ( 3, 3 ),
 ( 0.000000000000000000, 0.003993085574633944979, 0.007986171149267889957, 0.01197925672390183494, 0.01597234229853577991 ),
 ( 0.000000000000000000, 1.000000000000000000 ),
 .UNSPECIFIED. ) 
 GEOMETRIC_REPRESENTATION_ITEM ( )  RATIONAL_B_SPLINE_SURFACE ( (
 ( 1.000000000000000000, 0.7071067811865472397, 1.000000000000000000),
 ( 1.000000000000000000, 0.6986941146400569291, 1.000000000000000000),
 ( 1.000000000000000000, 0.6922065170621660712, 1.000000000000000000),
 ( 1.000000000000000000, 0.6834952607749176234, 1.000000000000000000),
 ( 1.000000000000000000, 0.6812778029564223736, 1.000000000000000000),
 ( 1.000000000000000000, 0.6812778029564223736, 1.000000000000000000),
 ( 1.000000000000000000, 0.6834952607775843791, 1.000000000000000000),
 ( 1.000000000000000000, 0.6922065170594993155, 1.000000000000000000),
 ( 1.000000000000000000, 0.6986941146420598825, 1.000000000000000000),
 ( 1.000000000000000000, 0.7071067811865472397, 1.000000000000000000) ) ) 
 REPRESENTATION_ITEM ( '' )  SURFACE ( )  );
#21854=CIRCLE ( 'NONE', #8087, 1.999999999999996669 ) ;
#21855=CARTESIAN_POINT ( 'NONE',  ( 107.3061218088456457, 127.3934823310315920, -100.0000000000216573 ) ) ;
#21857=VERTEX_POINT ( 'NONE', #26227 ) ;
#21858=CARTESIAN_POINT ( 'NONE',  ( -214.2130517962793590, 88.01573912158703195, 20.10369910981496844 ) ) ;
#21867=CARTESIAN_POINT ( 'NONE',  ( -156.2917263574996127, 178.8555734514394828, 12.99999999999999822 ) ) ;
#21869=FACE_BOUND ( 'NONE', #8271, .T. ) ;
#21870=ADVANCED_FACE ( 'NONE', ( #14617 ), #16900, .T. ) ;
#21877=CARTESIAN_POINT ( 'NONE',  ( -185.7285736283564006, 106.1028100233644125, -32.35901429591675083 ) ) ;
#21881=CARTESIAN_POINT ( 'NONE',  ( -111.1798965680916069, 69.38626228962301923, 82.93899756288178082 ) ) ;
#21884=ORIENTED_EDGE ( 'NONE', *, *, #24701, .T. ) ;
#21885=ORIENTED_EDGE ( 'NONE', *, *, #23823, .F. ) ;
#21886=CARTESIAN_POINT ( 'NONE',  ( -160.0000000000000284, 119.7660240611718763, 22.85081902853005431 ) ) ;
#21892=CARTESIAN_POINT ( 'NONE',  ( -209.8597496167328984, 64.07541194713586208, -30.05229862005789343 ) ) ;
#21894=ORIENTED_EDGE ( 'NONE', *, *, #24096, .F. ) ;
#21905=EDGE_CURVE ( 'NONE', #18951, #27397, #19850, .T. ) ;
#21913=CARTESIAN_POINT ( 'NONE',  ( -224.6762461164437354, 72.15359395014388610, 18.54889087295863348 ) ) ;
#21922=CARTESIAN_POINT ( 'NONE',  ( -229.2498027451139251, 132.0565166830976693, 15.00000000000000000 ) ) ;
#21923=CARTESIAN_POINT ( 'NONE',  ( 102.0697454929744907, 243.6045995028989068, 24.40655498896089171 ) ) ;
#21924=DIRECTION ( 'NONE',  ( -1.000000000000000000, 0.000000000000000000, 0.000000000000000000 ) ) ;
#21925=CARTESIAN_POINT ( 'NONE',  ( -40.40953891503691153, 0.000000000000000000, 99.00000000000000000 ) ) ;
#21929=CARTESIAN_POINT ( 'NONE',  ( -210.0000000000000284, -3.238150488490040751E-14, -70.00000000000001421 ) ) ;
#21930=FACE_OUTER_BOUND ( 'NONE', #1532, .T. ) ;
#21940=AXIS2_PLACEMENT_3D ( 'NONE', #26779, #24771, #7245 ) ;
#21945=CARTESIAN_POINT ( 'NONE',  ( 108.4669391322105412, 252.2354088788440549, -31.48703123558458472 ) ) ;
#21950=CIRCLE ( 'NONE', #4985, 10.00000000000000888 ) ;
#21953=ORIENTED_EDGE ( 'NONE', *, *, #7790, .T. ) ;
#21954=PLANE ( 'NONE',  #18245 ) ;
#21955=VECTOR ( 'NONE', #22366, 1000.000000000000000 ) ;
#21956=CIRCLE ( 'NONE', #19212, 30.00000000000000000 ) ;
#21959=CARTESIAN_POINT ( 'NONE',  ( -214.0383293111055139, 72.11341309493462859, 27.85175881924721608 ) ) ;
#21963=CYLINDRICAL_SURFACE ( 'NONE', #11303, 9.999999999999991118 ) ;
#21964=DIRECTION ( 'NONE',  ( -0.000000000000000000, -1.000000000000000000, -0.000000000000000000 ) ) ;
#21966=CARTESIAN_POINT ( 'NONE',  ( -232.6118856788241374, 77.06315004911816402, -15.48856666946770311 ) ) ;
#21968=CARTESIAN_POINT ( 'NONE',  ( -33.73595832852618059, 129.3982092947608749, 15.58051948656918562 ) ) ;
#21969=CARTESIAN_POINT ( 'NONE',  ( -140.1213116003368668, 122.5384136796733827, -15.00000000000000000 ) ) ;
#21976=EDGE_CURVE ( 'NONE', #26678, #26198, #5811, .T. ) ;
#21979=CARTESIAN_POINT ( 'NONE',  ( -203.1779787704217313, 93.05164332230199875, -28.77272332722132830 ) ) ;
#21984=CARTESIAN_POINT ( 'NONE',  ( -17.24491960465745777, -18.01420295945611727, 95.00000000000000000 ) ) ;
#21987=CARTESIAN_POINT ( 'NONE',  ( 81.45493510946427307, 110.0000000030975400, -100.0000000000000142 ) ) ;
#21992=ORIENTED_EDGE ( 'NONE', *, *, #16273, .T. ) ;
#21993=CARTESIAN_POINT ( 'NONE',  ( -227.1040115265393524, 87.91506694670529498, 15.89722369506078437 ) ) ;
#22001=CARTESIAN_POINT ( 'NONE',  ( -226.9034654752796314, 131.5715075451946348, -15.04814241297669319 ) ) ;
#22003=PLANE ( 'NONE',  #18550 ) ;
#22004=ORIENTED_EDGE ( 'NONE', *, *, #15000, .F. ) ;
#22005=DIRECTION ( 'NONE',  ( 1.000000000000000000, 0.000000000000000000, 0.000000000000000000 ) ) ;
#22015=AXIS2_PLACEMENT_3D ( 'NONE', #15890, #8978, #22335 ) ;
#22016=DIRECTION ( 'NONE',  ( 1.000000000000000000, 0.000000000000000000, 0.000000000000000000 ) ) ;
#22017=CARTESIAN_POINT ( 'NONE',  ( -185.2631373304065789, 106.4084716055997291, -32.26645048881131572 ) ) ;
#22023=EDGE_LOOP ( 'NONE', ( #10580, #14613, #11797 ) ) ;
#22028=AXIS2_PLACEMENT_3D ( 'NONE', #4822, #28370, #20200 ) ;
#22029=CARTESIAN_POINT ( 'NONE',  ( 39.99999999999995026, -19.99999999999983302, 100.0000000000000142 ) ) ;
#22031=FACE_OUTER_BOUND ( 'NONE', #13659, .T. ) ;
#22041=DIRECTION ( 'NONE',  ( 1.000000000000000000, 2.602085213965211135E-16, -0.000000000000000000 ) ) ;
#22042=ORIENTED_EDGE ( 'NONE', *, *, #22889, .T. ) ;
#22043=CARTESIAN_POINT ( 'NONE',  ( -212.8228108689316969, 60.01962377528477077, 15.18702394368705733 ) ) ;
#22047=DIRECTION ( 'NONE',  ( 0.8153095126952236704, -0.5790253867566402812, 0.000000000000000000 ) ) ;
#22048=ORIENTED_EDGE ( 'NONE', *, *, #1641, .F. ) ;
#22053=CIRCLE ( 'NONE', #6446, 429.0408555545579929 ) ;
#22057=EDGE_LOOP ( 'NONE', ( #10636, #24748, #8572, #17002 ) ) ;
#22064=CARTESIAN_POINT ( 'NONE',  ( -228.3260894844903532, 133.0445070941187851, 15.00000000000000000 ) ) ;
#22065=EDGE_CURVE ( 'NONE', #17181, #27481, #28053, .T. ) ;
#22066=CARTESIAN_POINT ( 'NONE',  ( 92.49170488790998945, 239.7529794472745834, 17.61766721976643879 ) ) ;
#22067=ADVANCED_FACE ( 'NONE', ( #1914 ), #9778, .T. ) ;
#22077=CARTESIAN_POINT ( 'NONE',  ( -143.6428522700808230, 80.49308115506423178, 248.5795775865965993 ) ) ;
#22083=DIRECTION ( 'NONE',  ( 1.000000000000000000, 0.000000000000000000, 0.000000000000000000 ) ) ;
#22087=CARTESIAN_POINT ( 'NONE',  ( 109.2338094452045425, 254.3984564254963630, -35.27666983503028320 ) ) ;
#22091=VERTEX_POINT ( 'NONE', #16874 ) ;
#22100=CIRCLE ( 'NONE', #4185, 21.59849023212046149 ) ;
#22101=B_SPLINE_CURVE_WITH_KNOTS ( 'NONE', 3,
 ( #9423, #24787, #22775, #5094, #25068, #11864, #5379, #14158, #22910, #3217, #12003, #11589, #20327, #1071, #9839, #18597, #27345, #25200, #14297, #23051, #3359, #8388, #21591, #25612, #25899, #28184, #27764, #10261 ),
 .UNSPECIFIED., .F., .F.,
 ( 4, 2, 2, 2, 2, 2, 2, 2, 2, 2, 2, 2, 2, 4 ),
 ( 0.000000000000000000, 0.01499785927852794604, 0.02999571855705591289, 0.03749464819631988938, 0.04124411301595189844, 0.04499357783558391444, 0.05999143711411201313, 0.07498929639264009794, 0.08998715567116818970, 0.09373662049080021264, 0.09748608531043220782, 0.1049850149496963231, 0.1124839445889604245, 0.1199828742282245259 ),
 .UNSPECIFIED. ) ;
#22105=CARTESIAN_POINT ( 'NONE',  ( -199.5809478526699650, 61.42778479158862126, 28.44561038856815927 ) ) ;
#22108=FACE_OUTER_BOUND ( 'NONE', #9707, .T. ) ;
#22109=DIRECTION ( 'NONE',  ( 1.000000000000000000, 0.000000000000000000, 0.000000000000000000 ) ) ;
#22113=CARTESIAN_POINT ( 'NONE',  ( 0.6954374052207565882, 136.6090791541018632, 13.39223910979635690 ) ) ;
#22114=CARTESIAN_POINT ( 'NONE',  ( -138.6428522700808230, 66.54464929955099706, 83.00000000000001421 ) ) ;
#22116=CARTESIAN_POINT ( 'NONE',  ( -200.0000000000000284, -91.18033988749901653, -21.20097097723064294 ) ) ;
#22121=CARTESIAN_POINT ( 'NONE',  ( -160.8326600028555902, 120.2355194873574931, 21.37420696376537776 ) ) ;
#22122=CARTESIAN_POINT ( 'NONE',  ( -205.8155715011940288, 91.09379270857378685, -26.99297343021914131 ) ) ;
#22125=ORIENTED_EDGE ( 'NONE', *, *, #16841, .F. ) ;
#22126=EDGE_CURVE ( 'NONE', #16598, #18699, #3230, .T. ) ;
#22127=CARTESIAN_POINT ( 'NONE',  ( -40.40953891503691153, 0.000000000000000000, 100.0000000000000000 ) ) ;
#22128=CARTESIAN_POINT ( 'NONE',  ( -127.7167972290761071, 131.6999243923856397, 16.10307571226574197 ) ) ;
#22131=CYLINDRICAL_SURFACE ( 'NONE', #9976, 29.99999999999999645 ) ;
#22132=AXIS2_PLACEMENT_3D ( 'NONE', #4305, #2144, #6739 ) ;
#22135=ORIENTED_EDGE ( 'NONE', *, *, #8809, .T. ) ;
#22136=CARTESIAN_POINT ( 'NONE',  ( -207.8784783882069860, 89.22626204389251825, 26.87087741168311084 ) ) ;
#22137=TOROIDAL_SURFACE ( 'NONE', #15712, 33.76444293738737912, 9.999999999999996447 ) ;
#22139=CIRCLE ( 'NONE', #16192, 32.49120955644046660 ) ;
#22140=EDGE_CURVE ( 'NONE', #1515, #9431, #11409, .T. ) ;
#22145=CARTESIAN_POINT ( 'NONE',  ( -228.3260894844903817, 133.0445070941187851, -15.00000000000000178 ) ) ;
#22147=FACE_OUTER_BOUND ( 'NONE', #21527, .T. ) ;
#22149=EDGE_CURVE ( 'NONE', #23617, #10961, #26742, .T. ) ;
#22151=DIRECTION ( 'NONE',  ( -0.000000000000000000, -0.000000000000000000, -1.000000000000000000 ) ) ;
#22155=EDGE_LOOP ( 'NONE', ( #1863, #26804, #15500, #13891 ) ) ;
#22157=ORIENTED_EDGE ( 'NONE', *, *, #5498, .T. ) ;
#22159=EDGE_CURVE ( 'NONE', #18799, #15830, #8397, .T. ) ;
#22161=CARTESIAN_POINT ( 'NONE',  ( -201.7173803564383263, 94.30285377706006500, -30.02230663004699451 ) ) ;
#22168=VERTEX_POINT ( 'NONE', #21886 ) ;
#22169=CIRCLE ( 'NONE', #16680, 9.999999999999996447 ) ;
#22171=EDGE_CURVE ( 'NONE', #25311, #22340, #3816, .T. ) ;
#22172=AXIS2_PLACEMENT_3D ( 'NONE', #26747, #17555, #4615 ) ;
#22174=DIRECTION ( 'NONE',  ( -0.000000000000000000, -0.000000000000000000, 1.000000000000000000 ) ) ;
#22177=CIRCLE ( 'NONE', #4277, 30.00000000000000000 ) ;
#22181=ORIENTED_EDGE ( 'NONE', *, *, #20931, .T. ) ;
#22187=EDGE_CURVE ( 'NONE', #18495, #11369, #28330, .T. ) ;
#22200=ORIENTED_EDGE ( 'NONE', *, *, #18471, .F. ) ;
#22204=CIRCLE ( 'NONE', #7971, 3.532530335305414493 ) ;
#22210=CARTESIAN_POINT ( 'NONE',  ( 95.55652878161114927, 240.7834791927029983, 9.443977278918188389 ) ) ;
#22213=AXIS2_PLACEMENT_3D ( 'NONE', #22684, #18230, #16223 ) ;
#22216=DIRECTION ( 'NONE',  ( -1.000000000000000000, 0.000000000000000000, 0.000000000000000000 ) ) ;
#22228=ADVANCED_FACE ( 'NONE', ( #26767, #15868, #24616, #8678, #13710 ), #10834, .T. ) ;
#22233=CARTESIAN_POINT ( 'NONE',  ( -23.16361609519321973, 129.3663660641504407, -15.59648484705163796 ) ) ;
#22235=AXIS2_PLACEMENT_3D ( 'NONE', #15121, #16706, #27741 ) ;
#22246=CARTESIAN_POINT ( 'NONE',  ( -219.7112380651049364, 60.27397245185820651, 23.81555219817632008 ) ) ;
#22256=CARTESIAN_POINT ( 'NONE',  ( -0.3498732073529682296, 134.1707435274499005, 15.55713657458744947 ) ) ;
#22257=CARTESIAN_POINT ( 'NONE',  ( -209.9870476429693156, 61.15597564521014817, 23.95642062441354625 ) ) ;
#22259=EDGE_CURVE ( 'NONE', #22407, #24933, #23549, .T. ) ;
#22263=ORIENTED_EDGE ( 'NONE', *, *, #6970, .F. ) ;
#22266=EDGE_CURVE ( 'NONE', #17545, #2342, #11702, .T. ) ;
#22269=CARTESIAN_POINT ( 'NONE',  ( -204.4655292202942292, 92.00796242303097472, -28.73370588204663889 ) ) ;
#22274=CARTESIAN_POINT ( 'NONE',  ( -133.4910656777217355, 128.8270384526469172, 17.15628984000436219 ) ) ;
#22275=ORIENTED_EDGE ( 'NONE', *, *, #5878, .T. ) ;
#22278=VECTOR ( 'NONE', #3394, 1000.000000000000000 ) ;
#22279=DIRECTION ( 'NONE',  ( 1.000000000000000000, 0.000000000000000000, 0.000000000000000000 ) ) ;
#22280=CARTESIAN_POINT ( 'NONE',  ( -40.40953891503691153, 0.000000000000000000, 99.00000000000000000 ) ) ;
#22283=CIRCLE ( 'NONE', #25033, 2.000000000000012879 ) ;
#22287=CARTESIAN_POINT ( 'NONE',  ( -220.5757601432208617, 60.53190028573507675, -22.93231238515986092 ) ) ;
#22292=ADVANCED_FACE ( 'NONE', ( #3330 ), #11560, .F. ) ;
#22294=CARTESIAN_POINT ( 'NONE',  ( -221.1044245926502185, 138.9463871349811939, -14.97905406095822656 ) ) ;
#22295=DIRECTION ( 'NONE',  ( 0.000000000000000000, 1.000000000000000000, -0.000000000000000000 ) ) ;
#22296=ORIENTED_EDGE ( 'NONE', *, *, #16385, .F. ) ;
#22300=CARTESIAN_POINT ( 'NONE',  ( -180.0000000000000284, -40.00000000000004974, 70.00000000000001421 ) ) ;
#22301=CARTESIAN_POINT ( 'NONE',  ( -141.1970735032543303, 70.84982942354511692, 82.84771202320575867 ) ) ;
#22305=ORIENTED_EDGE ( 'NONE', *, *, #18568, .T. ) ;
#22306=EDGE_CURVE ( 'NONE', #1362, #15527, #27046, .T. ) ;
#22307=DIRECTION ( 'NONE',  ( -1.541976423090495387E-16, 1.000000000000000000, 0.000000000000000000 ) ) ;
#22308=LINE ( 'NONE', #11829, #6231 ) ;
#22309=ORIENTED_EDGE ( 'NONE', *, *, #14984, .T. ) ;
#22317=CARTESIAN_POINT ( 'NONE',  ( -31.67953875179438228, 128.0283279034048007, 17.49215224234154675 ) ) ;
#22320=CARTESIAN_POINT ( 'NONE',  ( -31.66438925218564293, 128.0276125918315131, -17.49246453772925847 ) ) ;
#22323=FACE_OUTER_BOUND ( 'NONE', #12387, .T. ) ;
#22324=CYLINDRICAL_SURFACE ( 'NONE', #18883, 19.07743405327024888 ) ;
#22329=CARTESIAN_POINT ( 'NONE',  ( -12.24491960465745599, -23.01420295945612082, 95.00000000000000000 ) ) ;
#22330=DIRECTION ( 'NONE',  ( -0.000000000000000000, -0.000000000000000000, 1.000000000000000000 ) ) ;
#22331=VERTEX_POINT ( 'NONE', #9396 ) ;
#22332=CARTESIAN_POINT ( 'NONE',  ( -218.0684950290401787, 60.60891383183042080, 12.02124378490089285 ) ) ;
#22333=VERTEX_POINT ( 'NONE', #22881 ) ;
#22335=DIRECTION ( 'NONE',  ( 0.000000000000000000, 0.000000000000000000, -1.000000000000000000 ) ) ;
#22340=VERTEX_POINT ( 'NONE', #3189 ) ;
#22341=AXIS2_PLACEMENT_3D ( 'NONE', #625, #18424, #9390 ) ;
#22342=EDGE_CURVE ( 'NONE', #23124, #27860, #11978, .T. ) ;
#22343=CARTESIAN_POINT ( 'NONE',  ( -215.1490939589890274, 71.74855184469089409, 26.39437962326677578 ) ) ;
#22346=CARTESIAN_POINT ( 'NONE',  ( -17.24491960465746132, 75.97823757117562593, 95.00000000000000000 ) ) ;
#22349=LINE ( 'NONE', #27629, #19564 ) ;
#22351=EDGE_LOOP ( 'NONE', ( #320, #26109, #14286, #19817 ) ) ;
#22353=EDGE_CURVE ( 'NONE', #24201, #11803, #16665, .T. ) ;
#22354=CARTESIAN_POINT ( 'NONE',  ( 106.3805259670891559, 243.6561646000983785, 30.69292865458877273 ) ) ;
#22355=B_SPLINE_CURVE_WITH_KNOTS ( 'NONE', 3,
 ( #5264, #14049, #22799, #3097, #11891, #25223, #26063, #17166, #8555, #17023, #13020, #1514, #12732, #27923, #25779, #10848, #8270, #4088, #28066, #26203, #10564, #19605, #12594, #14738 ),
 .UNSPECIFIED., .F., .F.,
 ( 4, 2, 2, 2, 2, 2, 2, 2, 2, 2, 2, 4 ),
 ( 0.006955041467238867736, 0.01003080572916798148, 0.01156868786013253748, 0.01310656999109709522, 0.01618233425302619682, 0.01772021638399075283, 0.01925809851495530883, 0.02233386277688433411, 0.02387174490784884848, 0.02540962703881335938, 0.02848539130074245404, 0.03156115556267154870 ),
 .UNSPECIFIED. ) ;
#22358=AXIS2_PLACEMENT_3D ( 'NONE', #1315, #25578, #25164 ) ;
#22360=DIRECTION ( 'NONE',  ( 1.000000000000000000, 0.000000000000000000, 0.000000000000000000 ) ) ;
#22362=DIRECTION ( 'NONE',  ( 0.000000000000000000, -0.000000000000000000, -1.000000000000000000 ) ) ;
#22365=LINE ( 'NONE', #2672, #17492 ) ;
#22366=DIRECTION ( 'NONE',  ( -1.000000000000000000, -0.000000000000000000, -0.000000000000000000 ) ) ;
#22369=CARTESIAN_POINT ( 'NONE',  ( 89.99999999999988631, 240.0000000000000284, 6.270166537925822681 ) ) ;
#22377=EDGE_LOOP ( 'NONE', ( #27383, #5501, #16285, #19518, #10928, #26714, #5562, #27136 ) ) ;
#22381=ORIENTED_EDGE ( 'NONE', *, *, #19549, .F. ) ;
#22383=VERTEX_POINT ( 'NONE', #1878 ) ;
#22387=FACE_BOUND ( 'NONE', #25970, .T. ) ;
#22388=ADVANCED_FACE ( 'NONE', ( #12264 ), #3752, .T. ) ;
#22389=DIRECTION ( 'NONE',  ( 0.000000000000000000, 0.000000000000000000, 1.000000000000000000 ) ) ;
#22390=EDGE_CURVE ( 'NONE', #17645, #12991, #6058, .T. ) ;
#22391=CARTESIAN_POINT ( 'NONE',  ( -228.3003245610658496, 63.46411924056219789, 17.58993856060416405 ) ) ;
#22394=DIRECTION ( 'NONE',  ( 1.000000000000000000, 0.000000000000000000, 0.000000000000000000 ) ) ;
#22395=CARTESIAN_POINT ( 'NONE',  ( -3.642919299551294898E-14, 139.9999999999999716, -45.00000000000000000 ) ) ;
#22399=CARTESIAN_POINT ( 'NONE',  ( -42.99650729631200363, 71.03850157808263077, 99.00000000000000000 ) ) ;
#22402=LINE ( 'NONE', #11502, #23802 ) ;
#22403=DIRECTION ( 'NONE',  ( -0.000000000000000000, 1.000000000000000000, 0.000000000000000000 ) ) ;
#22407=VERTEX_POINT ( 'NONE', #14837 ) ;
#22408=DIRECTION ( 'NONE',  ( 0.000000000000000000, 1.000000000000000000, 0.000000000000000000 ) ) ;
#22417=CIRCLE ( 'NONE', #16917, 18.91107291867258411 ) ;
#22419=VERTEX_POINT ( 'NONE', #18847 ) ;
#22421=CARTESIAN_POINT ( 'NONE',  ( 134.9999999999998579, 220.0000000000000284, 90.00000000000002842 ) ) ;
#22424=CARTESIAN_POINT ( 'NONE',  ( -206.1401686320352837, 90.30263034637913222, 28.11534395024635558 ) ) ;
#22427=CONICAL_SURFACE ( 'NONE', #26530, 6.025000000000002132, 0.7853981633974482790 ) ;
#22429=CARTESIAN_POINT ( 'NONE',  ( -187.8924994060663494, 156.4650759647683742, -15.00000000000000000 ) ) ;
#22431=CARTESIAN_POINT ( 'NONE',  ( -208.8418814728804023, 74.65865074066952900, -37.27912060900214186 ) ) ;
#22433=EDGE_LOOP ( 'NONE', ( #2864, #24181, #16515, #7751 ) ) ;
#22435=AXIS2_PLACEMENT_3D ( 'NONE', #12236, #1430, #8045 ) ;
#22438=DIRECTION ( 'NONE',  ( -0.000000000000000000, -0.000000000000000000, 1.000000000000000000 ) ) ;
#22439=ORIENTED_EDGE ( 'NONE', *, *, #24297, .F. ) ;
#22441=CARTESIAN_POINT ( 'NONE',  ( -233.4632575733469650, 77.89441575049642097, 15.30815287833161342 ) ) ;
#22445=EDGE_LOOP ( 'NONE', ( #16075, #20962, #25714 ) ) ;
#22449=ORIENTED_EDGE ( 'NONE', *, *, #15720, .T. ) ;
#22453=AXIS2_PLACEMENT_3D ( 'NONE', #25540, #21090, #1270 ) ;
#22459=CARTESIAN_POINT ( 'NONE',  ( -6.823563161442123715, 131.5377459308396055, 16.21528367945318649 ) ) ;
#22460=CIRCLE ( 'NONE', #10074, 3.532530335305414493 ) ;
#22461=ADVANCED_FACE ( 'NONE', ( #17121 ), #6201, .F. ) ;
#22462=EDGE_CURVE ( 'NONE', #24936, #17385, #22169, .T. ) ;
#22464=DIRECTION ( 'NONE',  ( -0.000000000000000000, 1.000000000000000000, -0.000000000000000000 ) ) ;
#22465=CARTESIAN_POINT ( 'NONE',  ( -23.58081250372386251, 128.1194696888447311, -17.45268724460935061 ) ) ;
#22466=CARTESIAN_POINT ( 'NONE',  ( -124.9781469243918934, 222.2250949724356985, 5.000000000000002665 ) ) ;
#22467=DIRECTION ( 'NONE',  ( -0.5555587585212703461, -0.8314772792026879911, 1.927481641382755247E-15 ) ) ;
#22468=CARTESIAN_POINT ( 'NONE',  ( 134.9999999999998579, 220.0000000000000284, 84.99999999999995737 ) ) ;
#22472=DIRECTION ( 'NONE',  ( 0.000000000000000000, -1.000000000000000000, 0.000000000000000000 ) ) ;
#22476=CARTESIAN_POINT ( 'NONE',  ( 65.00000000000000000, -120.0000000000000711, 63.97500000000001563 ) ) ;
#22477=AXIS2_PLACEMENT_3D ( 'NONE', #18067, #4687, #13474 ) ;
#22480=DIRECTION ( 'NONE',  ( 0.000000000000000000, 0.000000000000000000, -1.000000000000000000 ) ) ;
#22481=CARTESIAN_POINT ( 'NONE',  ( -210.0000000000000284, -3.238150488490040751E-14, 100.0000000000000142 ) ) ;
#22483=( NAMED_UNIT ( * ) PLANE_ANGLE_UNIT ( ) SI_UNIT ( $, .RADIAN. ) );
#22487=ORIENTED_EDGE ( 'NONE', *, *, #6265, .T. ) ;
#22489=ORIENTED_EDGE ( 'NONE', *, *, #52, .T. ) ;
#22494=ADVANCED_FACE ( 'NONE', ( #1604 ), #25392, .T. ) ;
#22495=VECTOR ( 'NONE', #27358, 1000.000000000000000 ) ;
#22497=B_SPLINE_CURVE_WITH_KNOTS ( 'NONE', 3,
 ( #26895, #8941, #11247, #9085, #13697, #15559, #9230, #22301, #17842, #15422, #2462, #17700, #15704, #328 ),
 .UNSPECIFIED., .F., .F.,
 ( 4, 2, 2, 2, 2, 2, 4 ),
 ( 0.000000000000000000, 0.001449387442315872411, 0.002174081163473810027, 0.002898774884631747425, 0.003623468605789684823, 0.004348162326947622655, 0.005797549769263428930 ),
 .UNSPECIFIED. ) ;
#22499=CARTESIAN_POINT ( 'NONE',  ( 107.7348956500412100, 246.7603209947075982, 33.46154240484374043 ) ) ;
#22509=CARTESIAN_POINT ( 'NONE',  ( 134.9999999999998579, 220.0000000000000284, -105.0000000000000284 ) ) ;
#22514=ORIENTED_EDGE ( 'NONE', *, *, #12455, .F. ) ;
#22520=ORIENTED_EDGE ( 'NONE', *, *, #946, .T. ) ;
#22523=CARTESIAN_POINT ( 'NONE',  ( 109.9999999999998863, 259.2933449741933032, -44.14322629332889392 ) ) ;
#22524=EDGE_LOOP ( 'NONE', ( #13958, #6649, #27450, #6780 ) ) ;
#22531=CARTESIAN_POINT ( 'NONE',  ( -134.0122209785728273, 130.0131674746676538, 15.29879588572737426 ) ) ;
#22534=CARTESIAN_POINT ( 'NONE',  ( -100.3750459336811787, 135.9165849456836384, -15.23352683708864141 ) ) ;
#22538=CARTESIAN_POINT ( 'NONE',  ( -194.2306746384193730, 63.21821459927384979, 44.70951427402087575 ) ) ;
#22541=EDGE_CURVE ( 'NONE', #21665, #13456, #4459, .T. ) ;
#22542=DIRECTION ( 'NONE',  ( 0.000000000000000000, 0.000000000000000000, 1.000000000000000000 ) ) ;
#22543=CARTESIAN_POINT ( 'NONE',  ( -231.9378824387731299, 93.53122965655668963, -13.00000000000000000 ) ) ;
#22544=CARTESIAN_POINT ( 'NONE',  ( -68.57415822541635464, 29.64876300893806516, 95.00000000000000000 ) ) ;
#22547=CARTESIAN_POINT ( 'NONE',  ( 1.671497233361736612, 135.1829325683629577, 15.36772416567834476 ) ) ;
#22553=ADVANCED_FACE ( 'NONE', ( #11377 ), #3362, .F. ) ;
#22554=CARTESIAN_POINT ( 'NONE',  ( -146.6428522700808230, 22.24192588826928585, 83.00000000000001421 ) ) ;
#22564=CARTESIAN_POINT ( 'NONE',  ( -141.8785761468075464, 126.4564228109756101, 18.21987071921232371 ) ) ;
#22570=LINE ( 'NONE', #14239, #16941 ) ;
#22571=ORIENTED_EDGE ( 'NONE', *, *, #16385, .T. ) ;
#22572=CARTESIAN_POINT ( 'NONE',  ( -204.2340599944510586, 92.18449363278668329, 28.15791701117214529 ) ) ;
#22574=AXIS2_PLACEMENT_3D ( 'NONE', #9257, #8825, #26342 ) ;
#22579=CARTESIAN_POINT ( 'NONE',  ( -215.5934637701523684, 59.01440814108518396, -29.65465734991407132 ) ) ;
#22581=LINE ( 'NONE', #2891, #7300 ) ;
#22582=CARTESIAN_POINT ( 'NONE',  ( -217.7546030100656083, 138.5587306369264411, -15.07876772301851354 ) ) ;
#22589=EDGE_LOOP ( 'NONE', ( #7506, #726, #27353, #27508 ) ) ;
#22592=CIRCLE ( 'NONE', #20356, 30.00000000000000000 ) ;
#22596=DIRECTION ( 'NONE',  ( -0.000000000000000000, 0.000000000000000000, 1.000000000000000000 ) ) ;
#22598=ORIENTED_EDGE ( 'NONE', *, *, #2429, .F. ) ;
#22599=LINE ( 'NONE', #9669, #9031 ) ;
#22611=CARTESIAN_POINT ( 'NONE',  ( -23.11731384102234443, 129.3701763555853859, -16.91551946832288422 ) ) ;
#22612=DIRECTION ( 'NONE',  ( -0.000000000000000000, 1.000000000000000000, -1.387778780781445429E-16 ) ) ;
#22615=DIRECTION ( 'NONE',  ( 1.000000000000000000, 0.000000000000000000, 0.000000000000000000 ) ) ;
#22617=AXIS2_PLACEMENT_3D ( 'NONE', #27134, #4869, #7470 ) ;
#22621=CIRCLE ( 'NONE', #23989, 41.00000000000000000 ) ;
#22623=DIRECTION ( 'NONE',  ( 0.000000000000000000, 0.000000000000000000, -1.000000000000000000 ) ) ;
#22626=AXIS2_PLACEMENT_3D ( 'NONE', #1524, #14751, #10575 ) ;
#22628=FACE_OUTER_BOUND ( 'NONE', #6006, .T. ) ;
#22629=CARTESIAN_POINT ( 'NONE',  ( -235.5935699371920293, 67.74125567661748448, -5.863186529791158286 ) ) ;
#22634=ORIENTED_EDGE ( 'NONE', *, *, #11680, .F. ) ;
#22636=DIRECTION ( 'NONE',  ( 0.000000000000000000, 1.000000000000000000, -1.224646799147353207E-16 ) ) ;
#22641=AXIS2_PLACEMENT_3D ( 'NONE', #12544, #21567, #1323 ) ;
#22654=FACE_OUTER_BOUND ( 'NONE', #2831, .T. ) ;
#22659=ORIENTED_EDGE ( 'NONE', *, *, #149, .F. ) ;
#22663=AXIS2_PLACEMENT_3D ( 'NONE', #764, #1038, #27180 ) ;
#22666=DIRECTION ( 'NONE',  ( 1.000000000000000000, 1.927605262034834208E-15, 0.000000000000000000 ) ) ;
#22671=EDGE_CURVE ( 'NONE', #18983, #5384, #11187, .T. ) ;
#22675=ORIENTED_EDGE ( 'NONE', *, *, #24701, .F. ) ;
#22679=VECTOR ( 'NONE', #22464, 1000.000000000000000 ) ;
#22682=CARTESIAN_POINT ( 'NONE',  ( -67.66675424875249689, 133.9296644792104871, -15.61820326278706972 ) ) ;
#22683=VECTOR ( 'NONE', #22623, 1000.000000000000000 ) ;
#22684=CARTESIAN_POINT ( 'NONE',  ( -200.0000000000000284, -91.18033988749901653, 0.000000000000000000 ) ) ;
#22691=DIRECTION ( 'NONE',  ( 0.000000000000000000, 0.000000000000000000, -1.000000000000000000 ) ) ;
#22692=CARTESIAN_POINT ( 'NONE',  ( 104.1118574119297762, 122.0584436052485700, 84.84374999969743669 ) ) ;
#22695=CARTESIAN_POINT ( 'NONE',  ( -181.4803588069671036, 108.8061799861145431, 31.29209452200661801 ) ) ;
#22697=EDGE_LOOP ( 'NONE', ( #820, #16663, #294, #18637 ) ) ;
#22700=CARTESIAN_POINT ( 'NONE',  ( -207.6601984805002132, 89.35148749558611314, -27.03156250143107897 ) ) ;
#22701=FACE_OUTER_BOUND ( 'NONE', #21450, .T. ) ;
#22708=CARTESIAN_POINT ( 'NONE',  ( 0.000000000000000000, 330.0000000000000000, -100.0000000000000142 ) ) ;
#22711=CARTESIAN_POINT ( 'NONE',  ( 109.9999999999999005, 240.0000000000000284, -45.00000000000000000 ) ) ;
#22712=CARTESIAN_POINT ( 'NONE',  ( -68.57415822541635464, 75.97823757117562593, 95.00000000000000000 ) ) ;
#22720=CARTESIAN_POINT ( 'NONE',  ( -160.0000000000000284, 109.9999999999999432, 70.00000000000001421 ) ) ;
#22721=CARTESIAN_POINT ( 'NONE',  ( -205.1716483941798401, 60.34345434848681577, -21.58965668827011442 ) ) ;
#22722=CARTESIAN_POINT ( 'NONE',  ( 3.469446951953618133E-15, -50.00000000000004263, 98.28427124746191623 ) ) ;
#22723=EDGE_CURVE ( 'NONE', #970, #2675, #739, .T. ) ;
#22729=CARTESIAN_POINT ( 'NONE',  ( -237.0233935005625767, 68.72940251376630272, 14.95240471282495598 ) ) ;
#22736=DIRECTION ( 'NONE',  ( 0.000000000000000000, 0.000000000000000000, 1.000000000000000000 ) ) ;
#22738=AXIS2_PLACEMENT_3D ( 'NONE', #9326, #9612, #18232 ) ;
#22739=AXIS2_PLACEMENT_3D ( 'NONE', #27856, #8197, #16961 ) ;
#22740=ORIENTED_EDGE ( 'NONE', *, *, #24461, .F. ) ;
#22741=DIRECTION ( 'NONE',  ( 0.000000000000000000, 0.000000000000000000, 1.000000000000000000 ) ) ;
#22745=PLANE ( 'NONE',  #18337 ) ;
#22746=ORIENTED_EDGE ( 'NONE', *, *, #24082, .T. ) ;
#22750=CARTESIAN_POINT ( 'NONE',  ( -216.4421519707229606, 141.6000904446840991, 13.00000000000000000 ) ) ;
#22751=CARTESIAN_POINT ( 'NONE',  ( -18.04820575590032661, 129.9789000731339570, -16.68755046163289535 ) ) ;
#22758=DIRECTION ( 'NONE',  ( -1.000000000000000000, 6.752478448789676648E-18, 0.000000000000000000 ) ) ;
#22763=CARTESIAN_POINT ( 'NONE',  ( -17.24491960465745777, 29.64876300893806516, 95.00000000000000000 ) ) ;
#22764=LINE ( 'NONE', #7809, #5218 ) ;
#22766=DIRECTION ( 'NONE',  ( 8.659560562354934091E-17, 0.7071067811865474617, -0.7071067811865476838 ) ) ;
#22768=FACE_OUTER_BOUND ( 'NONE', #11406, .T. ) ;
#22773=CARTESIAN_POINT ( 'NONE',  ( 22.58950924271104910, 154.2349915562422780, 15.00000000000000000 ) ) ;
#22775=CARTESIAN_POINT ( 'NONE',  ( -52.81561984911300556, 131.8400808202090957, 16.12034709971533886 ) ) ;
#22776=CARTESIAN_POINT ( 'NONE',  ( 98.49257838773085894, 241.8754478897298839, 12.06630627437291992 ) ) ;
#22783=( BOUNDED_CURVE ( )  B_SPLINE_CURVE ( 2, ( #25045, #16564, #18711 ),
 .UNSPECIFIED., .F., .F. ) 
 B_SPLINE_CURVE_WITH_KNOTS ( ( 3, 3 ),
 ( 0.000000000000000000, 1.000000000000000000 ),
 .UNSPECIFIED. ) 
 CURVE ( )  GEOMETRIC_REPRESENTATION_ITEM ( )  RATIONAL_B_SPLINE_CURVE ( ( 1.000000000000000000, 0.7071067811865484609, 1.000000000000000000 ) ) 
 REPRESENTATION_ITEM ( '' )  );
#22784=ORIENTED_EDGE ( 'NONE', *, *, #24127, .F. ) ;
#22786=DIRECTION ( 'NONE',  ( 0.000000000000000000, 0.000000000000000000, 1.000000000000000000 ) ) ;
#22787=EDGE_CURVE ( 'NONE', #24673, #17712, #26176, .T. ) ;
#22791=CARTESIAN_POINT ( 'NONE',  ( 82.68942924499074820, 110.0997128786250840, -70.07812500014861712 ) ) ;
#22793=DIRECTION ( 'NONE',  ( -0.000000000000000000, 0.000000000000000000, 1.000000000000000000 ) ) ;
#22797=DIRECTION ( 'NONE',  ( -1.000000000000000000, 0.000000000000000000, 0.000000000000000000 ) ) ;
#22799=CARTESIAN_POINT ( 'NONE',  ( 114.6895484223570918, 210.2681915721689450, -98.48649515991441206 ) ) ;
#22801=ORIENTED_EDGE ( 'NONE', *, *, #7625, .T. ) ;
#22805=B_SPLINE_CURVE_WITH_KNOTS ( 'NONE', 3,
 ( #20661, #846, #5151, #2849, #9615, #27126, #16090, #2991, #24694, #7459, #15945, #18650, #11783, #16230, #24979, #7171, #14076, #5002 ),
 .UNSPECIFIED., .F., .F.,
 ( 4, 2, 2, 2, 2, 2, 2, 2, 4 ),
 ( 0.000000000000000000, 0.1250000000000000000, 0.2500000000000000000, 0.3750000000000000000, 0.5000000000000000000, 0.6250000000000000000, 0.7500000000000000000, 0.8750000000000000000, 1.000000000000000000 ),
 .UNSPECIFIED. ) ;
#22808=ORIENTED_EDGE ( 'NONE', *, *, #124, .T. ) ;
#22813=EDGE_LOOP ( 'NONE', ( #23645, #15296, #20880, #2170 ) ) ;
#22818=ADVANCED_FACE ( 'NONE', ( #14516 ), #7964, .F. ) ;
#22820=CARTESIAN_POINT ( 'NONE',  ( -52.45095902829482526, 133.2634102098851372, -14.19419100766092257 ) ) ;
#22822=ADVANCED_FACE ( 'NONE', ( #21251 ), #3437, .T. ) ;
#22823=CARTESIAN_POINT ( 'NONE',  ( -207.5699030661693030, 75.55056756148773900, 43.24289214104831558 ) ) ;
#22825=CARTESIAN_POINT ( 'NONE',  ( -52.44999544250409684, 133.2632066869771563, -14.19424921271702011 ) ) ;
#22828=CARTESIAN_POINT ( 'NONE',  ( -227.0596193454513525, 90.08420170043139308, -13.60108752251566244 ) ) ;
#22831=CARTESIAN_POINT ( 'NONE',  ( -34.12965183067004205, -18.01420295945611727, 100.0000000000000000 ) ) ;
#22833=CARTESIAN_POINT ( 'NONE',  ( 96.76194576697405125, 83.89264379418708018, -100.0000000000000284 ) ) ;
#22834=DIRECTION ( 'NONE',  ( -1.000000000000000000, 0.000000000000000000, 0.000000000000000000 ) ) ;
#22835=EDGE_LOOP ( 'NONE', ( #24960, #12154, #13346 ) ) ;
#22836=ORIENTED_EDGE ( 'NONE', *, *, #946, .F. ) ;
#22838=CARTESIAN_POINT ( 'NONE',  ( -236.8667578982872044, 138.8517089611673043, 5.000000000000002665 ) ) ;
#22840=ORIENTED_EDGE ( 'NONE', *, *, #3191, .T. ) ;
#22842=ORIENTED_EDGE ( 'NONE', *, *, #20583, .F. ) ;
#22846=AXIS2_PLACEMENT_3D ( 'NONE', #19672, #24134, #13221 ) ;
#22852=LINE ( 'NONE', #9788, #19488 ) ;
#22853=DIRECTION ( 'NONE',  ( -1.000000000000000000, -1.233581138472397295E-15, 0.000000000000000000 ) ) ;
#22854=CARTESIAN_POINT ( 'NONE',  ( -219.7112380651048227, 60.27397245185819230, -23.81555219816717894 ) ) ;
#22855=ADVANCED_FACE ( 'NONE', ( #16945 ), #25699, .T. ) ;
#22857=DIRECTION ( 'NONE',  ( 8.673617379884037937E-17, -1.000000000000000000, 0.000000000000000000 ) ) ;
#22859=PLANE ( 'NONE',  #9842 ) ;
#22861=LINE ( 'NONE', #24596, #5479 ) ;
#22863=CARTESIAN_POINT ( 'NONE',  ( -229.4479296852373409, 74.49644851802749201, 16.38316105113803545 ) ) ;
#22864=AXIS2_PLACEMENT_3D ( 'NONE', #6946, #26472, #23771 ) ;
#22870=CARTESIAN_POINT ( 'NONE',  ( 104.1118574116920428, 122.0584436054522257, 100.0000000000000142 ) ) ;
#22877=LINE ( 'NONE', #13996, #3151 ) ;
#22879=CARTESIAN_POINT ( 'NONE',  ( 9.999999999999738876, -50.00000000000004263, 80.00000000000001421 ) ) ;
#22880=ORIENTED_EDGE ( 'NONE', *, *, #18746, .F. ) ;
#22881=CARTESIAN_POINT ( 'NONE',  ( 134.9999999999998579, 330.0000000000000000, -84.99999999999995737 ) ) ;
#22884=CARTESIAN_POINT ( 'NONE',  ( -160.0000000000000568, 139.9999999999999716, 15.00000000000000000 ) ) ;
#22889=EDGE_CURVE ( 'NONE', #19795, #26495, #10200, .T. ) ;
#22892=ORIENTED_EDGE ( 'NONE', *, *, #2904, .T. ) ;
#22899=ORIENTED_EDGE ( 'NONE', *, *, #5299, .T. ) ;
#22901=CYLINDRICAL_SURFACE ( 'NONE', #7943, 10.00000000000000888 ) ;
#22903=DIRECTION ( 'NONE',  ( 0.000000000000000000, 0.000000000000000000, -1.000000000000000000 ) ) ;
#22910=CARTESIAN_POINT ( 'NONE',  ( -82.67666394482243675, 134.7683680720327573, 15.45968317728961594 ) ) ;
#22911=FACE_OUTER_BOUND ( 'NONE', #11908, .T. ) ;
#22922=CARTESIAN_POINT ( 'NONE',  ( 109.9999999999999005, 260.0000000000000000, 45.00000000000000000 ) ) ;
#22925=CARTESIAN_POINT ( 'NONE',  ( -216.4421519707229606, 141.6000904446840991, 15.00000000000000000 ) ) ;
#22926=CARTESIAN_POINT ( 'NONE',  ( 108.2273028572353297, 129.5338070842080924, -88.59375000024363089 ) ) ;
#22931=ADVANCED_FACE ( 'NONE', ( #277 ), #2916, .F. ) ;
#22932=LINE ( 'NONE', #3379, #9240 ) ;
#22937=CARTESIAN_POINT ( 'NONE',  ( 95.84668550246941265, 240.8689031315771558, -9.670617930119313144 ) ) ;
#22940=EDGE_LOOP ( 'NONE', ( #17491, #21072, #22892, #14565 ) ) ;
#22949=AXIS2_PLACEMENT_3D ( 'NONE', #14242, #16808, #9787 ) ;
#22952=ORIENTED_EDGE ( 'NONE', *, *, #2082, .F. ) ;
#22953=CARTESIAN_POINT ( 'NONE',  ( -180.0000000000000284, -70.00000000000004263, 25.00000000000000000 ) ) ;
#22954=LINE ( 'NONE', #7592, #5011 ) ;
#22955=LINE ( 'NONE', #21075, #19380 ) ;
#22956=CARTESIAN_POINT ( 'NONE',  ( -62.53415162963487717, 134.9206139158971780, -15.37869918857521334 ) ) ;
#22960=CARTESIAN_POINT ( 'NONE',  ( -158.6374707261681465, 121.2406993230886201, -20.46622289123956762 ) ) ;
#22964=CARTESIAN_POINT ( 'NONE',  ( -209.0082310152468779, 89.44643712831107507, -24.31564584614111268 ) ) ;
#22966=B_SPLINE_CURVE_WITH_KNOTS ( 'NONE', 3,
 ( #6944, #15445, #2340, #24058, #11121, #4362, #203, #13152, #21892, #15729, #8964, #17723, #26469, #24328, #4638, #24478, #4785, #13573, #1919, #18163, #11985, #27325 ),
 .UNSPECIFIED., .F., .F.,
 ( 4, 2, 2, 2, 2, 2, 2, 2, 2, 2, 4 ),
 ( 0.000000000000000000, 0.004058198178794836415, 0.006087297268192255056, 0.008116396357589672830, 0.01623279271517933872, 0.02029099089397414998, 0.02434918907276896471, 0.02840738725156378292, 0.03043648634096116773, 0.03145103588565986708, 0.03246558543035856642 ),
 .UNSPECIFIED. ) ;
#22967=DIRECTION ( 'NONE',  ( -1.000000000000000000, 0.000000000000000000, 0.000000000000000000 ) ) ;
#22968=CARTESIAN_POINT ( 'NONE',  ( -63.57415822541634043, 29.64876300893806516, 95.00000000000000000 ) ) ;
#22970=AXIS2_PLACEMENT_3D ( 'NONE', #21010, #1335, #8228 ) ;
#22971=CARTESIAN_POINT ( 'NONE',  ( -41.48633590429507478, -19.07744248478647009, 99.88564445205030040 ) ) ;
#22972=CARTESIAN_POINT ( 'NONE',  ( -196.7519430251776384, 98.10118020365993630, 32.13010062293410130 ) ) ;
#22974=ORIENTED_EDGE ( 'NONE', *, *, #3278, .F. ) ;
#22975=ORIENTED_EDGE ( 'NONE', *, *, #17104, .T. ) ;
#22979=EDGE_CURVE ( 'NONE', #13271, #5384, #13491, .T. ) ;
#22990=CARTESIAN_POINT ( 'NONE',  ( 98.66165036324171922, 233.9456810963309579, -21.50628274051351951 ) ) ;
#22992=LINE ( 'NONE', #20550, #15381 ) ;
#22993=LINE ( 'NONE', #27990, #6369 ) ;
#22994=CARTESIAN_POINT ( 'NONE',  ( -207.8780609232275651, 75.32569699198245416, -40.84837702943764981 ) ) ;
#23001=CARTESIAN_POINT ( 'NONE',  ( -200.0065789263009037, 95.74113499274756123, 30.18550423898969015 ) ) ;
#23002=CIRCLE ( 'NONE', #12477, 3.532530335305414493 ) ;
#23005=EDGE_LOOP ( 'NONE', ( #25038, #19557, #5367, #15007 ) ) ;
#23007=CARTESIAN_POINT ( 'NONE',  ( 93.07270601802888166, 112.9533406971467429, 74.06249999970600584 ) ) ;
#23013=ADVANCED_FACE ( 'NONE', ( #4428 ), #7548, .T. ) ;
#23015=DIRECTION ( 'NONE',  ( 1.000000000000000000, 0.000000000000000000, 0.000000000000000000 ) ) ;
#23017=ORIENTED_EDGE ( 'NONE', *, *, #15411, .T. ) ;
#23027=CARTESIAN_POINT ( 'NONE',  ( -175.0000000000000000, -120.0000000000001705, 70.00000000000001421 ) ) ;
#23030=CARTESIAN_POINT ( 'NONE',  ( -185.8971396743188791, 105.9914516682979126, -32.39061618393369457 ) ) ;
#23033=PLANE ( 'NONE',  #20215 ) ;
#23034=CYLINDRICAL_SURFACE ( 'NONE', #11576, 5.000000000000004441 ) ;
#23035=CARTESIAN_POINT ( 'NONE',  ( 79.99999999999990052, 230.0000000000000284, -15.00000000000000000 ) ) ;
#23038=ORIENTED_EDGE ( 'NONE', *, *, #26233, .F. ) ;
#23041=DIRECTION ( 'NONE',  ( 0.000000000000000000, 0.000000000000000000, 1.000000000000000000 ) ) ;
#23042=CARTESIAN_POINT ( 'NONE',  ( 119.9999999999999147, 140.0000000000000000, -100.0000000000000142 ) ) ;
#23043=DIRECTION ( 'NONE',  ( 1.000000000000000000, 0.000000000000000000, 0.000000000000000000 ) ) ;
#23046=DIRECTION ( 'NONE',  ( 1.000000000000000000, 0.000000000000000000, 0.000000000000000000 ) ) ;
#23051=CARTESIAN_POINT ( 'NONE',  ( -136.9485176461679998, 127.8960360072517801, 17.54782681003734268 ) ) ;
#23053=ORIENTED_EDGE ( 'NONE', *, *, #5342, .F. ) ;
#23060=ORIENTED_EDGE ( 'NONE', *, *, #8874, .F. ) ;
#23065=CARTESIAN_POINT ( 'NONE',  ( 109.9999999999999574, -120.0000000000000426, 100.0000000000000142 ) ) ;
#23068=AXIS2_PLACEMENT_3D ( 'NONE', #10121, #21021, #19294 ) ;
#23069=CARTESIAN_POINT ( 'NONE',  ( 84.91648909967481984, 110.3843228249420321, -70.37109374985145394 ) ) ;
#23071=CARTESIAN_POINT ( 'NONE',  ( -115.3221550338875687, 71.54464929955099706, 83.00000000000001421 ) ) ;
#23072=ADVANCED_FACE ( 'NONE', ( #24689 ), #7985, .F. ) ;
#23073=DIRECTION ( 'NONE',  ( 0.4163300014277677707, -0.9092135777204137792, 0.000000000000000000 ) ) ;
#23078=CARTESIAN_POINT ( 'NONE',  ( -23.64180107668250486, 129.3206000201379879, 15.61667362249785818 ) ) ;
#23080=CARTESIAN_POINT ( 'NONE',  ( 79.99999999999990052, 230.0000000000000284, -5.000000000000002665 ) ) ;
#23084=ORIENTED_EDGE ( 'NONE', *, *, #23656, .T. ) ;
#23086=AXIS2_PLACEMENT_3D ( 'NONE', #25061, #23041, #20737 ) ;
#23088=VERTEX_POINT ( 'NONE', #14071 ) ;
#23097=CARTESIAN_POINT ( 'NONE',  ( 113.1867617905505625, 214.4608731583509496, 97.32202223992300105 ) ) ;
#23108=VECTOR ( 'NONE', #1376, 1000.000000000000000 ) ;
#23111=DIRECTION ( 'NONE',  ( -1.000000000000000000, 0.000000000000000000, 0.000000000000000000 ) ) ;
#23114=CARTESIAN_POINT ( 'NONE',  ( -35.14662420382099128, -18.36872720267034254, 100.0000000000000142 ) ) ;
#23115=CARTESIAN_POINT ( 'NONE',  ( -189.6856883378720795, 103.4044969352196546, 32.84415653362697896 ) ) ;
#23124=VERTEX_POINT ( 'NONE', #3121 ) ;
#23129=EDGE_CURVE ( 'NONE', #6895, #5063, #25854, .T. ) ;
#23130=DIRECTION ( 'NONE',  ( -1.530283246943720875E-16, 1.000000000000000000, -0.000000000000000000 ) ) ;
#23131=DIRECTION ( 'NONE',  ( 0.000000000000000000, 0.000000000000000000, -1.000000000000000000 ) ) ;
#23132=CARTESIAN_POINT ( 'NONE',  ( -11.25164642577565033, 130.1410301030969663, -16.65746621873669397 ) ) ;
#23133=DIRECTION ( 'NONE',  ( 0.000000000000000000, 0.000000000000000000, -1.000000000000000000 ) ) ;
#23136=CARTESIAN_POINT ( 'NONE',  ( -221.2300551840314711, 71.39986350410367777, -20.78524708593021941 ) ) ;
#23139=ADVANCED_FACE ( 'NONE', ( #7167 ), #14409, .T. ) ;
#23142=DIRECTION ( 'NONE',  ( 0.000000000000000000, -0.000000000000000000, 1.000000000000000000 ) ) ;
#23144=DIRECTION ( 'NONE',  ( -1.000000000000000000, 0.000000000000000000, -0.000000000000000000 ) ) ;
#23146=ORIENTED_EDGE ( 'NONE', *, *, #25091, .T. ) ;
#23147=CARTESIAN_POINT ( 'NONE',  ( -200.0664673763980943, 95.37061492405908325, 31.11141022391927535 ) ) ;
#23152=CARTESIAN_POINT ( 'NONE',  ( 119.9999999999999147, 140.0000000000000000, 100.0000000000000142 ) ) ;
#23157=CARTESIAN_POINT ( 'NONE',  ( 84.91648909967481984, 110.3843228249420321, -70.37109374985145394 ) ) ;
#23158=CARTESIAN_POINT ( 'NONE',  ( 109.9999999999999005, 260.0000000000000000, 45.00000000000000000 ) ) ;
#23164=DIRECTION ( 'NONE',  ( -1.000000000000000000, -0.000000000000000000, -0.000000000000000000 ) ) ;
#23167=CARTESIAN_POINT ( 'NONE',  ( -17.24491960465746132, 75.97823757117562593, 95.00000000000000000 ) ) ;
#23171=DIRECTION ( 'NONE',  ( -0.000000000000000000, -1.000000000000000000, -0.000000000000000000 ) ) ;
#23175=EDGE_CURVE ( 'NONE', #26642, #10685, #1146, .T. ) ;
#23177=FACE_OUTER_BOUND ( 'NONE', #11724, .T. ) ;
#23179=CARTESIAN_POINT ( 'NONE',  ( -175.0000000000000000, -120.0000000000001847, -76.02499999999999147 ) ) ;
#23180=VERTEX_POINT ( 'NONE', #12723 ) ;
#23181=VECTOR ( 'NONE', #17908, 1000.000000000000000 ) ;
#23182=CARTESIAN_POINT ( 'NONE',  ( -241.9743096803475453, -91.18033988749901653, 0.000000000000000000 ) ) ;
#23186=CARTESIAN_POINT ( 'NONE',  ( -28.05246235954390244, 188.0718642840173516, -13.00000000000000000 ) ) ;
#23190=VECTOR ( 'NONE', #887, 1000.000000000000000 ) ;
#23195=VERTEX_POINT ( 'NONE', #14729 ) ;
#23197=VERTEX_POINT ( 'NONE', #5954 ) ;
#23202=CARTESIAN_POINT ( 'NONE',  ( 109.8202728674729656, 257.1791079647171614, 41.57776855479137623 ) ) ;
#23207=VECTOR ( 'NONE', #18829, 1000.000000000000000 ) ;
#23209=CYLINDRICAL_SURFACE ( 'NONE', #13124, 16.46313063346208239 ) ;
#23215=EDGE_LOOP ( 'NONE', ( #6524, #21487, #27553, #4590 ) ) ;
#23217=EDGE_CURVE ( 'NONE', #28119, #11333, #10739, .T. ) ;
#23219=CARTESIAN_POINT ( 'NONE',  ( 89.99999999999988631, 240.0000000000000284, -6.270166537926030514 ) ) ;
#23220=CARTESIAN_POINT ( 'NONE',  ( 11.04815889348632041, 90.00000000000004263, 98.28427124746193044 ) ) ;
#23224=ORIENTED_EDGE ( 'NONE', *, *, #16118, .T. ) ;
#23233=CARTESIAN_POINT ( 'NONE',  ( -67.48155814317149748, 135.5182078837663369, 13.65863916513348997 ) ) ;
#23235=APPLICATION_CONTEXT ( 'automotive_design' ) ;
#23238=CARTESIAN_POINT ( 'NONE',  ( 113.9305603607157025, 227.9104510466760303, 97.95022080735130032 ) ) ;
#23239=DIRECTION ( 'NONE',  ( 0.000000000000000000, 1.000000000000000000, 0.000000000000000000 ) ) ;
#23240=CARTESIAN_POINT ( 'NONE',  ( 79.99999999999994316, -100.0000000000000284, 100.0000000000000142 ) ) ;
#23243=DIRECTION ( 'NONE',  ( -0.000000000000000000, 0.000000000000000000, 1.000000000000000000 ) ) ;
#23251=ORIENTED_EDGE ( 'NONE', *, *, #24565, .F. ) ;
#23252=ADVANCED_FACE ( 'NONE', ( #8681 ), #6237, .T. ) ;
#23254=CARTESIAN_POINT ( 'NONE',  ( -46.68942599940377391, -18.01420295945611727, 100.0000000000000000 ) ) ;
#23256=EDGE_LOOP ( 'NONE', ( #18422, #23084, #4335, #8702 ) ) ;
#23260=ORIENTED_EDGE ( 'NONE', *, *, #14087, .T. ) ;
#23261=VECTOR ( 'NONE', #3044, 1000.000000000000000 ) ;
#23264=AXIS2_PLACEMENT_3D ( 'NONE', #5844, #7859, #5985 ) ;
#23269=CARTESIAN_POINT ( 'NONE',  ( -233.2943309833553371, 92.06151970357247194, 13.00000000000000000 ) ) ;
#23271=LINE ( 'NONE', #4144, #12384 ) ;
#23273=DIRECTION ( 'NONE',  ( 0.000000000000000000, 1.000000000000000000, -0.000000000000000000 ) ) ;
#23277=CIRCLE ( 'NONE', #16417, 6.000000000000005329 ) ;
#23278=CARTESIAN_POINT ( 'NONE',  ( -194.2411556039511709, 63.21395545898181467, -45.39084185613187827 ) ) ;
#23279=LINE ( 'NONE', #27428, #15089 ) ;
#23280=CARTESIAN_POINT ( 'NONE',  ( 79.99999999999991473, 140.0000000000000000, -45.00000000000000000 ) ) ;
#23281=CARTESIAN_POINT ( 'NONE',  ( -270.1025481742786951, -91.18033988749901653, 11.42311362948588105 ) ) ;
#23283=VERTEX_POINT ( 'NONE', #19594 ) ;
#23285=CARTESIAN_POINT ( 'NONE',  ( -229.2498027451138967, 132.0565166830976978, -15.00000000000000000 ) ) ;
#23288=EDGE_LOOP ( 'NONE', ( #7189, #267, #9824, #17802 ) ) ;
#23291=CARTESIAN_POINT ( 'NONE',  ( 95.20156243614241021, 83.09913198708241566, 100.0000000000000142 ) ) ;
#23292=LINE ( 'NONE', #12394, #6705 ) ;
#23293=VERTEX_POINT ( 'NONE', #26193 ) ;
#23294=EDGE_CURVE ( 'NONE', #14508, #8985, #12054, .T. ) ;
#23302=CARTESIAN_POINT ( 'NONE',  ( 119.7545560453059892, 132.4900181921427702, 100.0000000000000142 ) ) ;
#23308=DIRECTION ( 'NONE',  ( 0.000000000000000000, 0.000000000000000000, -1.000000000000000000 ) ) ;
#23313=CARTESIAN_POINT ( 'NONE',  ( 79.99999999999992895, 110.0000000000000000, 70.00000000000001421 ) ) ;
#23321=CARTESIAN_POINT ( 'NONE',  ( -200.0057241004398634, 95.74183647495578953, 30.18583206540278141 ) ) ;
#23322=DIRECTION ( 'NONE',  ( 0.000000000000000000, -0.000000000000000000, -1.000000000000000000 ) ) ;
#23327=EDGE_CURVE ( 'NONE', #6913, #18244, #11209, .T. ) ;
#23335=ORIENTED_EDGE ( 'NONE', *, *, #17034, .T. ) ;
#23340=B_SPLINE_CURVE_WITH_KNOTS ( 'NONE', 3,
 ( #17567, #26325, #15292, #24045, #13141, #26044, #6364, #17148, #12997, #192, #24316, #21881, #2187, #1909 ),
 .UNSPECIFIED., .F., .F.,
 ( 4, 2, 2, 2, 2, 2, 4 ),
 ( 2.775557561562891351E-17, 0.001449360111607882239, 0.002174040167411816094, 0.002898720223215749733, 0.003623400279019683371, 0.004348080334823617443, 0.005797440446431482118 ),
 .UNSPECIFIED. ) ;
#23347=CARTESIAN_POINT ( 'NONE',  ( -225.1304350307114532, 62.42764488596311878, -8.801787756210094571 ) ) ;
#23360=CARTESIAN_POINT ( 'NONE',  ( -231.0630381273050489, 75.70161533889120165, 15.87871908887787953 ) ) ;
#23361=ORIENTED_EDGE ( 'NONE', *, *, #17196, .F. ) ;
#23365=CARTESIAN_POINT ( 'NONE',  ( -85.27503253815632434, 136.4561186087251770, 15.16277632316441881 ) ) ;
#23366=CIRCLE ( 'NONE', #11452, 30.00000000000000000 ) ;
#23369=ORIENTED_EDGE ( 'NONE', *, *, #12611, .F. ) ;
#23371=CARTESIAN_POINT ( 'NONE',  ( 113.6021183481338284, 226.9733193880700242, 97.68838206577115102 ) ) ;
#23372=DIRECTION ( 'NONE',  ( 0.000000000000000000, 0.000000000000000000, 1.000000000000000000 ) ) ;
#23375=ADVANCED_FACE ( 'NONE', ( #22031 ), #27251, .F. ) ;
#23376=CARTESIAN_POINT ( 'NONE',  ( -134.5993320547982535, 128.5490369126959251, -17.26385867077430447 ) ) ;
#23380=LINE ( 'NONE', #21081, #14509 ) ;
#23382=CARTESIAN_POINT ( 'NONE',  ( -218.6660474811943971, 86.19516118637005775, 19.43150922036087280 ) ) ;
#23383=CARTESIAN_POINT ( 'NONE',  ( 65.00000000000000000, -120.0250000000000909, -69.99999999999998579 ) ) ;
#23389=CARTESIAN_POINT ( 'NONE',  ( -110.3221550338875687, 20.24192588826928585, 80.00000000000001421 ) ) ;
#23395=CARTESIAN_POINT ( 'NONE',  ( 101.0213870967668299, 236.0005211361351485, -23.58009545578860511 ) ) ;
#23398=ORIENTED_EDGE ( 'NONE', *, *, #2842, .F. ) ;
#23400=ORIENTED_EDGE ( 'NONE', *, *, #24461, .T. ) ;
#23404=EDGE_CURVE ( 'NONE', #15146, #23195, #2626, .T. ) ;
#23409=VECTOR ( 'NONE', #12507, 1000.000000000000000 ) ;
#23411=DIRECTION ( 'NONE',  ( 0.000000000000000000, 1.000000000000000000, 0.000000000000000000 ) ) ;
#23413=CARTESIAN_POINT ( 'NONE',  ( -207.5241688850417745, 75.58432268001081411, -43.94049219536437789 ) ) ;
#23417=LINE ( 'NONE', #19678, #12911 ) ;
#23420=CARTESIAN_POINT ( 'NONE',  ( -203.3278902001933943, 92.92226908766612326, 29.32321494459338851 ) ) ;
#23423=DIRECTION ( 'NONE',  ( 0.000000000000000000, 0.000000000000000000, 1.000000000000000000 ) ) ;
#23428=ORIENTED_EDGE ( 'NONE', *, *, #17196, .T. ) ;
#23435=DIRECTION ( 'NONE',  ( -0.000000000000000000, -0.000000000000000000, 1.000000000000000000 ) ) ;
#23439=CARTESIAN_POINT ( 'NONE',  ( -175.0000000000000000, -150.0000000000000853, -69.99999999999998579 ) ) ;
#23441=DIRECTION ( 'NONE',  ( 0.000000000000000000, 0.000000000000000000, -1.000000000000000000 ) ) ;
#23445=DIRECTION ( 'NONE',  ( -0.000000000000000000, -0.000000000000000000, -1.000000000000000000 ) ) ;
#23456=EDGE_LOOP ( 'NONE', ( #441, #1136, #18027, #11994 ) ) ;
#23462=CARTESIAN_POINT ( 'NONE',  ( -227.0732549327441632, 90.14410762487624140, 13.63207569781857131 ) ) ;
#23463=ORIENTED_EDGE ( 'NONE', *, *, #7015, .F. ) ;
#23467=AXIS2_PLACEMENT_3D ( 'NONE', #16783, #25961, #12764 ) ;
#23470=ORIENTED_EDGE ( 'NONE', *, *, #16314, .F. ) ;
#23472=ORIENTED_EDGE ( 'NONE', *, *, #5750, .T. ) ;
#23475=AXIS2_PLACEMENT_3D ( 'NONE', #823, #7847, #16620 ) ;
#23481=DIRECTION ( 'NONE',  ( 0.000000000000000000, 0.000000000000000000, -1.000000000000000000 ) ) ;
#23483=FACE_OUTER_BOUND ( 'NONE', #1948, .T. ) ;
#23486=CARTESIAN_POINT ( 'NONE',  ( -242.5499235585615452, 73.68467268309757401, -14.74213902348974159 ) ) ;
#23493=LINE ( 'NONE', #22329, #10049 ) ;
#23498=EDGE_CURVE ( 'NONE', #12493, #2404, #25319, .T. ) ;
#23500=CARTESIAN_POINT ( 'NONE',  ( -156.2917263574996127, 178.8555734514394828, -15.00000000000000000 ) ) ;
#23501=DIRECTION ( 'NONE',  ( 1.000000000000000000, 0.000000000000000000, 0.000000000000000000 ) ) ;
#23504=CARTESIAN_POINT ( 'NONE',  ( -234.3977820475819840, 78.94297905343258037, 15.16298856074166679 ) ) ;
#23505=ORIENTED_EDGE ( 'NONE', *, *, #12508, .T. ) ;
#23516=CIRCLE ( 'NONE', #15740, 18.46313063346208239 ) ;
#23517=CARTESIAN_POINT ( 'NONE',  ( -122.5485268256659594, 131.3750725269259476, -16.25384529279319779 ) ) ;
#23521=EDGE_CURVE ( 'NONE', #17245, #10183, #25875, .T. ) ;
#23523=CARTESIAN_POINT ( 'NONE',  ( -229.2280533001591607, 91.38976949163449603, -15.26004308210696792 ) ) ;
#23526=CARTESIAN_POINT ( 'NONE',  ( -227.9935532272682508, 88.33663008737792666, 15.67459936273962384 ) ) ;
#23529=DIRECTION ( 'NONE',  ( 1.000000000000000000, 0.000000000000000000, 0.000000000000000000 ) ) ;
#23536=CARTESIAN_POINT ( 'NONE',  ( 65.00000000000000000, -120.0250000000000625, 70.00000000000001421 ) ) ;
#23538=ORIENTED_EDGE ( 'NONE', *, *, #11773, .F. ) ;
#23542=CARTESIAN_POINT ( 'NONE',  ( 103.8044331943715122, 239.2408796537650346, -26.67200500018732612 ) ) ;
#23549=CIRCLE ( 'NONE', #11168, 6.204828372381208546 ) ;
#23550=DIRECTION ( 'NONE',  ( 0.000000000000000000, 0.000000000000000000, -1.000000000000000000 ) ) ;
#23551=VECTOR ( 'NONE', #20320, 1000.000000000000000 ) ;
#23553=CIRCLE ( 'NONE', #11174, 22.49999999999999289 ) ;
#23554=CARTESIAN_POINT ( 'NONE',  ( -196.7918453702777128, 20.24192588826928585, 80.00000000000001421 ) ) ;
#23556=CARTESIAN_POINT ( 'NONE',  ( 7.471928113118646131, 138.6332119385803594, -15.00000000000000178 ) ) ;
#23564=CARTESIAN_POINT ( 'NONE',  ( 0.000000000000000000, 0.000000000000000000, 100.0000000000000000 ) ) ;
#23566=AXIS2_PLACEMENT_3D ( 'NONE', #11808, #20548, #9364 ) ;
#23567=CARTESIAN_POINT ( 'NONE',  ( 117.2377723979416970, 233.8231604766229168, -99.61817846762012607 ) ) ;
#23570=EDGE_CURVE ( 'NONE', #4881, #6807, #22783, .T. ) ;
#23583=CARTESIAN_POINT ( 'NONE',  ( 103.3065434576170531, 238.5579404054215047, 26.03666308166562970 ) ) ;
#23584=CARTESIAN_POINT ( 'NONE',  ( -192.2801638615682691, 101.7426455718185281, -32.00518413859087730 ) ) ;
#23587=ORIENTED_EDGE ( 'NONE', *, *, #13381, .F. ) ;
#23588=AXIS2_PLACEMENT_3D ( 'NONE', #26334, #18157, #15441 ) ;
#23591=VECTOR ( 'NONE', #2457, 1000.000000000000000 ) ;
#23594=CARTESIAN_POINT ( 'NONE',  ( -194.9328835026024080, 99.53491429316976280, -32.53590786292448200 ) ) ;
#23603=CARTESIAN_POINT ( 'NONE',  ( -203.1779787704217313, 93.05164332230201296, 28.77272332722132120 ) ) ;
#23604=CARTESIAN_POINT ( 'NONE',  ( -214.3828916364065833, 175.2783111443768576, -13.00000000000000000 ) ) ;
#23607=FACE_OUTER_BOUND ( 'NONE', #18216, .T. ) ;
#23610=DIRECTION ( 'NONE',  ( -0.000000000000000000, -0.000000000000000000, 1.000000000000000000 ) ) ;
#23611=CARTESIAN_POINT ( 'NONE',  ( -199.2320231536486403, 96.36337958803088100, -30.96155907179247890 ) ) ;
#23617=VERTEX_POINT ( 'NONE', #17260 ) ;
#23618=ORIENTED_EDGE ( 'NONE', *, *, #18536, .F. ) ;
#23621=EDGE_CURVE ( 'NONE', #24673, #14597, #2956, .T. ) ;
#23623=AXIS2_PLACEMENT_3D ( 'NONE', #16877, #5953, #12722 ) ;
#23624=EDGE_CURVE ( 'NONE', #3986, #17824, #19935, .T. ) ;
#23625=DIRECTION ( 'NONE',  ( 0.000000000000000000, 0.000000000000000000, -1.000000000000000000 ) ) ;
#23626=CARTESIAN_POINT ( 'NONE',  ( -180.0000000000000284, -50.00000000000004263, 80.00000000000001421 ) ) ;
#23628=CIRCLE ( 'NONE', #15837, 41.00000000000000000 ) ;
#23629=CARTESIAN_POINT ( 'NONE',  ( -279.3160071107327553, -512.7211954420570237, 0.000000000000000000 ) ) ;
#23631=CARTESIAN_POINT ( 'NONE',  ( -238.3574390336367514, 69.78222348740686698, -5.410870504202835995 ) ) ;
#23634=TOROIDAL_SURFACE ( 'NONE', #3442, 60.90601976618767566, 2.000000000000000000 ) ;
#23638=EDGE_LOOP ( 'NONE', ( #8528, #16868, #18794, #23745 ) ) ;
#23640=DIRECTION ( 'NONE',  ( 0.000000000000000000, 0.000000000000000000, -1.000000000000000000 ) ) ;
#23642=CARTESIAN_POINT ( 'NONE',  ( -43.02437977270766112, 129.0347155322979233, 14.93735646117640847 ) ) ;
#23644=CARTESIAN_POINT ( 'NONE',  ( 79.99999999999995737, 59.99999999999998579, 45.00000000000000000 ) ) ;
#23645=ORIENTED_EDGE ( 'NONE', *, *, #4876, .T. ) ;
#23648=CARTESIAN_POINT ( 'NONE',  ( 179.9999999999999147, -150.0000000000000284, 100.0000000000000142 ) ) ;
#23649=ORIENTED_EDGE ( 'NONE', *, *, #6149, .T. ) ;
#23650=CIRCLE ( 'NONE', #17675, 30.00000000000000000 ) ;
#23651=VECTOR ( 'NONE', #25633, 1000.000000000000000 ) ;
#23652=TOROIDAL_SURFACE ( 'NONE', #4361, 80.00000000000000000, 30.00000000000000000 ) ;
#23654=CARTESIAN_POINT ( 'NONE',  ( -67.69391036949915019, 133.9331560312302258, 15.61747421727902463 ) ) ;
#23655=VERTEX_POINT ( 'NONE', #12689 ) ;
#23656=EDGE_CURVE ( 'NONE', #26678, #9167, #8926, .T. ) ;
#23657=CIRCLE ( 'NONE', #7131, 4.999999999999997335 ) ;
#23658=ORIENTED_EDGE ( 'NONE', *, *, #27823, .F. ) ;
#23663=ADVANCED_FACE ( 'NONE', ( #4180 ), #12149, .F. ) ;
#23664=ADVANCED_FACE ( 'NONE', ( #6202 ), #16981, .T. ) ;
#23665=CARTESIAN_POINT ( 'NONE',  ( -113.0279832246674232, 134.5396197302765700, -13.86330562916807274 ) ) ;
#23668=CARTESIAN_POINT ( 'NONE',  ( -214.9809428154103728, 87.87766106360727747, -21.23882047124828176 ) ) ;
#23671=CARTESIAN_POINT ( 'NONE',  ( -203.2481855153402250, 92.57460631283319685, 29.78692811926998729 ) ) ;
#23676=ORIENTED_EDGE ( 'NONE', *, *, #27528, .F. ) ;
#23679=LINE ( 'NONE', #21516, #1440 ) ;
#23681=ORIENTED_EDGE ( 'NONE', *, *, #23621, .T. ) ;
#23683=CARTESIAN_POINT ( 'NONE',  ( 96.29556199549620032, 241.0127520899152387, -10.03785181564776963 ) ) ;
#23684=VERTEX_POINT ( 'NONE', #2030 ) ;
#23686=ORIENTED_EDGE ( 'NONE', *, *, #15186, .F. ) ;
#23690=VERTEX_POINT ( 'NONE', #16843 ) ;
#23691=ORIENTED_EDGE ( 'NONE', *, *, #12830, .F. ) ;
#23692=CIRCLE ( 'NONE', #27811, 22.49999999999999289 ) ;
#23694=ADVANCED_FACE ( 'NONE', ( #14839 ), #1467, .T. ) ;
#23696=CARTESIAN_POINT ( 'NONE',  ( 65.00000000000000000, -120.0000000000000711, 70.00000000000001421 ) ) ;
#23700=DIRECTION ( 'NONE',  ( -0.000000000000000000, 1.000000000000000000, 0.000000000000000000 ) ) ;
#23702=CARTESIAN_POINT ( 'NONE',  ( -227.7405116417571946, 73.49447507798586798, -17.05698111974955111 ) ) ;
#23703=CARTESIAN_POINT ( 'NONE',  ( -42.53273978471831640, 130.9733465240572627, 14.93735646117640670 ) ) ;
#23704=DIRECTION ( 'NONE',  ( -0.000000000000000000, 0.000000000000000000, -1.000000000000000000 ) ) ;
#23707=EDGE_LOOP ( 'NONE', ( #5698, #4169, #19574, #20328 ) ) ;
#23709=CARTESIAN_POINT ( 'NONE',  ( -186.0983758910577990, 106.1011689576974248, 31.60744335178514319 ) ) ;
#23716=CARTESIAN_POINT ( 'NONE',  ( 113.4920585194047078, 104.4775165427241319, 100.0000000000000142 ) ) ;
#23717=CARTESIAN_POINT ( 'NONE',  ( 110.9201389036588949, 220.0000000000000284, 153.1081322850112940 ) ) ;
#23720=CARTESIAN_POINT ( 'NONE',  ( 101.7779539750033280, 119.2876405404464890, -82.50000000032424907 ) ) ;
#23721=CARTESIAN_POINT ( 'NONE',  ( 99.01626835887864786, 234.2217840360999332, 21.79255213936348312 ) ) ;
#23722=DIRECTION ( 'NONE',  ( 1.000000000000000000, 2.312964634635742957E-16, 0.000000000000000000 ) ) ;
#23723=ORIENTED_EDGE ( 'NONE', *, *, #13572, .T. ) ;
#23724=CARTESIAN_POINT ( 'NONE',  ( -206.8923702502391393, 90.46133927671940000, 26.11705481793761052 ) ) ;
#23727=DIRECTION ( 'NONE',  ( 0.000000000000000000, 0.000000000000000000, -1.000000000000000000 ) ) ;
#23729=EDGE_CURVE ( 'NONE', #1362, #21744, #8928, .T. ) ;
#23730=DIRECTION ( 'NONE',  ( 0.000000000000000000, 0.000000000000000000, -1.000000000000000000 ) ) ;
#23731=DIRECTION ( 'NONE',  ( 1.000000000000000000, 4.533410683886055032E-14, 0.000000000000000000 ) ) ;
#23740=CARTESIAN_POINT ( 'NONE',  ( 179.9999999999999147, 0.000000000000000000, 100.0000000000000142 ) ) ;
#23741=AXIS2_PLACEMENT_3D ( 'NONE', #5918, #14416, #23308 ) ;
#23742=CARTESIAN_POINT ( 'NONE',  ( -184.3234090630027140, 107.2774685039649114, 31.16804357237790057 ) ) ;
#23743=CARTESIAN_POINT ( 'NONE',  ( 33.10302365956999182, 203.2034914284457159, -13.00000000000000000 ) ) ;
#23744=CARTESIAN_POINT ( 'NONE',  ( -219.0825447683637606, 87.83772393549990909, 16.88515830131742490 ) ) ;
#23745=ORIENTED_EDGE ( 'NONE', *, *, #19364, .F. ) ;
#23746=SHAPE_REPRESENTATION_RELATIONSHIP ( 'NONE' , 'NONE' ,  #24038, #19102 ) ;
#23747=DIRECTION ( 'NONE',  ( -0.000000000000000000, -0.000000000000000000, -1.000000000000000000 ) ) ;
#23749=TOROIDAL_SURFACE ( 'NONE', #27405, 55.86582179324592090, 2.000000000000000000 ) ;
#23750=EDGE_CURVE ( 'NONE', #2290, #2948, #11380, .T. ) ;
#23752=CARTESIAN_POINT ( 'NONE',  ( -168.1616170882788026, 116.6881954979569258, -24.56124631037856076 ) ) ;
#23761=CIRCLE ( 'NONE', #8161, 166.0121251338587172 ) ;
#23763=CARTESIAN_POINT ( 'NONE',  ( 33.10302365956999182, 219.6666220619077876, -15.00000000000000000 ) ) ;
#23767=DIRECTION ( 'NONE',  ( 1.000000000000000000, 0.000000000000000000, 0.000000000000000000 ) ) ;
#23768=CARTESIAN_POINT ( 'NONE',  ( -228.3003245610471481, 63.46411924055758647, -17.58993856061233529 ) ) ;
#23771=DIRECTION ( 'NONE',  ( 1.000000000000000000, 0.000000000000000000, 0.000000000000000000 ) ) ;
#23779=DIRECTION ( 'NONE',  ( 1.000000000000000000, 0.000000000000000000, 0.000000000000000000 ) ) ;
#23784=VERTEX_POINT ( 'NONE', #4603 ) ;
#23792=ORIENTED_EDGE ( 'NONE', *, *, #14485, .T. ) ;
#23795=DIRECTION ( 'NONE',  ( 1.000000000000000000, 0.000000000000000000, -0.000000000000000000 ) ) ;
#23799=CARTESIAN_POINT ( 'NONE',  ( -217.7401460507702780, 138.5677444271782122, 12.99353264123212703 ) ) ;
#23800=CARTESIAN_POINT ( 'NONE',  ( -127.2321417042300311, 130.3961964139149075, -16.54948570837689914 ) ) ;
#23802=VECTOR ( 'NONE', #2713, 1000.000000000000000 ) ;
#23803=CARTESIAN_POINT ( 'NONE',  ( -158.3239166661295485, 121.3790681822268738, -21.42498206582862608 ) ) ;
#23807=AXIS2_PLACEMENT_3D ( 'NONE', #25430, #3584, #8334 ) ;
#23808=DIRECTION ( 'NONE',  ( -0.7059982162894324897, 0.7082136108520787898, 0.000000000000000000 ) ) ;
#23809=CARTESIAN_POINT ( 'NONE',  ( -220.6589170087162017, 88.04539541979674766, -18.04441532903050671 ) ) ;
#23818=CARTESIAN_POINT ( 'NONE',  ( 119.9999999999999147, 140.0000000000000000, 100.0000000000000142 ) ) ;
#23823=EDGE_CURVE ( 'NONE', #27477, #15024, #672, .T. ) ;
#23824=AXIS2_PLACEMENT_3D ( 'NONE', #16023, #27202, #9261 ) ;
#23825=CARTESIAN_POINT ( 'NONE',  ( 105.2802062291979581, 246.7841820210335584, -28.66020632211111518 ) ) ;
#23827=CARTESIAN_POINT ( 'NONE',  ( -4.329483062107786218, 134.1423878703578225, -13.93341408620584687 ) ) ;
#23836=CIRCLE ( 'NONE', #18784, 53.86582179324592090 ) ;
#23838=PLANE ( 'NONE',  #16061 ) ;
#23844=LINE ( 'NONE', #12235, #1150 ) ;
#23846=FACE_OUTER_BOUND ( 'NONE', #18464, .T. ) ;
#23849=CARTESIAN_POINT ( 'NONE',  ( -210.0000000000000568, 59.99999999999992895, 18.66498670256683212 ) ) ;
#23851=ADVANCED_FACE ( 'NONE', ( #11676 ), #27155, .T. ) ;
#23852=DIRECTION ( 'NONE',  ( 0.000000000000000000, 0.000000000000000000, 1.000000000000000000 ) ) ;
#23854=DIRECTION ( 'NONE',  ( -0.000000000000000000, 1.000000000000000000, -0.000000000000000000 ) ) ;
#23872=CARTESIAN_POINT ( 'NONE',  ( -225.7040669049297037, 89.49289086750439992, 16.08021328254498883 ) ) ;
#23874=CARTESIAN_POINT ( 'NONE',  ( 65.00000000000000000, -120.0000000000000995, -69.99999999999998579 ) ) ;
#23881=CARTESIAN_POINT ( 'NONE',  ( 115.6411010564578561, 208.5333949360010308, 99.00000000000001421 ) ) ;
#23883=DIRECTION ( 'NONE',  ( -0.000000000000000000, 0.000000000000000000, 1.000000000000000000 ) ) ;
#23885=ORIENTED_EDGE ( 'NONE', *, *, #18926, .T. ) ;
#23886=FACE_BOUND ( 'NONE', #1164, .T. ) ;
#23889=CARTESIAN_POINT ( 'NONE',  ( -175.4043012490592730, 112.7503553874411608, 27.84382049740324305 ) ) ;
#23890=CARTESIAN_POINT ( 'NONE',  ( -235.6837214056122036, 120.7228219557777180, 12.99999999999999822 ) ) ;
#23891=CARTESIAN_POINT ( 'NONE',  ( -223.0800714857218452, 88.58381330274964682, 14.94850374233409696 ) ) ;
#23897=CARTESIAN_POINT ( 'NONE',  ( -164.2202815706227454, 118.6546980540646956, -23.76065989308352755 ) ) ;
#23899=ORIENTED_EDGE ( 'NONE', *, *, #9093, .F. ) ;
#23901=ORIENTED_EDGE ( 'NONE', *, *, #13917, .T. ) ;
#23904=ORIENTED_EDGE ( 'NONE', *, *, #16045, .F. ) ;
#23914=CARTESIAN_POINT ( 'NONE',  ( -235.2766700735766960, 67.45978041261076896, -15.24953891110926918 ) ) ;
#23917=B_SPLINE_CURVE_WITH_KNOTS ( 'NONE', 3,
 ( #23881, #2035, #10809, #28306, #17408, #26167, #17546, #13119 ),
 .UNSPECIFIED., .F., .F.,
 ( 4, 2, 2, 4 ),
 ( 0.03156115556266906458, 0.03330631506936755637, 0.03505147457606604816, 0.03854179358946308726 ),
 .UNSPECIFIED. ) ;
#23919=DIRECTION ( 'NONE',  ( 0.000000000000000000, 0.000000000000000000, -1.000000000000000000 ) ) ;
#23921=ORIENTED_EDGE ( 'NONE', *, *, #8250, .T. ) ;
#23928=ORIENTED_EDGE ( 'NONE', *, *, #6104, .F. ) ;
#23932=CARTESIAN_POINT ( 'NONE',  ( 134.9999999999998579, 220.0000000000000284, -90.00000000000002842 ) ) ;
#23942=CARTESIAN_POINT ( 'NONE',  ( -92.57281119172596107, 134.7193011466158339, -15.46818772961191257 ) ) ;
#23947=B_SPLINE_CURVE_WITH_KNOTS ( 'NONE', 3,
 ( #13342, #17349, #15641, #15215, #26256, #23827, #11038, #19787, #4135, #23969, #10897, #11180, #19652, #22233, #28389, #26388, #115, #2396, #11329, #17924, #6717, #28259, #8737, #12918 ),
 .UNSPECIFIED., .F., .F.,
 ( 4, 2, 2, 2, 2, 2, 2, 2, 2, 2, 2, 4 ),
 ( 0.000000000000000000, 0.006705505486134448294, 0.01341101097226889659, 0.01676376371533612117, 0.02011651645840334748, 0.02682202194453779318, 0.03352752743067224928, 0.03520390380220585202, 0.03688028017373946171, 0.04023303291680666027, 0.04693853840294105045, 0.05364404388907543370 ),
 .UNSPECIFIED. ) ;
#23948=CARTESIAN_POINT ( 'NONE',  ( -189.8086322075389774, 92.49158130768422836, 12.99999999999999822 ) ) ;
#23950=VECTOR ( 'NONE', #16030, 1000.000000000000000 ) ;
#23957=DIRECTION ( 'NONE',  ( -0.000000000000000000, 0.000000000000000000, 1.000000000000000000 ) ) ;
#23959=DIRECTION ( 'NONE',  ( -1.000000000000000000, -4.625929269271485914E-16, 0.000000000000000000 ) ) ;
#23960=ORIENTED_EDGE ( 'NONE', *, *, #10296, .F. ) ;
#23961=DIRECTION ( 'NONE',  ( 1.000000000000000000, 0.000000000000000000, 0.000000000000000000 ) ) ;
#23962=CARTESIAN_POINT ( 'NONE',  ( 118.6910030610041815, 140.0000000000000000, 100.0000000000000000 ) ) ;
#23965=VERTEX_POINT ( 'NONE', #3022 ) ;
#23967=CARTESIAN_POINT ( 'NONE',  ( 89.82706236707214487, 239.6935390654258242, -16.61376038145277434 ) ) ;
#23969=CARTESIAN_POINT ( 'NONE',  ( -11.65927247860673255, 131.4491652140310407, -14.75293135532740152 ) ) ;
#23976=CARTESIAN_POINT ( 'NONE',  ( -140.1213116003368668, 122.5384136796733827, -13.00000000000000000 ) ) ;
#23982=EDGE_CURVE ( 'NONE', #5063, #606, #22992, .T. ) ;
#23986=DIRECTION ( 'NONE',  ( 1.000000000000000000, 0.000000000000000000, -0.000000000000000000 ) ) ;
#23987=CARTESIAN_POINT ( 'NONE',  ( 48.45469728424486533, 192.9461374953035033, -15.00000000000000000 ) ) ;
#23989=AXIS2_PLACEMENT_3D ( 'NONE', #16053, #18892, #25219 ) ;
#23993=DIRECTION ( 'NONE',  ( 0.000000000000000000, 0.000000000000000000, -1.000000000000000000 ) ) ;
#23997=EDGE_LOOP ( 'NONE', ( #158, #11514, #25571, #27906, #19295, #10687 ) ) ;
#23998=CARTESIAN_POINT ( 'NONE',  ( -173.6123854203675592, 113.7649492691934086, 27.03905483108168895 ) ) ;
#23999=CARTESIAN_POINT ( 'NONE',  ( -17.24491960465745777, -18.01420295945611727, 95.00000000000000000 ) ) ;
#24000=ORIENTED_EDGE ( 'NONE', *, *, #17717, .F. ) ;
#24001=PRODUCT_CONTEXT ( 'NONE', #8003, 'mechanical' ) ;
#24003=AXIS2_PLACEMENT_3D ( 'NONE', #19870, #13417, #342 ) ;
#24004=EDGE_LOOP ( 'NONE', ( #1861, #6719, #11734, #18701 ) ) ;
#24006=CYLINDRICAL_SURFACE ( 'NONE', #17072, 30.00000000000000000 ) ;
#24007=EDGE_CURVE ( 'NONE', #3920, #19657, #22852, .T. ) ;
#24011=CARTESIAN_POINT ( 'NONE',  ( 113.4920585194047078, 104.4775165427241461, -100.0000000000000142 ) ) ;
#24013=ORIENTED_EDGE ( 'NONE', *, *, #3883, .F. ) ;
#24014=EDGE_CURVE ( 'NONE', #7637, #28220, #20834, .T. ) ;
#24015=CARTESIAN_POINT ( 'NONE',  ( -223.2197326358865723, 88.62327920559705774, 14.89134622796188445 ) ) ;
#24017=DIRECTION ( 'NONE',  ( 0.000000000000000000, 0.000000000000000000, 1.000000000000000000 ) ) ;
#24018=EDGE_CURVE ( 'NONE', #15118, #12495, #14928, .T. ) ;
#24034=DIRECTION ( 'NONE',  ( -1.000000000000000000, -2.312964634635742957E-16, 0.000000000000000000 ) ) ;
#24038=SHAPE_REPRESENTATION ( 'Structural Component', ( #10637 ), #3285 ) ;
#24041=CARTESIAN_POINT ( 'NONE',  ( -160.5161435040798494, 120.3804527765386467, -22.28951900308574707 ) ) ;
#24045=CARTESIAN_POINT ( 'NONE',  ( -113.6546414130708058, 71.26467278202298417, 82.82413405842315512 ) ) ;
#24048=CARTESIAN_POINT ( 'NONE',  ( -71.37541315349507443, 230.0000000000000000, 15.00000000000000000 ) ) ;
#24052=CARTESIAN_POINT ( 'NONE',  ( -33.96955706545894316, 128.1973378200279399, 17.41747935847348572 ) ) ;
#24058=CARTESIAN_POINT ( 'NONE',  ( -209.9968668340340514, 60.57717296128767970, -21.99721431589914644 ) ) ;
#24062=DIRECTION ( 'NONE',  ( 1.000000000000000000, 2.602085213965211135E-16, 0.000000000000000000 ) ) ;
#24070=CARTESIAN_POINT ( 'NONE',  ( -244.5479615644635771, 75.99513337129096158, -5.000000000000004441 ) ) ;
#24071=LINE ( 'NONE', #23500, #2979 ) ;
#24073=CARTESIAN_POINT ( 'NONE',  ( 125.3433571860710600, 197.9412384757604570, 84.99999999999995737 ) ) ;
#24074=AXIS2_PLACEMENT_3D ( 'NONE', #12913, #8309, #1971 ) ;
#24076=CARTESIAN_POINT ( 'NONE',  ( -207.5044420441008128, 75.59897387903035337, 43.94429683754297855 ) ) ;
#24077=ORIENTED_EDGE ( 'NONE', *, *, #3145, .T. ) ;
#24082=EDGE_CURVE ( 'NONE', #12779, #25488, #1595, .T. ) ;
#24088=CARTESIAN_POINT ( 'NONE',  ( -101.3605996677730872, 134.2152826476940959, -15.56279420024448612 ) ) ;
#24089=CARTESIAN_POINT ( 'NONE',  ( 103.8044331943677321, 239.2408796538006186, 26.67200500018185494 ) ) ;
#24090=CARTESIAN_POINT ( 'NONE',  ( -37.82257053376181233, 36.92584315232891612, 99.00000000000000000 ) ) ;
#24091=LINE ( 'NONE', #28235, #4552 ) ;
#24092=AXIS2_PLACEMENT_3D ( 'NONE', #15891, #24636, #22047 ) ;
#24093=CARTESIAN_POINT ( 'NONE',  ( -68.57415822541635464, 24.64876300893806160, 100.0000000000000000 ) ) ;
#24096=EDGE_CURVE ( 'NONE', #25971, #7114, #19101, .T. ) ;
#24098=DIRECTION ( 'NONE',  ( 1.000000000000000000, 0.000000000000000000, 0.000000000000000000 ) ) ;
#24101=DIRECTION ( 'NONE',  ( -0.000000000000000000, -0.000000000000000000, 1.000000000000000000 ) ) ;
#24102=CARTESIAN_POINT ( 'NONE',  ( -200.0000000000000284, -91.18033988749901653, 0.000000000000000000 ) ) ;
#24105=CARTESIAN_POINT ( 'NONE',  ( -210.0000000000000284, -40.00000000000005684, -70.00000000000001421 ) ) ;
#24106=CARTESIAN_POINT ( 'NONE',  ( -160.0000000000000284, 59.99999999999994316, -70.00000000000001421 ) ) ;
#24107=PLANE ( 'NONE',  #16732 ) ;
#24109=DIRECTION ( 'NONE',  ( -0.000000000000000000, -0.000000000000000000, -1.000000000000000000 ) ) ;
#24111=AXIS2_PLACEMENT_3D ( 'NONE', #11609, #24946, #14046 ) ;
#24117=VECTOR ( 'NONE', #38, 1000.000000000000000 ) ;
#24121=ORIENTED_EDGE ( 'NONE', *, *, #14051, .T. ) ;
#24125=AXIS2_PLACEMENT_3D ( 'NONE', #5055, #2908, #11691 ) ;
#24127=EDGE_CURVE ( 'NONE', #14873, #2828, #19244, .T. ) ;
#24128=CARTESIAN_POINT ( 'NONE',  ( -223.9727688501994578, 61.67225750692129793, 20.13450274023654529 ) ) ;
#24130=DIRECTION ( 'NONE',  ( 0.000000000000000000, 0.000000000000000000, -1.000000000000000000 ) ) ;
#24134=DIRECTION ( 'NONE',  ( 1.000000000000000000, 0.000000000000000000, 0.000000000000000000 ) ) ;
#24135=CARTESIAN_POINT ( 'NONE',  ( 119.9999999999998863, 330.0000000000000000, -100.0000000000000142 ) ) ;
#24137=DIRECTION ( 'NONE',  ( 1.000000000000000000, 0.000000000000000000, 0.000000000000000000 ) ) ;
#24138=CARTESIAN_POINT ( 'NONE',  ( -180.5664960625764195, 109.3611654016444419, 31.00115732394728241 ) ) ;
#24142=EDGE_CURVE ( 'NONE', #12217, #1063, #23844, .T. ) ;
#24143=CARTESIAN_POINT ( 'NONE',  ( -164.2459188995896682, 118.6424907086743161, 23.77112046045245108 ) ) ;
#24144=CARTESIAN_POINT ( 'NONE',  ( -203.7123084376263762, 92.59051442877377269, -28.49533127386492026 ) ) ;
#24156=CARTESIAN_POINT ( 'NONE',  ( 116.3389527600916722, 113.0483370489294686, -100.0000000000000142 ) ) ;
#24157=DIRECTION ( 'NONE',  ( 1.000000000000000000, 0.000000000000000000, 0.000000000000000000 ) ) ;
#24158=ORIENTED_EDGE ( 'NONE', *, *, #27140, .F. ) ;
#24159=CARTESIAN_POINT ( 'NONE',  ( -215.4422302146570871, 87.87472848447453089, 19.21920766392561575 ) ) ;
#24162=EDGE_CURVE ( 'NONE', #21449, #8519, #5278, .T. ) ;
#24166=FACE_OUTER_BOUND ( 'NONE', #933, .T. ) ;
#24168=B_SPLINE_CURVE_WITH_KNOTS ( 'NONE', 3,
 ( #3069, #10256, #6354, #19577, #3775, #23462, #15135, #25747, #3916, #19013, #23891, #28316, #4196, #23744, #8236, #12564, #21442, #8661, #4339, #12842, #8378, #27758, #5934, #16995, #10534, #4053, #14708, #12987, #17417, #1756 ),
 .UNSPECIFIED., .F., .F.,
 ( 4, 2, 2, 2, 2, 2, 2, 2, 2, 2, 2, 2, 2, 2, 4 ),
 ( 0.000000000000000000, 0.004470907159210596622, 0.005588633949013227346, 0.006706360738815858938, 0.008941814318421193244, 0.01117726789802652755, 0.01341272147763186012, 0.01788362863684252527, 0.02011908221644785957, 0.02235453579605319388, 0.02682544295526392841, 0.02906089653486926619, 0.03129635011447460397, 0.03353180369407994521, 0.03576725727368528646 ),
 .UNSPECIFIED. ) ;
#24169=CARTESIAN_POINT ( 'NONE',  ( 79.99999999999992895, 110.0000000000000000, -70.00000000000001421 ) ) ;
#24174=DIRECTION ( 'NONE',  ( -0.000000000000000000, 1.000000000000000000, -0.000000000000000000 ) ) ;
#24178=CARTESIAN_POINT ( 'NONE',  ( 134.9999999999998579, 220.0000000000000284, 100.0000000000000142 ) ) ;
#24180=CARTESIAN_POINT ( 'NONE',  ( -188.6978706431725357, 104.3090321516409631, -31.95341200857410158 ) ) ;
#24181=ORIENTED_EDGE ( 'NONE', *, *, #12839, .F. ) ;
#24182=CIRCLE ( 'NONE', #19129, 16.46313063346208239 ) ;
#24183=EDGE_LOOP ( 'NONE', ( #6817, #21992, #23060, #16322, #24790 ) ) ;
#24198=LINE ( 'NONE', #24628, #8672 ) ;
#24200=CIRCLE ( 'NONE', #11831, 30.00000000000000000 ) ;
#24201=VERTEX_POINT ( 'NONE', #11199 ) ;
#24203=ORIENTED_EDGE ( 'NONE', *, *, #10194, .T. ) ;
#24204=FACE_OUTER_BOUND ( 'NONE', #15581, .T. ) ;
#24206=CARTESIAN_POINT ( 'NONE',  ( -40.40953891503691153, 0.000000000000000000, 99.00000000000000000 ) ) ;
#24213=ORIENTED_EDGE ( 'NONE', *, *, #27341, .T. ) ;
#24217=ORIENTED_EDGE ( 'NONE', *, *, #20062, .F. ) ;
#24219=AXIS2_PLACEMENT_3D ( 'NONE', #14079, #568, #22691 ) ;
#24220=ORIENTED_EDGE ( 'NONE', *, *, #26001, .T. ) ;
#24223=CARTESIAN_POINT ( 'NONE',  ( 91.17299970895479078, 230.3777436784795043, 17.14176051628196262 ) ) ;
#24228=DIRECTION ( 'NONE',  ( -0.000000000000000000, -0.000000000000000000, -1.000000000000000000 ) ) ;
#24230=CARTESIAN_POINT ( 'NONE',  ( -160.0000000000000284, 59.99999999999994316, -45.00000000000000000 ) ) ;
#24235=DIRECTION ( 'NONE',  ( -1.000000000000000000, -0.000000000000000000, 0.000000000000000000 ) ) ;
#24236=TOROIDAL_SURFACE ( 'NONE', #20111, 30.49120955644046660, 2.000000000000000000 ) ;
#24237=EDGE_CURVE ( 'NONE', #13747, #1725, #23628, .T. ) ;
#24240=CARTESIAN_POINT ( 'NONE',  ( -63.57415822541634043, 0.000000000000000000, 100.0000000000000000 ) ) ;
#24243=CARTESIAN_POINT ( 'NONE',  ( 107.7175597583449189, 250.4128021204703600, -33.27520275791160742 ) ) ;
#24244=ORIENTED_EDGE ( 'NONE', *, *, #17079, .F. ) ;
#24246=VERTEX_POINT ( 'NONE', #23987 ) ;
#24249=EDGE_CURVE ( 'NONE', #23784, #1799, #4147, .T. ) ;
#24257=FACE_OUTER_BOUND ( 'NONE', #18503, .T. ) ;
#24259=EDGE_CURVE ( 'NONE', #24930, #15707, #1997, .T. ) ;
#24260=CARTESIAN_POINT ( 'NONE',  ( -198.1081924558745584, 61.84288891412396083, 30.88603804298443833 ) ) ;
#24267=ADVANCED_FACE ( 'NONE', ( #4717 ), #4299, .T. ) ;
#24269=CARTESIAN_POINT ( 'NONE',  ( -3.472619751711179426, 132.8132803667743644, 15.86983229809730389 ) ) ;
#24271=DIRECTION ( 'NONE',  ( -1.000000000000000000, -1.321694076934710155E-16, 0.000000000000000000 ) ) ;
#24273=VERTEX_POINT ( 'NONE', #2137 ) ;
#24275=CARTESIAN_POINT ( 'NONE',  ( -230.2711638029755932, 89.63949233591094412, -15.23082775398237487 ) ) ;
#24276=CIRCLE ( 'NONE', #19231, 1.999999999999996891 ) ;
#24277=CARTESIAN_POINT ( 'NONE',  ( -206.1524755872160881, 90.88176262967643027, -27.63232739364782020 ) ) ;
#24282=LINE ( 'NONE', #17964, #3297 ) ;
#24284=CARTESIAN_POINT ( 'NONE',  ( -160.8326600028555617, 120.2355194873574931, 21.37420696376539908 ) ) ;
#24285=ORIENTED_EDGE ( 'NONE', *, *, #14133, .F. ) ;
#24286=DIRECTION ( 'NONE',  ( -3.469446951953614189E-16, 1.000000000000000000, -0.000000000000000000 ) ) ;
#24289=AXIS2_PLACEMENT_3D ( 'NONE', #23439, #18988, #25729 ) ;
#24291=CARTESIAN_POINT ( 'NONE',  ( -209.6188097997069519, 88.33184316452725682, 25.56917691525033121 ) ) ;
#24293=EDGE_CURVE ( 'NONE', #4321, #18978, #26548, .T. ) ;
#24297=EDGE_CURVE ( 'NONE', #5984, #2640, #25445, .T. ) ;
#24299=PLANE ( 'NONE',  #13696 ) ;
#24301=CARTESIAN_POINT ( 'NONE',  ( -217.6530384384032573, 140.9974917369195566, -15.00000000000000000 ) ) ;
#24306=VECTOR ( 'NONE', #10276, 1000.000000000000000 ) ;
#24307=CARTESIAN_POINT ( 'NONE',  ( -236.8667578982872044, 138.8517089611673043, 15.00000000000000000 ) ) ;
#24312=DIRECTION ( 'NONE',  ( -0.7730186417261840637, -0.6343833064826071011, 0.000000000000000000 ) ) ;
#24313=CYLINDRICAL_SURFACE ( 'NONE', #12673, 30.00000000000000000 ) ;
#24315=ORIENTED_EDGE ( 'NONE', *, *, #2306, .F. ) ;
#24316=CARTESIAN_POINT ( 'NONE',  ( -111.6450422266150326, 69.94128127818710539, 82.90302649402674717 ) ) ;
#24317=CARTESIAN_POINT ( 'NONE',  ( -71.37541315349507443, 150.2892445414773590, 5.000000000000002665 ) ) ;
#24319=ORIENTED_EDGE ( 'NONE', *, *, #15619, .T. ) ;
#24328=CARTESIAN_POINT ( 'NONE',  ( -208.6311953968240687, 71.65302225189010699, -39.58319495383710773 ) ) ;
#24329=AXIS2_PLACEMENT_3D ( 'NONE', #23743, #17138, #12986 ) ;
#24344=ORIENTED_EDGE ( 'NONE', *, *, #1654, .F. ) ;
#24345=CIRCLE ( 'NONE', #26637, 22.49999999999999289 ) ;
#24357=CARTESIAN_POINT ( 'NONE',  ( -218.8273392347107063, 140.3457761587386869, 14.99191580167233973 ) ) ;
#24358=CARTESIAN_POINT ( 'NONE',  ( 91.79864198314062662, 239.6982472080604794, 17.32810371389381388 ) ) ;
#24359=CARTESIAN_POINT ( 'NONE',  ( -210.0000000000000284, -40.00000000000005684, 100.0000000000000142 ) ) ;
#24360=ADVANCED_FACE ( 'NONE', ( #1124 ), #13571, .T. ) ;
#24362=EDGE_CURVE ( 'NONE', #4407, #16727, #10065, .T. ) ;
#24366=DIRECTION ( 'NONE',  ( -0.000000000000000000, -0.000000000000000000, 1.000000000000000000 ) ) ;
#24367=CIRCLE ( 'NONE', #26207, 24.07986109634097005 ) ;
#24371=CARTESIAN_POINT ( 'NONE',  ( 115.6411010564591777, 231.4666050640012429, -99.00000000000001421 ) ) ;
#24373=FACE_OUTER_BOUND ( 'NONE', #15920, .T. ) ;
#24376=CIRCLE ( 'NONE', #977, 30.00000000000000000 ) ;
#24379=DIRECTION ( 'NONE',  ( 1.000000000000000000, 0.000000000000000000, 0.000000000000000000 ) ) ;
#24382=VERTEX_POINT ( 'NONE', #25534 ) ;
#24395=EDGE_CURVE ( 'NONE', #23197, #17312, #25398, .T. ) ;
#24397=EDGE_CURVE ( 'NONE', #26863, #19837, #20342, .T. ) ;
#24401=CARTESIAN_POINT ( 'NONE',  ( -215.3329573320907571, 58.91837420258404023, 30.17944279517852024 ) ) ;
#24405=CARTESIAN_POINT ( 'NONE',  ( -221.3650667873343139, -91.18033988749901653, 14.94182580522077330 ) ) ;
#24406=CARTESIAN_POINT ( 'NONE',  ( 93.99999999999985789, 268.4896896257338312, -84.99999999999997158 ) ) ;
#24410=AXIS2_PLACEMENT_3D ( 'NONE', #12940, #2424, #25994 ) ;
#24411=CARTESIAN_POINT ( 'NONE',  ( 9.345921402568903247, 140.0000000000000000, 14.99999999999999467 ) ) ;
#24412=DIRECTION ( 'NONE',  ( -1.000000000000000000, 0.000000000000000000, 0.000000000000000000 ) ) ;
#24413=LINE ( 'NONE', #26557, #3714 ) ;
#24414=FACE_OUTER_BOUND ( 'NONE', #19867, .T. ) ;
#24419=CARTESIAN_POINT ( 'NONE',  ( -211.1098990695232374, 87.67290574086477761, -24.45168726860073605 ) ) ;
#24422=CARTESIAN_POINT ( 'NONE',  ( -206.8748453633142219, 90.47121226081961254, -26.13154464733097981 ) ) ;
#24427=DIRECTION ( 'NONE',  ( 1.000000000000000000, 0.000000000000000000, 0.000000000000000000 ) ) ;
#24428=CARTESIAN_POINT ( 'NONE',  ( -149.3148642887314850, 125.0486274829139717, 18.95245273128049490 ) ) ;
#24429=ORIENTED_EDGE ( 'NONE', *, *, #25406, .T. ) ;
#24437=CARTESIAN_POINT ( 'NONE',  ( -204.4606010538157079, 92.01149164604352393, 28.73671646131870361 ) ) ;
#24442=CARTESIAN_POINT ( 'NONE',  ( -212.2468527728169931, 60.00277588997245459, -15.59298365947654297 ) ) ;
#24444=EDGE_CURVE ( 'NONE', #23655, #8985, #1404, .T. ) ;
#24447=CARTESIAN_POINT ( 'NONE',  ( -222.2072112174627136, 138.1987073436359026, -14.97424725141360291 ) ) ;
#24449=DIRECTION ( 'NONE',  ( 0.5555587585212703461, 0.8314772792026879911, -0.000000000000000000 ) ) ;
#24451=AXIS2_PLACEMENT_3D ( 'NONE', #9952, #7661, #7796 ) ;
#24453=CIRCLE ( 'NONE', #28107, 19.07743405327024888 ) ;
#24456=EDGE_LOOP ( 'NONE', ( #25690, #14333, #10272, #2693 ) ) ;
#24457=CIRCLE ( 'NONE', #27221, 23.59849023212046149 ) ;
#24461=EDGE_CURVE ( 'NONE', #3789, #8411, #13188, .T. ) ;
#24463=CARTESIAN_POINT ( 'NONE',  ( -203.1779787704217313, 93.05164332230199875, -28.77272332722132120 ) ) ;
#24465=ORIENTED_EDGE ( 'NONE', *, *, #20568, .F. ) ;
#24468=VERTEX_POINT ( 'NONE', #19498 ) ;
#24475=FACE_OUTER_BOUND ( 'NONE', #28045, .T. ) ;
#24476=VECTOR ( 'NONE', #11991, 1000.000000000000000 ) ;
#24478=CARTESIAN_POINT ( 'NONE',  ( -208.0819832607409410, 73.72223769926478099, -42.22193701883060868 ) ) ;
#24479=DIRECTION ( 'NONE',  ( 0.000000000000000000, 0.000000000000000000, -1.000000000000000000 ) ) ;
#24480=ORIENTED_EDGE ( 'NONE', *, *, #16314, .T. ) ;
#24484=CARTESIAN_POINT ( 'NONE',  ( 134.9999999999998579, -150.0000000000000284, 84.99999999999995737 ) ) ;
#24488=VERTEX_POINT ( 'NONE', #10744 ) ;
#24490=CARTESIAN_POINT ( 'NONE',  ( -226.5998460896584561, 62.96930358458838128, -8.263950894743111064 ) ) ;
#24495=ORIENTED_EDGE ( 'NONE', *, *, #4234, .F. ) ;
#24497=CARTESIAN_POINT ( 'NONE',  ( -229.8570707599101297, 74.77602913581384314, 16.24303275925431933 ) ) ;
#24499=CARTESIAN_POINT ( 'NONE',  ( -175.0000000000000000, -120.0000000000001847, -76.02499999999999147 ) ) ;
#24508=EDGE_LOOP ( 'NONE', ( #4746, #12674, #25382, #14786 ) ) ;
#24510=CARTESIAN_POINT ( 'NONE',  ( 105.5907556405553720, 242.1385898947461328, 29.32397797499837466 ) ) ;
#24512=CARTESIAN_POINT ( 'NONE',  ( -221.1044245926312044, 138.9463871349868782, -14.97905406095859249 ) ) ;
#24515=CARTESIAN_POINT ( 'NONE',  ( -160.0000000000000284, 59.99999999999994316, 15.00000000000000000 ) ) ;
#24521=CARTESIAN_POINT ( 'NONE',  ( 65.00000000000000000, -150.0000000000000568, 70.00000000000001421 ) ) ;
#24527=CARTESIAN_POINT ( 'NONE',  ( -28.05246235954390244, 188.0718642840173516, 15.00000000000000000 ) ) ;
#24528=ORIENTED_EDGE ( 'NONE', *, *, #24096, .T. ) ;
#24529=CARTESIAN_POINT ( 'NONE',  ( 109.9639884629222877, 258.5863491989132967, -43.28603914697800548 ) ) ;
#24530=VERTEX_POINT ( 'NONE', #15625 ) ;
#24531=DIRECTION ( 'NONE',  ( 0.000000000000000000, 0.000000000000000000, 1.000000000000000000 ) ) ;
#24534=ORIENTED_EDGE ( 'NONE', *, *, #10319, .T. ) ;
#24537=ORIENTED_EDGE ( 'NONE', *, *, #26992, .F. ) ;
#24540=ORIENTED_EDGE ( 'NONE', *, *, #8298, .F. ) ;
#24541=CARTESIAN_POINT ( 'NONE',  ( 119.9999999999998863, 330.0000000000000000, -90.00000000000004263 ) ) ;
#24546=CARTESIAN_POINT ( 'NONE',  ( -220.5757601432209185, 60.53190028572070958, 22.93231238515498305 ) ) ;
#24550=AXIS2_PLACEMENT_3D ( 'NONE', #9991, #3372, #3794 ) ;
#24551=CARTESIAN_POINT ( 'NONE',  ( -219.7365213294408477, 87.93330934136336907, -16.54735205736179893 ) ) ;
#24557=CARTESIAN_POINT ( 'NONE',  ( -1.097484912870223539, 135.6466149407013688, 15.26443675455116455 ) ) ;
#24558=PLANE ( 'NONE',  #1352 ) ;
#24561=CIRCLE ( 'NONE', #24092, 1.999999999999990452 ) ;
#24565=EDGE_CURVE ( 'NONE', #17857, #13481, #17761, .T. ) ;
#24572=CARTESIAN_POINT ( 'NONE',  ( -122.8162676995331708, 132.7862067426565886, 15.82969067823930587 ) ) ;
#24577=AXIS2_PLACEMENT_3D ( 'NONE', #27443, #21131, #3598 ) ;
#24578=LINE ( 'NONE', #7200, #20050 ) ;
#24586=CARTESIAN_POINT ( 'NONE',  ( -210.0090741174316804, 73.93180346605655018, -34.41452853221989727 ) ) ;
#24588=DIRECTION ( 'NONE',  ( 0.000000000000000000, -1.000000000000000000, 0.000000000000000000 ) ) ;
#24590=ADVANCED_FACE ( 'NONE', ( #19773 ), #23652, .F. ) ;
#24591=CARTESIAN_POINT ( 'NONE',  ( -217.7401460507702780, 138.5677444271782122, -12.99353264123096885 ) ) ;
#24593=LINE ( 'NONE', #20132, #7554 ) ;
#24596=CARTESIAN_POINT ( 'NONE',  ( -63.57415822541634043, 80.97823757117562593, 100.0000000000000000 ) ) ;
#24598=CARTESIAN_POINT ( 'NONE',  ( -227.3197243376772860, 73.27520359174637576, 17.23934621637404163 ) ) ;
#24603=EDGE_LOOP ( 'NONE', ( #7446, #18705, #27726, #2913, #8769, #14836, #8763, #3859, #5168, #24632 ) ) ;
#24604=CARTESIAN_POINT ( 'NONE',  ( 90.92319367352486381, 112.0484670279021771, 72.65625000014701129 ) ) ;
#24608=VERTEX_POINT ( 'NONE', #4539 ) ;
#24609=DIRECTION ( 'NONE',  ( 0.000000000000000000, 0.000000000000000000, 1.000000000000000000 ) ) ;
#24612=ORIENTED_EDGE ( 'NONE', *, *, #4213, .T. ) ;
#24616=FACE_BOUND ( 'NONE', #9203, .T. ) ;
#24619=CARTESIAN_POINT ( 'NONE',  ( -20.28198206961980787, 129.6360743166005705, -16.81503550425660265 ) ) ;
#24620=VECTOR ( 'NONE', #3378, 1000.000000000000000 ) ;
#24625=ORIENTED_EDGE ( 'NONE', *, *, #3111, .F. ) ;
#24627=CARTESIAN_POINT ( 'NONE',  ( -223.3099978423093432, 137.4510275522739562, 14.96944044186858491 ) ) ;
#24628=CARTESIAN_POINT ( 'NONE',  ( 9.999999999999749534, 90.00000000000001421, 110.0000000000000284 ) ) ;
#24629=CARTESIAN_POINT ( 'NONE',  ( -248.1546605714623013, -91.18033988749901653, -16.91094714394370158 ) ) ;
#24631=CARTESIAN_POINT ( 'NONE',  ( -229.6839157287631963, 64.28192771017235430, 7.255073467994254344 ) ) ;
#24632=ORIENTED_EDGE ( 'NONE', *, *, #17358, .T. ) ;
#24635=DIRECTION ( 'NONE',  ( -1.000000000000000000, 0.000000000000000000, 0.000000000000000000 ) ) ;
#24636=DIRECTION ( 'NONE',  ( -0.5790253867566403922, -0.8153095126952237814, -0.000000000000000000 ) ) ;
#24639=LINE ( 'NONE', #22773, #8831 ) ;
#24643=ORIENTED_EDGE ( 'NONE', *, *, #3709, .T. ) ;
#24647=ADVANCED_FACE ( 'NONE', ( #7424 ), #6988, .F. ) ;
#24648=LINE ( 'NONE', #12007, #3971 ) ;
#24651=ORIENTED_EDGE ( 'NONE', *, *, #17172, .F. ) ;
#24652=ORIENTED_EDGE ( 'NONE', *, *, #4570, .T. ) ;
#24653=CARTESIAN_POINT ( 'NONE',  ( 105.7413873646089684, 247.3652972445288469, 29.41146778675347662 ) ) ;
#24655=CARTESIAN_POINT ( 'NONE',  ( -225.3736415174282115, 135.7651958811247539, -14.97905406095859604 ) ) ;
#24659=DIRECTION ( 'NONE',  ( -1.000000000000000000, 0.000000000000000000, 0.000000000000000000 ) ) ;
#24661=CYLINDRICAL_SURFACE ( 'NONE', #755, 22.49999999999999289 ) ;
#24662=CARTESIAN_POINT ( 'NONE',  ( 65.00000000000000000, -120.0000000000000711, 76.02500000000001990 ) ) ;
#24673=VERTEX_POINT ( 'NONE', #26954 ) ;
#24683=ORIENTED_EDGE ( 'NONE', *, *, #9189, .T. ) ;
#24684=CARTESIAN_POINT ( 'NONE',  ( -62.44394432210693680, 134.9077315552440837, 13.78060465110143262 ) ) ;
#24685=DIRECTION ( 'NONE',  ( -0.000000000000000000, 1.000000000000000000, -1.387778780781445429E-16 ) ) ;
#24688=PRODUCT_DEFINITION_CONTEXT ( 'detailed design', #23235, 'design' ) ;
#24689=FACE_OUTER_BOUND ( 'NONE', #22433, .T. ) ;
#24690=CARTESIAN_POINT ( 'NONE',  ( -222.1843861435932581, 71.54148064075766911, 20.10873357379271908 ) ) ;
#24693=FACE_OUTER_BOUND ( 'NONE', #2027, .T. ) ;
#24694=CARTESIAN_POINT ( 'NONE',  ( 79.99999999999995737, 102.6016043537709379, -89.82480251742194355 ) ) ;
#24696=CARTESIAN_POINT ( 'NONE',  ( -214.0809518536805172, 88.01152685125013875, -20.18792008739580268 ) ) ;
#24701=EDGE_CURVE ( 'NONE', #14569, #20039, #2063, .T. ) ;
#24703=CARTESIAN_POINT ( 'NONE',  ( 5.596985676125543208, 137.4248447260847854, 15.08939176349822020 ) ) ;
#24707=ORIENTED_EDGE ( 'NONE', *, *, #9979, .T. ) ;
#24709=DIRECTION ( 'NONE',  ( 0.000000000000000000, 0.000000000000000000, -1.000000000000000000 ) ) ;
#24713=ORIENTED_EDGE ( 'NONE', *, *, #7052, .T. ) ;
#24716=CARTESIAN_POINT ( 'NONE',  ( -142.3006454101396514, 127.5200935965802387, 17.68125478821149699 ) ) ;
#24717=EDGE_CURVE ( 'NONE', #20004, #2614, #11463, .T. ) ;
#24723=ADVANCED_FACE ( 'NONE', ( #4967 ), #18142, .T. ) ;
#24727=CARTESIAN_POINT ( 'NONE',  ( -17.24491960465746132, -23.01420295945612082, 100.0000000000000000 ) ) ;
#24732=CARTESIAN_POINT ( 'NONE',  ( -208.0231409554068875, 75.22252239880569391, -40.22632386312260167 ) ) ;
#24734=AXIS2_PLACEMENT_3D ( 'NONE', #27568, #12516, #16954 ) ;
#24736=EDGE_CURVE ( 'NONE', #1342, #24933, #15399, .T. ) ;
#24737=CIRCLE ( 'NONE', #12359, 5.000000000000004441 ) ;
#24738=CARTESIAN_POINT ( 'NONE',  ( -220.9647007329185158, 136.4514858755404987, -12.97939780113087060 ) ) ;
#24746=CARTESIAN_POINT ( 'NONE',  ( 65.00000000000000000, -120.0000000000000711, 76.00000000000001421 ) ) ;
#24748=ORIENTED_EDGE ( 'NONE', *, *, #1174, .T. ) ;
#24749=CARTESIAN_POINT ( 'NONE',  ( 107.3061218092289408, 127.3934823308085242, 87.81249999970602005 ) ) ;
#24753=ORIENTED_EDGE ( 'NONE', *, *, #5069, .F. ) ;
#24755=AXIS2_PLACEMENT_3D ( 'NONE', #14082, #22403, #3132 ) ;
#24765=CARTESIAN_POINT ( 'NONE',  ( -13.80312808312014816, 130.8720850416648318, -14.97150579888662492 ) ) ;
#24766=CARTESIAN_POINT ( 'NONE',  ( -110.3221550338875687, 20.24192588826928585, 83.00000000000001421 ) ) ;
#24768=DIRECTION ( 'NONE',  ( 1.000000000000000000, 0.000000000000000000, 0.000000000000000000 ) ) ;
#24770=VECTOR ( 'NONE', #466, 1000.000000000000000 ) ;
#24771=DIRECTION ( 'NONE',  ( -0.000000000000000000, 1.000000000000000000, -1.387778780781445429E-16 ) ) ;
#24777=CARTESIAN_POINT ( 'NONE',  ( -239.7229382034103935, 70.94047833162915140, 5.249966640536482210 ) ) ;
#24778=CIRCLE ( 'NONE', #22477, 2.000000000000000000 ) ;
#24782=CARTESIAN_POINT ( 'NONE',  ( -17.24491960465747553, 80.97823757117562593, 80.00000000000001421 ) ) ;
#24783=DIRECTION ( 'NONE',  ( 1.000000000000000000, 1.541976423090495387E-16, -0.000000000000000000 ) ) ;
#24785=DIRECTION ( 'NONE',  ( 0.000000000000000000, 0.000000000000000000, -1.000000000000000000 ) ) ;
#24787=CARTESIAN_POINT ( 'NONE',  ( -47.90464318815075018, 130.8803359162888569, 16.39305836622124346 ) ) ;
#24790=ORIENTED_EDGE ( 'NONE', *, *, #2274, .T. ) ;
#24793=ORIENTED_EDGE ( 'NONE', *, *, #6497, .F. ) ;
#24794=AXIS2_PLACEMENT_3D ( 'NONE', #11743, #18051, #5108 ) ;
#24795=ORIENTED_EDGE ( 'NONE', *, *, #6193, .T. ) ;
#24802=CARTESIAN_POINT ( 'NONE',  ( 109.9999999999999005, 260.0000000000000000, -45.00000000000000000 ) ) ;
#24806=CARTESIAN_POINT ( 'NONE',  ( -160.0000000000000284, 59.99999999999994316, -15.00000000000000000 ) ) ;
#24808=CARTESIAN_POINT ( 'NONE',  ( -175.0000000000000000, -120.0000000000001705, 70.00000000000001421 ) ) ;
#24816=FACE_OUTER_BOUND ( 'NONE', #6920, .T. ) ;
#24818=ORIENTED_EDGE ( 'NONE', *, *, #27695, .F. ) ;
#24829=CARTESIAN_POINT ( 'NONE',  ( -156.4100387916780335, 122.2070193974234229, 19.70550239271524973 ) ) ;
#24833=CARTESIAN_POINT ( 'NONE',  ( -52.57787683962911984, 133.2861237126421088, -15.71127553108205177 ) ) ;
#24834=EDGE_CURVE ( 'NONE', #1913, #4814, #25796, .T. ) ;
#24836=CIRCLE ( 'NONE', #18414, 39.99999999999999289 ) ;
#24837=CARTESIAN_POINT ( 'NONE',  ( -214.0051257764050945, 55.38571953469081421, 43.60894023861363422 ) ) ;
#24839=CARTESIAN_POINT ( 'NONE',  ( -149.4295825701717320, 124.9919708967672989, -17.80889158364129798 ) ) ;
#24840=DIRECTION ( 'NONE',  ( -1.000000000000000000, 0.000000000000000000, 0.000000000000000000 ) ) ;
#24846=CARTESIAN_POINT ( 'NONE',  ( 117.1152841538456926, 116.0550883417529491, -100.0000000000000142 ) ) ;
#24852=LINE ( 'NONE', #17278, #2866 ) ;
#24856=AXIS2_PLACEMENT_3D ( 'NONE', #24527, #19783, #17918 ) ;
#24858=CARTESIAN_POINT ( 'NONE',  ( -151.8743502727079999, 124.0639289416861288, 18.38162538368994703 ) ) ;
#24860=ORIENTED_EDGE ( 'NONE', *, *, #13484, .F. ) ;
#24861=CARTESIAN_POINT ( 'NONE',  ( -169.4361096980427135, 115.4683091757704005, -26.67336330034965997 ) ) ;
#24862=CARTESIAN_POINT ( 'NONE',  ( 124.9999999999998579, 220.0000000000000284, -90.00000000000002842 ) ) ;
#24866=LINE ( 'NONE', #20407, #5459 ) ;
#24871=CARTESIAN_POINT ( 'NONE',  ( 3.469446951953618133E-15, -40.00000000000003553, -100.0000000000000142 ) ) ;
#24872=CARTESIAN_POINT ( 'NONE',  ( -214.1250002713545086, 55.22895589251590565, -44.08339233875913976 ) ) ;
#24873=FACE_OUTER_BOUND ( 'NONE', #12543, .T. ) ;
#24876=DIRECTION ( 'NONE',  ( 0.000000000000000000, 0.000000000000000000, 1.000000000000000000 ) ) ;
#24880=CARTESIAN_POINT ( 'NONE',  ( -242.5499235585427584, 73.68467268308823748, 14.74213902348265393 ) ) ;
#24891=EDGE_CURVE ( 'NONE', #6895, #19138, #16786, .T. ) ;
#24892=CARTESIAN_POINT ( 'NONE',  ( -279.3160071107327553, -512.7211954420570237, 0.000000000000000000 ) ) ;
#24897=DIRECTION ( 'NONE',  ( 0.000000000000000000, 0.000000000000000000, -1.000000000000000000 ) ) ;
#24901=CARTESIAN_POINT ( 'NONE',  ( 157.4999999999998579, 220.0000000000000284, -105.0000000000000284 ) ) ;
#24904=CARTESIAN_POINT ( 'NONE',  ( -18.15357532044453137, 129.9610192713841741, -15.33575750053543985 ) ) ;
#24912=AXIS2_PLACEMENT_3D ( 'NONE', #7836, #12307, #7421 ) ;
#24916=CARTESIAN_POINT ( 'NONE',  ( -146.6428522700808230, 69.54464929955099706, 83.00000000000001421 ) ) ;
#24919=DIRECTION ( 'NONE',  ( 1.000000000000000000, -0.000000000000000000, -0.000000000000000000 ) ) ;
#24922=CARTESIAN_POINT ( 'NONE',  ( -112.3221550338875687, 69.54464929955099706, 83.00000000000001421 ) ) ;
#24923=ORIENTED_EDGE ( 'NONE', *, *, #587, .T. ) ;
#24927=CARTESIAN_POINT ( 'NONE',  ( 89.99999999999988631, 240.0000000000000284, 6.270166537925822681 ) ) ;
#24930=VERTEX_POINT ( 'NONE', #1941 ) ;
#24933=VERTEX_POINT ( 'NONE', #17315 ) ;
#24936=VERTEX_POINT ( 'NONE', #10577 ) ;
#24946=DIRECTION ( 'NONE',  ( 1.530283246943720875E-16, -1.000000000000000000, 0.000000000000000000 ) ) ;
#24947=CARTESIAN_POINT ( 'NONE',  ( -190.0000000000000284, -40.00000000000004974, 98.28427124746191623 ) ) ;
#24955=CARTESIAN_POINT ( 'NONE',  ( -143.6428522700808230, 20.24192588826928585, 93.88690167569083656 ) ) ;
#24959=CARTESIAN_POINT ( 'NONE',  ( 134.9999999999998579, 268.4896896257338881, 84.99999999999995737 ) ) ;
#24960=ORIENTED_EDGE ( 'NONE', *, *, #205, .T. ) ;
#24964=ORIENTED_EDGE ( 'NONE', *, *, #3904, .F. ) ;
#24965=B_SPLINE_CURVE_WITH_KNOTS ( 'NONE', 3,
 ( #7522, #16423, #11407, #4394, #15866, #1601, #1321, #14835, #12261, #8073, #3607, #3748, #3896, #28017, #5772, #14546, #12402, #8214, #10092, #23302, #14268, #21138 ),
 .UNSPECIFIED., .F., .F.,
 ( 4, 2, 2, 2, 2, 2, 2, 2, 2, 2, 4 ),
 ( 0.000000000000000000, 0.06249999999999987510, 0.1249999999999999306, 0.1875000000000000000, 0.2500000000000000555, 0.3750000000000000000, 0.5000000000000000000, 0.6250000000000000000, 0.7500000000000000000, 0.8750000000000001110, 1.000000000000000000 ),
 .UNSPECIFIED. ) ;
#24967=CARTESIAN_POINT ( 'NONE',  ( -77.61721128200930764, 136.2551396520290723, 13.51936372730774849 ) ) ;
#24969=CARTESIAN_POINT ( 'NONE',  ( 179.9999999999999147, 0.000000000000000000, 84.99999999999995737 ) ) ;
#24970=FACE_OUTER_BOUND ( 'NONE', #26560, .T. ) ;
#24972=DIRECTION ( 'NONE',  ( 0.000000000000000000, 0.000000000000000000, -1.000000000000000000 ) ) ;
#24975=CARTESIAN_POINT ( 'NONE',  ( -23.64013312899696828, 129.3207233730292955, 15.61661841831484132 ) ) ;
#24976=CARTESIAN_POINT ( 'NONE',  ( -207.5108889574473494, 75.59417117316073131, 44.26576816510100798 ) ) ;
#24978=CARTESIAN_POINT ( 'NONE',  ( -47.47907723713406369, 132.2277457862344932, -14.48493892500291835 ) ) ;
#24979=CARTESIAN_POINT ( 'NONE',  ( 79.99999999999995737, 87.77847705527369726, -99.04049946057673992 ) ) ;
#24985=PLANE ( 'NONE',  #24755 ) ;
#24986=CARTESIAN_POINT ( 'NONE',  ( -188.7721129603572194, 104.0449037398145009, 32.78712893570086351 ) ) ;
#24990=AXIS2_PLACEMENT_3D ( 'NONE', #10520, #4038, #14554 ) ;
#24991=EDGE_CURVE ( 'NONE', #9161, #12189, #15034, .T. ) ;
#24994=AXIS2_PLACEMENT_3D ( 'NONE', #7434, #2682, #9303 ) ;
#24997=CARTESIAN_POINT ( 'NONE',  ( -77.72059375409217807, 134.6165094220598917, 15.48686464813458841 ) ) ;
#25010=AXIS2_PLACEMENT_3D ( 'NONE', #2043, #25894, #17276 ) ;
#25011=CARTESIAN_POINT ( 'NONE',  ( 134.9999999999998579, 220.0000000000000284, -99.00000000000001421 ) ) ;
#25012=CARTESIAN_POINT ( 'NONE',  ( -213.4823095283139196, 56.20074567116226660, -41.47858424781075115 ) ) ;
#25020=CARTESIAN_POINT ( 'NONE',  ( -231.9378824387731299, 93.53122965655668963, -13.00000000000000000 ) ) ;
#25021=EDGE_CURVE ( 'NONE', #13173, #6225, #7148, .T. ) ;
#25022=CARTESIAN_POINT ( 'NONE',  ( -230.6867234551439196, 75.40543009380269268, 15.98884730490149764 ) ) ;
#25023=CARTESIAN_POINT ( 'NONE',  ( -68.57415822541635464, -23.01420295945612082, 95.00000000000000000 ) ) ;
#25033=AXIS2_PLACEMENT_3D ( 'NONE', #14115, #20846, #9934 ) ;
#25035=LINE ( 'NONE', #16138, #23261 ) ;
#25036=CYLINDRICAL_SURFACE ( 'NONE', #10201, 64.76834224489934400 ) ;
#25038=ORIENTED_EDGE ( 'NONE', *, *, #13201, .T. ) ;
#25042=DIRECTION ( 'NONE',  ( 1.000000000000000000, 0.000000000000000000, 0.000000000000000000 ) ) ;
#25045=CARTESIAN_POINT ( 'NONE',  ( 109.9999999999999147, 140.0000000000000000, -90.00000000000004263 ) ) ;
#25046=CARTESIAN_POINT ( 'NONE',  ( 6.408192432492758606, 140.2484972092699138, -14.93046625219126078 ) ) ;
#25049=DIRECTION ( 'NONE',  ( 0.8314772792026879911, -0.5555587585212703461, 0.000000000000000000 ) ) ;
#25053=CIRCLE ( 'NONE', #13604, 5.000000000000004441 ) ;
#25060=ORIENTED_EDGE ( 'NONE', *, *, #240, .T. ) ;
#25061=CARTESIAN_POINT ( 'NONE',  ( -217.2892621185082760, 109.4029876883478352, -13.00000000000000000 ) ) ;
#25065=CARTESIAN_POINT ( 'NONE',  ( 0.000000000000000000, 0.000000000000000000, 0.000000000000000000 ) ) ;
#25066=DIRECTION ( 'NONE',  ( 1.000000000000000000, 0.000000000000000000, 0.000000000000000000 ) ) ;
#25068=CARTESIAN_POINT ( 'NONE',  ( -67.66005108804499457, 133.9293368352053051, 15.61826086920359913 ) ) ;
#25069=CARTESIAN_POINT ( 'NONE',  ( 105.0441603316952381, 246.7663426280820147, 21.68296015126954401 ) ) ;
#25070=VERTEX_POINT ( 'NONE', #7263 ) ;
#25071=AXIS2_PLACEMENT_3D ( 'NONE', #19621, #86, #15184 ) ;
#25074=ORIENTED_EDGE ( 'NONE', *, *, #2331, .F. ) ;
#25084=DIRECTION ( 'NONE',  ( 0.7348549764921636918, -0.6782242722910333255, 0.000000000000000000 ) ) ;
#25091=EDGE_CURVE ( 'NONE', #7226, #5857, #4862, .T. ) ;
#25093=CYLINDRICAL_SURFACE ( 'NONE', #14000, 5.000000000000004441 ) ;
#25096=DIRECTION ( 'NONE',  ( -1.000000000000000000, 0.000000000000000000, 0.000000000000000000 ) ) ;
#25102=EDGE_LOOP ( 'NONE', ( #1250, #20982, #27452, #9315 ) ) ;
#25103=CARTESIAN_POINT ( 'NONE',  ( -144.8714485210765304, 126.6523762207952757, 16.84425668626998984 ) ) ;
#25105=DIRECTION ( 'NONE',  ( -0.000000000000000000, -0.000000000000000000, 1.000000000000000000 ) ) ;
#25108=CARTESIAN_POINT ( 'NONE',  ( -194.2478650485211062, 63.21120109188145619, 44.02102422013626892 ) ) ;
#25112=FACE_OUTER_BOUND ( 'NONE', #11769, .T. ) ;
#25120=DIRECTION ( 'NONE',  ( 0.000000000000000000, 0.000000000000000000, -1.000000000000000000 ) ) ;
#25128=ORIENTED_EDGE ( 'NONE', *, *, #18923, .F. ) ;
#25129=ORIENTED_EDGE ( 'NONE', *, *, #13849, .T. ) ;
#25135=AXIS2_PLACEMENT_3D ( 'NONE', #10316, #22967, #1552 ) ;
#25143=DIRECTION ( 'NONE',  ( 1.000000000000000000, 0.000000000000000000, 0.000000000000000000 ) ) ;
#25144=AXIS2_PLACEMENT_3D ( 'NONE', #19515, #8599, #2829 ) ;
#25147=PLANE ( 'NONE',  #27614 ) ;
#25150=CARTESIAN_POINT ( 'NONE',  ( -192.3374199748951412, 101.4858760524708430, 32.80924214881481760 ) ) ;
#25154=CARTESIAN_POINT ( 'NONE',  ( -237.6054256748464013, 69.18099216265957807, 14.87827728787644155 ) ) ;
#25164=DIRECTION ( 'NONE',  ( 1.000000000000000000, 0.000000000000000000, 0.000000000000000000 ) ) ;
#25167=CIRCLE ( 'NONE', #12795, 30.00000000000000000 ) ;
#25173=AXIS2_PLACEMENT_3D ( 'NONE', #2488, #644, #18022 ) ;
#25178=CARTESIAN_POINT ( 'NONE',  ( -42.53273978471831640, 130.9733465240572627, -14.93735646117641025 ) ) ;
#25180=CIRCLE ( 'NONE', #2248, 41.00000000000000711 ) ;
#25185=CARTESIAN_POINT ( 'NONE',  ( -228.3260857049913000, 133.0445111367240827, 15.00000000000000000 ) ) ;
#25187=ORIENTED_EDGE ( 'NONE', *, *, #18218, .T. ) ;
#25196=VECTOR ( 'NONE', #3187, 1000.000000000000000 ) ;
#25197=DIRECTION ( 'NONE',  ( -0.000000000000000000, 0.000000000000000000, 1.000000000000000000 ) ) ;
#25198=EDGE_LOOP ( 'NONE', ( #24429, #16977, #19143, #13592, #16459, #24285 ) ) ;
#25200=CARTESIAN_POINT ( 'NONE',  ( -133.3218633279795995, 128.8707778179846741, 17.13879255355997699 ) ) ;
#25205=CARTESIAN_POINT ( 'NONE',  ( -225.7036482868739427, -91.18033988749901653, 0.000000000000000000 ) ) ;
#25211=ADVANCED_FACE ( 'NONE', ( #22911 ), #11200, .T. ) ;
#25212=VECTOR ( 'NONE', #28283, 1000.000000000000000 ) ;
#25213=CARTESIAN_POINT ( 'NONE',  ( 1.982541115402066017E-14, -150.0000000000000568, 100.0000000000000142 ) ) ;
#25215=DIRECTION ( 'NONE',  ( 1.000000000000000000, 0.000000000000000000, 0.000000000000000000 ) ) ;
#25218=CARTESIAN_POINT ( 'NONE',  ( -63.57415822541634043, -18.01420295945611727, 100.0000000000000000 ) ) ;
#25219=DIRECTION ( 'NONE',  ( -1.000000000000000000, 0.000000000000000000, 0.000000000000000000 ) ) ;
#25220=DIRECTION ( 'NONE',  ( -0.8498245983675984938, -0.3891357156574838383, -0.3554877590144110422 ) ) ;
#25223=CARTESIAN_POINT ( 'NONE',  ( 113.6021183481336294, 213.0266806119306580, -97.68838206577098049 ) ) ;
#25226=CARTESIAN_POINT ( 'NONE',  ( -7.377946765535823737, 132.9103126869670461, 14.28005041300768951 ) ) ;
#25229=FACE_OUTER_BOUND ( 'NONE', #24183, .T. ) ;
#25235=CARTESIAN_POINT ( 'NONE',  ( 51.56615429303207065, 203.2034914284457159, -13.00000000000000000 ) ) ;
#25242=ADVANCED_FACE ( 'NONE', ( #4910 ), #4770, .F. ) ;
#25245=FACE_OUTER_BOUND ( 'NONE', #16110, .T. ) ;
#25248=EDGE_CURVE ( 'NONE', #8411, #5833, #22308, .T. ) ;
#25250=CARTESIAN_POINT ( 'NONE',  ( -96.46213353889478981, 134.5400755604871392, -15.50096989933989278 ) ) ;
#25251=CARTESIAN_POINT ( 'NONE',  ( -208.1368626653883780, 75.14204529818155720, 39.73078884062161364 ) ) ;
#25252=DIRECTION ( 'NONE',  ( 1.000000000000000000, -0.000000000000000000, -0.000000000000000000 ) ) ;
#25253=CARTESIAN_POINT ( 'NONE',  ( -137.5457983441765464, 129.0117491753162255, -15.70601345937086535 ) ) ;
#25255=DIRECTION ( 'NONE',  ( 1.000000000000000000, 0.000000000000000000, 0.000000000000000000 ) ) ;
#25256=CARTESIAN_POINT ( 'NONE',  ( -203.7987795937083888, 92.08070442507484188, 29.54447684135760355 ) ) ;
#25257=CARTESIAN_POINT ( 'NONE',  ( -235.6837214056122036, 120.7228219557777180, -15.00000000000000000 ) ) ;
#25269=ORIENTED_EDGE ( 'NONE', *, *, #17067, .T. ) ;
#25276=DIRECTION ( 'NONE',  ( -0.000000000000000000, 1.000000000000000000, -1.387778780781445429E-16 ) ) ;
#25278=EDGE_CURVE ( 'NONE', #13809, #4321, #4385, .T. ) ;
#25280=CARTESIAN_POINT ( 'NONE',  ( 107.0237911392832189, 245.0638502168177979, -31.95161221448068645 ) ) ;
#25284=CARTESIAN_POINT ( 'NONE',  ( -190.0000000000000284, 59.99999999999995026, 98.28427124746191623 ) ) ;
#25285=CARTESIAN_POINT ( 'NONE',  ( -220.8087078309937397, 71.35508338393960059, -21.10002476983576969 ) ) ;
#25286=AXIS2_PLACEMENT_3D ( 'NONE', #1785, #25503, #10562 ) ;
#25289=CYLINDRICAL_SURFACE ( 'NONE', #15677, 30.00000000000000000 ) ;
#25296=VERTEX_POINT ( 'NONE', #3040 ) ;
#25301=CARTESIAN_POINT ( 'NONE',  ( 89.77759941121971110, 81.13568025368125802, 100.0000000000000142 ) ) ;
#25305=CARTESIAN_POINT ( 'NONE',  ( 81.45493510941093973, 110.0000000000000142, -70.00000000034538061 ) ) ;
#25308=DIRECTION ( 'NONE',  ( -0.000000000000000000, -0.000000000000000000, -1.000000000000000000 ) ) ;
#25310=CARTESIAN_POINT ( 'NONE',  ( -228.3964932543056250, 90.87356368223484537, 15.41412920056914260 ) ) ;
#25311=VERTEX_POINT ( 'NONE', #622 ) ;
#25316=EDGE_CURVE ( 'NONE', #23965, #16453, #8990, .T. ) ;
#25317=ADVANCED_FACE ( 'NONE', ( #760 ), #24313, .F. ) ;
#25319=LINE ( 'NONE', #20448, #19465 ) ;
#25321=DIRECTION ( 'NONE',  ( 1.000000000000000000, 4.625929269271485914E-16, 0.000000000000000000 ) ) ;
#25322=CARTESIAN_POINT ( 'NONE',  ( -231.9378824387731299, 93.53122965655670384, 12.99999999999999822 ) ) ;
#25323=CARTESIAN_POINT ( 'NONE',  ( -180.4068668408075666, 109.4706979435998306, -30.97813022004903516 ) ) ;
#25332=ORIENTED_EDGE ( 'NONE', *, *, #21905, .T. ) ;
#25334=TOROIDAL_SURFACE ( 'NONE', #1030, 60.00000000000000000, 30.00000000000000000 ) ;
#25335=DIRECTION ( 'NONE',  ( -0.000000000000000000, 1.000000000000000000, -1.387778780781445429E-16 ) ) ;
#25338=ORIENTED_EDGE ( 'NONE', *, *, #23982, .F. ) ;
#25353=DIRECTION ( 'NONE',  ( 0.000000000000000000, 0.000000000000000000, 1.000000000000000000 ) ) ;
#25359=AXIS2_PLACEMENT_3D ( 'NONE', #14382, #9926, #25143 ) ;
#25362=DIRECTION ( 'NONE',  ( 0.9960550913260672878, 1.086714821493793968E-17, 0.08873699929240064233 ) ) ;
#25367=DIRECTION ( 'NONE',  ( -2.139922160430261846E-32, 1.387778780781445429E-16, 1.000000000000000000 ) ) ;
#25370=CARTESIAN_POINT ( 'NONE',  ( 109.9999999999999005, 260.0000000000000000, -45.00000000000000000 ) ) ;
#25371=CARTESIAN_POINT ( 'NONE',  ( 24.59638288546416973, 86.21496700725640494, 99.35042210466092172 ) ) ;
#25373=DIRECTION ( 'NONE',  ( -1.000000000000000000, -2.312964634635742957E-16, 0.000000000000000000 ) ) ;
#25376=VECTOR ( 'NONE', #18709, 1000.000000000000000 ) ;
#25377=EDGE_CURVE ( 'NONE', #12779, #7297, #8520, .T. ) ;
#25378=AXIS2_PLACEMENT_3D ( 'NONE', #5512, #25335, #9831 ) ;
#25381=DIRECTION ( 'NONE',  ( 0.000000000000000000, 0.000000000000000000, -1.000000000000000000 ) ) ;
#25382=ORIENTED_EDGE ( 'NONE', *, *, #2793, .T. ) ;
#25388=DIRECTION ( 'NONE',  ( -0.000000000000000000, 1.000000000000000000, -1.387778780781445429E-16 ) ) ;
#25392=TOROIDAL_SURFACE ( 'NONE', #17596, 11.00000000000001066, 1.000000000000000000 ) ;
#25393=CARTESIAN_POINT ( 'NONE',  ( -208.8418814728804023, 74.65865074066952900, 37.27912060900214186 ) ) ;
#25395=CARTESIAN_POINT ( 'NONE',  ( -152.9354250843960585, 123.6290117556221162, -18.69239437641641999 ) ) ;
#25398=LINE ( 'NONE', #10034, #25940 ) ;
#25404=CARTESIAN_POINT ( 'NONE',  ( -175.0000000000000000, -120.0250000000001904, -69.99999999999998579 ) ) ;
#25405=CARTESIAN_POINT ( 'NONE',  ( -203.2481855153402250, 92.57460631283319685, 29.78692811926998729 ) ) ;
#25406=EDGE_CURVE ( 'NONE', #606, #18799, #28225, .T. ) ;
#25407=ORIENTED_EDGE ( 'NONE', *, *, #206, .F. ) ;
#25416=VERTEX_POINT ( 'NONE', #18560 ) ;
#25421=FACE_BOUND ( 'NONE', #9238, .T. ) ;
#25422=CARTESIAN_POINT ( 'NONE',  ( 108.4328758917250468, 248.8772442435372056, -35.32571066851171082 ) ) ;
#25423=CARTESIAN_POINT ( 'NONE',  ( 5.538391900817774882, 137.3871724827027947, -15.09218160842566370 ) ) ;
#25428=EDGE_CURVE ( 'NONE', #15348, #3825, #23292, .T. ) ;
#25429=CARTESIAN_POINT ( 'NONE',  ( 179.9999999999999147, -150.0000000000000284, 100.0000000000000142 ) ) ;
#25430=CARTESIAN_POINT ( 'NONE',  ( 3.469446951953617344E-15, -40.00000000000003553, -70.00000000000001421 ) ) ;
#25431=FACE_OUTER_BOUND ( 'NONE', #17142, .T. ) ;
#25435=CARTESIAN_POINT ( 'NONE',  ( -195.0245959749996132, 99.69668914553523109, 31.69045126054473371 ) ) ;
#25438=CARTESIAN_POINT ( 'NONE',  ( -12.24491960465745599, -23.01420295945612082, 80.00000000000001421 ) ) ;
#25442=CARTESIAN_POINT ( 'NONE',  ( 84.91648909974954051, 110.3843228243387102, 100.0000000000000142 ) ) ;
#25445=CIRCLE ( 'NONE', #13085, 5.000000000000004441 ) ;
#25446=VERTEX_POINT ( 'NONE', #16829 ) ;
#25448=B_SPLINE_CURVE_WITH_KNOTS ( 'NONE', 3,
 ( #8490, #8918, #12952, #8634, #17389, #2156, #26003, #26425, #4167 ),
 .UNSPECIFIED., .F., .F.,
 ( 4, 2, 1, 2, 4 ),
 ( 0.000000000000000000, 0.003850132855190854363, 0.007700265710381708727, 0.01155039856557256266, 0.01540053142076341745 ),
 .UNSPECIFIED. ) ;
#25450=CARTESIAN_POINT ( 'NONE',  ( -42.53273978471831640, 130.9733465240572627, -15.00000000000000000 ) ) ;
#25459=CARTESIAN_POINT ( 'NONE',  ( 79.99999999999992895, 110.0000000000000000, -45.00000000000000000 ) ) ;
#25469=ORIENTED_EDGE ( 'NONE', *, *, #27074, .T. ) ;
#25471=CARTESIAN_POINT ( 'NONE',  ( 109.9999999999999005, 3.816391647148972452E-14, -70.00000000000001421 ) ) ;
#25474=CYLINDRICAL_SURFACE ( 'NONE', #1969, 58.90601976618767566 ) ;
#25475=DIRECTION ( 'NONE',  ( 0.000000000000000000, 0.000000000000000000, -1.000000000000000000 ) ) ;
#25480=VECTOR ( 'NONE', #19114, 1000.000000000000000 ) ;
#25481=ORIENTED_EDGE ( 'NONE', *, *, #23327, .T. ) ;
#25483=CARTESIAN_POINT ( 'NONE',  ( 134.9999999999998579, 220.0000000000000284, -90.00000000000002842 ) ) ;
#25485=ORIENTED_EDGE ( 'NONE', *, *, #15793, .F. ) ;
#25488=VERTEX_POINT ( 'NONE', #27174 ) ;
#25490=ORIENTED_EDGE ( 'NONE', *, *, #27975, .F. ) ;
#25495=CARTESIAN_POINT ( 'NONE',  ( 9.999999999999738876, -50.00000000000004263, 110.0000000000000284 ) ) ;
#25496=CARTESIAN_POINT ( 'NONE',  ( -225.9729034214362571, 132.4331356209112300, 12.99353264133693919 ) ) ;
#25497=LINE ( 'NONE', #5814, #22495 ) ;
#25499=PLANE ( 'NONE',  #5760 ) ;
#25500=EDGE_CURVE ( 'NONE', #20823, #16820, #8491, .T. ) ;
#25501=CARTESIAN_POINT ( 'NONE',  ( -221.7690971916800322, 71.47334710437645811, -20.39711061091116662 ) ) ;
#25503=DIRECTION ( 'NONE',  ( -0.000000000000000000, -0.000000000000000000, 1.000000000000000000 ) ) ;
#25506=EDGE_LOOP ( 'NONE', ( #19973, #16739, #24158, #12607 ) ) ;
#25511=CYLINDRICAL_SURFACE ( 'NONE', #1015, 30.00000000000000000 ) ;
#25512=ORIENTED_EDGE ( 'NONE', *, *, #8204, .T. ) ;
#25513=VECTOR ( 'NONE', #12814, 1000.000000000000000 ) ;
#25516=CARTESIAN_POINT ( 'NONE',  ( -232.2365570322886299, 76.71063732366134502, 15.57345046155156432 ) ) ;
#25517=ORIENTED_EDGE ( 'NONE', *, *, #7986, .F. ) ;
#25521=CARTESIAN_POINT ( 'NONE',  ( -47.46858701631881416, 132.2250854490906420, 14.48589841498654174 ) ) ;
#25524=CARTESIAN_POINT ( 'NONE',  ( 112.8630565061745017, 215.9427151076712619, 97.00605251950267416 ) ) ;
#25525=EDGE_CURVE ( 'NONE', #1333, #13440, #3955, .T. ) ;
#25528=CARTESIAN_POINT ( 'NONE',  ( -152.6794942072440904, 123.7315770332490956, -19.76807053014819004 ) ) ;
#25530=DIRECTION ( 'NONE',  ( 1.000000000000000000, 0.000000000000000000, 0.000000000000000000 ) ) ;
#25531=DIRECTION ( 'NONE',  ( 0.000000000000000000, -0.000000000000000000, 1.000000000000000000 ) ) ;
#25532=DIRECTION ( 'NONE',  ( 0.7082136108520787898, 0.7059982162894324897, -0.000000000000000000 ) ) ;
#25534=CARTESIAN_POINT ( 'NONE',  ( -143.6428522700808230, 20.24192588826928585, 83.00000000000001421 ) ) ;
#25535=EDGE_CURVE ( 'NONE', #25488, #6227, #6325, .T. ) ;
#25537=LINE ( 'NONE', #3694, #19644 ) ;
#25539=ORIENTED_EDGE ( 'NONE', *, *, #6193, .F. ) ;
#25540=CARTESIAN_POINT ( 'NONE',  ( 93.99999999999985789, 171.5103103742661972, -105.0000000000000284 ) ) ;
#25545=VERTEX_POINT ( 'NONE', #14826 ) ;
#25548=ORIENTED_EDGE ( 'NONE', *, *, #18706, .T. ) ;
#25551=DIRECTION ( 'NONE',  ( -0.6782242722910949428, -0.7348549764921067373, 0.000000000000000000 ) ) ;
#25552=DIRECTION ( 'NONE',  ( -0.000000000000000000, -1.000000000000000000, -0.000000000000000000 ) ) ;
#25554=CARTESIAN_POINT ( 'NONE',  ( 109.9984815155424656, 259.5975204907896909, -44.65144252145412906 ) ) ;
#25558=DIRECTION ( 'NONE',  ( 0.000000000000000000, 0.000000000000000000, -1.000000000000000000 ) ) ;
#25560=CARTESIAN_POINT ( 'NONE',  ( -207.5044420441007276, 75.59897387903043864, -45.00000000000000000 ) ) ;
#25563=CARTESIAN_POINT ( 'NONE',  ( -76.25760768171836901, 154.8982798170083299, 15.00000000000000000 ) ) ;
#25565=CARTESIAN_POINT ( 'NONE',  ( -237.3870311360069536, 121.7710280244218950, 13.00000000000000000 ) ) ;
#25571=ORIENTED_EDGE ( 'NONE', *, *, #2049, .F. ) ;
#25574=EDGE_CURVE ( 'NONE', #24468, #16686, #21851, .T. ) ;
#25578=DIRECTION ( 'NONE',  ( 1.321694076934710155E-16, -1.000000000000000000, 0.000000000000000000 ) ) ;
#25579=CARTESIAN_POINT ( 'NONE',  ( 109.2201559107103037, 251.9988677676353177, 38.05717760203712174 ) ) ;
#25584=EDGE_LOOP ( 'NONE', ( #14435, #4170, #27547, #1699 ) ) ;
#25585=CARTESIAN_POINT ( 'NONE',  ( 134.9999999999998579, 220.0000000000000284, -99.00000000000001421 ) ) ;
#25587=EDGE_CURVE ( 'NONE', #27002, #2675, #17262, .T. ) ;
#25588=CARTESIAN_POINT ( 'NONE',  ( 33.10302365956999182, 203.2034914284457159, -15.00000000000000000 ) ) ;
#25592=CARTESIAN_POINT ( 'NONE',  ( 0.000000000000000000, 0.000000000000000000, -100.0000000000000142 ) ) ;
#25594=CONICAL_SURFACE ( 'NONE', #16008, 6.025000000000002132, 0.7853981633974482790 ) ;
#25598=CARTESIAN_POINT ( 'NONE',  ( 65.00000000000000000, -120.0000000000000995, -64.00000000000000000 ) ) ;
#25610=DIRECTION ( 'NONE',  ( 1.000000000000000000, 8.542487643439285958E-16, 0.000000000000000000 ) ) ;
#25612=CARTESIAN_POINT ( 'NONE',  ( -148.7496381368905247, 124.1794587942970907, 19.49431050908225060 ) ) ;
#25625=ORIENTED_EDGE ( 'NONE', *, *, #13050, .T. ) ;
#25633=DIRECTION ( 'NONE',  ( -1.850371707708594316E-16, 1.000000000000000000, -0.000000000000000000 ) ) ;
#25634=CARTESIAN_POINT ( 'NONE',  ( -230.0306293838648912, 64.31401865984727806, -16.82661551914406317 ) ) ;
#25640=EDGE_LOOP ( 'NONE', ( #8603, #6668 ) ) ;
#25642=AXIS2_PLACEMENT_3D ( 'NONE', #3945, #6246, #6106 ) ;
#25654=CARTESIAN_POINT ( 'NONE',  ( -43.02437977270768243, 129.7200458115292747, 16.81627168235289460 ) ) ;
#25657=VECTOR ( 'NONE', #6837, 1000.000000000000000 ) ;
#25660=ORIENTED_EDGE ( 'NONE', *, *, #757, .F. ) ;
#25662=CARTESIAN_POINT ( 'NONE',  ( -190.0000000000000284, 59.99999999999995026, 80.00000000000001421 ) ) ;
#25663=DIRECTION ( 'NONE',  ( 0.000000000000000000, 0.000000000000000000, -1.000000000000000000 ) ) ;
#25664=CIRCLE ( 'NONE', #5463, 70.83858790703926900 ) ;
#25665=CARTESIAN_POINT ( 'NONE',  ( -148.0316173832768527, 125.5119630376401432, -18.70358149194362340 ) ) ;
#25670=CARTESIAN_POINT ( 'NONE',  ( -218.1021218244185604, 87.79535473091540609, -19.36533790319589698 ) ) ;
#25672=EDGE_CURVE ( 'NONE', #24608, #11100, #2439, .T. ) ;
#25683=ORIENTED_EDGE ( 'NONE', *, *, #13685, .F. ) ;
#25686=CIRCLE ( 'NONE', #7789, 1.999999999999997335 ) ;
#25687=ADVANCED_FACE ( 'NONE', ( #6900 ), #15064, .T. ) ;
#25688=CARTESIAN_POINT ( 'NONE',  ( 96.03789414441068573, 240.4739163874471330, -19.46186845665527443 ) ) ;
#25690=ORIENTED_EDGE ( 'NONE', *, *, #11146, .T. ) ;
#25691=ORIENTED_EDGE ( 'NONE', *, *, #5004, .F. ) ;
#25698=CARTESIAN_POINT ( 'NONE',  ( -141.6428522700808230, 22.24192588826928585, 83.00000000000001421 ) ) ;
#25699=PLANE ( 'NONE',  #27670 ) ;
#25705=CARTESIAN_POINT ( 'NONE',  ( -194.4086842179900714, 63.14614340836796913, -41.97977085781615614 ) ) ;
#25707=CARTESIAN_POINT ( 'NONE',  ( 184.9999999999999432, -327.2004514666934369, -84.99999999999997158 ) ) ;
#25711=CARTESIAN_POINT ( 'NONE',  ( 115.9304285313508700, 231.9550723406498776, -99.14012769162694383 ) ) ;
#25713=DIRECTION ( 'NONE',  ( 1.000000000000000000, 0.000000000000000000, 0.000000000000000000 ) ) ;
#25714=ORIENTED_EDGE ( 'NONE', *, *, #14198, .T. ) ;
#25716=EDGE_CURVE ( 'NONE', #1393, #20275, #13618, .T. ) ;
#25717=ORIENTED_EDGE ( 'NONE', *, *, #5673, .F. ) ;
#25724=ORIENTED_EDGE ( 'NONE', *, *, #6008, .F. ) ;
#25726=CARTESIAN_POINT ( 'NONE',  ( 106.6902265666634122, 244.3124981716793513, 31.28096500751039599 ) ) ;
#25729=DIRECTION ( 'NONE',  ( 1.000000000000000000, 0.000000000000000000, 0.000000000000000000 ) ) ;
#25739=CARTESIAN_POINT ( 'NONE',  ( 119.9999999999999147, 140.0000000000000000, 100.0000000000000142 ) ) ;
#25744=CARTESIAN_POINT ( 'NONE',  ( 116.2340178909017396, 232.4263996303828606, 99.27034901580076109 ) ) ;
#25747=CARTESIAN_POINT ( 'NONE',  ( -225.7485474213321481, 89.51658778958633889, 13.99034047932378755 ) ) ;
#25753=EDGE_CURVE ( 'NONE', #11803, #1940, #17606, .T. ) ;
#25756=ADVANCED_FACE ( 'NONE', ( #2508, #17318 ), #6689, .F. ) ;
#25764=AXIS2_PLACEMENT_3D ( 'NONE', #10892, #20213, #24379 ) ;
#25773=CARTESIAN_POINT ( 'NONE',  ( -236.8177751472017007, 82.33896643611701904, -15.00000000000000178 ) ) ;
#25778=CARTESIAN_POINT ( 'NONE',  ( -175.0000000000000000, -120.0000000000001847, -69.99999999999998579 ) ) ;
#25779=CARTESIAN_POINT ( 'NONE',  ( 112.5712424644275131, 222.0554180856713060, -96.69730840357117074 ) ) ;
#25788=CARTESIAN_POINT ( 'NONE',  ( -63.57415822541634043, 0.000000000000000000, 95.00000000000000000 ) ) ;
#25796=LINE ( 'NONE', #23648, #22278 ) ;
#25799=EDGE_LOOP ( 'NONE', ( #21629, #6198, #9965, #8638 ) ) ;
#25800=CARTESIAN_POINT ( 'NONE',  ( -75.20817585874782196, 134.4830317599007685, 15.51105434715999465 ) ) ;
#25802=ORIENTED_EDGE ( 'NONE', *, *, #1564, .F. ) ;
#25805=CARTESIAN_POINT ( 'NONE',  ( -134.4422573331441697, 128.5907357665044799, -17.24671386403461071 ) ) ;
#25808=CARTESIAN_POINT ( 'NONE',  ( -112.7304692548805605, 133.0259997015394333, -15.80934902741073067 ) ) ;
#25810=CARTESIAN_POINT ( 'NONE',  ( -160.0000000000000284, 139.9999999999999716, 45.00000000000000000 ) ) ;
#25812=CARTESIAN_POINT ( 'NONE',  ( -220.0227340339567661, 87.95399931298469198, -18.35314071734302388 ) ) ;
#25813=CARTESIAN_POINT ( 'NONE',  ( -146.6428522700808230, 17.24192588826928585, 83.00000000000001421 ) ) ;
#25815=EDGE_CURVE ( 'NONE', #18495, #14427, #14070, .T. ) ;
#25817=DIRECTION ( 'NONE',  ( 0.000000000000000000, 0.000000000000000000, -1.000000000000000000 ) ) ;
#25820=VECTOR ( 'NONE', #20010, 1000.000000000000000 ) ;
#25825=DIRECTION ( 'NONE',  ( -0.000000000000000000, -0.000000000000000000, 1.000000000000000000 ) ) ;
#25826=CIRCLE ( 'NONE', #28089, 30.00000000000000000 ) ;
#25830=CARTESIAN_POINT ( 'NONE',  ( 95.18208312637753465, 240.6790578601106745, -9.159889466453034146 ) ) ;
#25836=ORIENTED_EDGE ( 'NONE', *, *, #25278, .F. ) ;
#25838=DIRECTION ( 'NONE',  ( 1.000000000000000000, 0.000000000000000000, 0.000000000000000000 ) ) ;
#25840=FACE_OUTER_BOUND ( 'NONE', #20079, .T. ) ;
#25841=VECTOR ( 'NONE', #7840, 1000.000000000000000 ) ;
#25842=CARTESIAN_POINT ( 'NONE',  ( 109.9999999999999005, 259.7997850037947956, -44.82660872220826320 ) ) ;
#25844=FACE_OUTER_BOUND ( 'NONE', #13288, .T. ) ;
#25847=DIRECTION ( 'NONE',  ( 1.000000000000000000, 0.000000000000000000, 0.000000000000000000 ) ) ;
#25848=EDGE_CURVE ( 'NONE', #20650, #23124, #20009, .T. ) ;
#25849=CARTESIAN_POINT ( 'NONE',  ( -42.65532241761712839, 131.0044336801082352, 16.34779397420836844 ) ) ;
#25851=CARTESIAN_POINT ( 'NONE',  ( -200.0000000000000284, -120.0000000000001847, 25.00000000000001776 ) ) ;
#25852=CARTESIAN_POINT ( 'NONE',  ( -68.57415822541635464, -23.01420295945612082, 100.0000000000000000 ) ) ;
#25853=ORIENTED_EDGE ( 'NONE', *, *, #21678, .F. ) ;
#25854=CIRCLE ( 'NONE', #17146, 16.46313063346208239 ) ;
#25855=CARTESIAN_POINT ( 'NONE',  ( -174.8584600856924283, 112.6472680211073936, 28.91287214637171132 ) ) ;
#25857=DIRECTION ( 'NONE',  ( -0.000000000000000000, -0.000000000000000000, -1.000000000000000000 ) ) ;
#25861=ORIENTED_EDGE ( 'NONE', *, *, #15371, .T. ) ;
#25862=EDGE_LOOP ( 'NONE', ( #6905, #3769, #17316, #26329, #1000, #6000 ) ) ;
#25863=EDGE_CURVE ( 'NONE', #23690, #19503, #8570, .T. ) ;
#25865=CARTESIAN_POINT ( 'NONE',  ( 119.7545560453059892, 132.4900181921427702, 100.0000000000000142 ) ) ;
#25867=ORIENTED_EDGE ( 'NONE', *, *, #8389, .F. ) ;
#25869=CARTESIAN_POINT ( 'NONE',  ( 107.3061218092339715, 127.3934823308176760, -87.81249999970602005 ) ) ;
#25870=CARTESIAN_POINT ( 'NONE',  ( 100.0424040729205188, 235.0879316926391596, 22.67296783064056243 ) ) ;
#25871=CARTESIAN_POINT ( 'NONE',  ( -180.0000000000000284, 59.99999999999994316, -70.00000000000001421 ) ) ;
#25872=ORIENTED_EDGE ( 'NONE', *, *, #7432, .F. ) ;
#25873=CARTESIAN_POINT ( 'NONE',  ( -207.2993993385316855, 89.56313076513357885, 27.29723889156834105 ) ) ;
#25875=CIRCLE ( 'NONE', #15819, 2.000000000000004885 ) ;
#25878=CARTESIAN_POINT ( 'NONE',  ( -63.57415822541634043, 75.97823757117562593, 95.00000000000000000 ) ) ;
#25880=FACE_OUTER_BOUND ( 'NONE', #13720, .T. ) ;
#25885=DIRECTION ( 'NONE',  ( 0.000000000000000000, 0.000000000000000000, 1.000000000000000000 ) ) ;
#25887=CARTESIAN_POINT ( 'NONE',  ( -270.1025481742786951, -91.18033988749901653, -11.42311362948588105 ) ) ;
#25890=VERTEX_POINT ( 'NONE', #1944 ) ;
#25892=CARTESIAN_POINT ( 'NONE',  ( -192.4016700810780094, 101.6532444370910468, 31.99634417553368948 ) ) ;
#25894=DIRECTION ( 'NONE',  ( 0.000000000000000000, 0.000000000000000000, 1.000000000000000000 ) ) ;
#25895=EDGE_LOOP ( 'NONE', ( #22181, #6643, #24344, #1281 ) ) ;
#25898=AXIS2_PLACEMENT_3D ( 'NONE', #12973, #10805, #23730 ) ;
#25899=CARTESIAN_POINT ( 'NONE',  ( -151.0494637935773881, 123.3493803929174391, 20.02198554298006528 ) ) ;
#25900=CARTESIAN_POINT ( 'NONE',  ( -184.1540942457759229, 107.3771663064187152, -31.09098462597617996 ) ) ;
#25901=VERTEX_POINT ( 'NONE', #11733 ) ;
#25902=EDGE_CURVE ( 'NONE', #27860, #25890, #23692, .T. ) ;
#25905=ORIENTED_EDGE ( 'NONE', *, *, #12455, .T. ) ;
#25909=FACE_OUTER_BOUND ( 'NONE', #26802, .T. ) ;
#25910=VECTOR ( 'NONE', #944, 1000.000000000000000 ) ;
#25912=DIRECTION ( 'NONE',  ( -0.000000000000000000, -0.000000000000000000, -1.000000000000000000 ) ) ;
#25913=AXIS2_PLACEMENT_3D ( 'NONE', #8043, #23700, #18817 ) ;
#25918=CARTESIAN_POINT ( 'NONE',  ( -230.6867234551526167, 75.40543009380724016, -15.98884730489883665 ) ) ;
#25920=CARTESIAN_POINT ( 'NONE',  ( 46.79174272583949090, 194.0572550123460474, -15.00000000000000000 ) ) ;
#25921=CIRCLE ( 'NONE', #13557, 5.000000000000004441 ) ;
#25937=ORIENTED_EDGE ( 'NONE', *, *, #24249, .F. ) ;
#25938=VECTOR ( 'NONE', #8541, 1000.000000000000000 ) ;
#25940=VECTOR ( 'NONE', #3840, 1000.000000000000000 ) ;
#25941=ORIENTED_EDGE ( 'NONE', *, *, #27975, .T. ) ;
#25943=ORIENTED_EDGE ( 'NONE', *, *, #19925, .T. ) ;
#25947=ORIENTED_EDGE ( 'NONE', *, *, #28012, .T. ) ;
#25948=LINE ( 'NONE', #6267, #5393 ) ;
#25949=CARTESIAN_POINT ( 'NONE',  ( -62.68650544878820341, 133.3634780166508165, -15.73273055292821354 ) ) ;
#25951=CARTESIAN_POINT ( 'NONE',  ( -156.3896018538470116, 122.2161512765613480, -19.69795454272433233 ) ) ;
#25956=CARTESIAN_POINT ( 'NONE',  ( -228.4262338387342197, 88.49915910525061236, -15.54344599199708910 ) ) ;
#25959=CIRCLE ( 'NONE', #15412, 18.46313063346208239 ) ;
#25961=DIRECTION ( 'NONE',  ( 1.000000000000000000, -0.000000000000000000, -0.000000000000000000 ) ) ;
#25970=EDGE_LOOP ( 'NONE', ( #1054, #26605, #26752, #24753, #10403, #2391, #786, #8032 ) ) ;
#25971=VERTEX_POINT ( 'NONE', #20476 ) ;
#25972=CARTESIAN_POINT ( 'NONE',  ( 91.79864198314089663, 239.6982472080514128, -17.32810371388483262 ) ) ;
#25973=ORIENTED_EDGE ( 'NONE', *, *, #2567, .F. ) ;
#25984=DIRECTION ( 'NONE',  ( 0.000000000000000000, 0.000000000000000000, -1.000000000000000000 ) ) ;
#25989=DIRECTION ( 'NONE',  ( -1.000000000000000000, -1.530283246943720875E-16, 0.000000000000000000 ) ) ;
#25991=CARTESIAN_POINT ( 'NONE',  ( -24.64763201754189481, 128.0468424616478273, 17.48411470635667797 ) ) ;
#25992=CARTESIAN_POINT ( 'NONE',  ( -209.9392250573528429, 62.66900426808626179, 27.74467448083618493 ) ) ;
#25994=DIRECTION ( 'NONE',  ( 1.000000000000000000, 0.000000000000000000, 0.000000000000000000 ) ) ;
#25995=VERTEX_POINT ( 'NONE', #9704 ) ;
#25997=CARTESIAN_POINT ( 'NONE',  ( -188.6435715486210540, 104.1343366490829823, 32.77691502914932897 ) ) ;
#26001=EDGE_CURVE ( 'NONE', #24382, #8538, #24648, .T. ) ;
#26002=EDGE_LOOP ( 'NONE', ( #3897, #1112 ) ) ;
#26003=CARTESIAN_POINT ( 'NONE',  ( -217.7401460507883826, 138.5677444271665877, -12.99353264133693919 ) ) ;
#26007=CARTESIAN_POINT ( 'NONE',  ( 108.2273028572353297, 129.5338070842080924, -88.59375000024363089 ) ) ;
#26012=CARTESIAN_POINT ( 'NONE',  ( -222.3308448878950401, 86.50594421447330262, 17.61308416972892132 ) ) ;
#26019=LINE ( 'NONE', #425, #1419 ) ;
#26020=ORIENTED_EDGE ( 'NONE', *, *, #13685, .T. ) ;
#26029=AXIS2_PLACEMENT_3D ( 'NONE', #25011, #4892, #22853 ) ;
#26037=AXIS2_PLACEMENT_3D ( 'NONE', #11188, #26397, #6724 ) ;
#26039=EDGE_CURVE ( 'NONE', #2675, #5984, #22349, .T. ) ;
#26041=CARTESIAN_POINT ( 'NONE',  ( -167.8789958130436162, 116.8334710968284327, -25.29509310206942985 ) ) ;
#26044=CARTESIAN_POINT ( 'NONE',  ( -112.9862511722770790, 70.97208026367574973, 82.84066614128462902 ) ) ;
#26050=DIRECTION ( 'NONE',  ( 0.000000000000000000, 0.000000000000000000, -1.000000000000000000 ) ) ;
#26051=TOROIDAL_SURFACE ( 'NONE', #1285, 68.83858790703926900, 2.000000000000000000 ) ;
#26054=DIRECTION ( 'NONE',  ( -1.000000000000000000, 0.000000000000000000, 0.000000000000000000 ) ) ;
#26057=LINE ( 'NONE', #8820, #14941 ) ;
#26058=CARTESIAN_POINT ( 'NONE',  ( -228.6046226639666088, 73.96500373646588855, -16.69423931604977085 ) ) ;
#26059=EDGE_LOOP ( 'NONE', ( #13745, #14362, #15071, #1693 ) ) ;
#26062=CARTESIAN_POINT ( 'NONE',  ( 156.4999999999998579, 220.0000000000000284, 100.0000000000000142 ) ) ;
#26063=CARTESIAN_POINT ( 'NONE',  ( 113.4521041897134097, 213.5046054548297434, -97.56026172913361449 ) ) ;
#26065=CARTESIAN_POINT ( 'NONE',  ( -226.5998460896583993, 62.96930358458836707, 8.263950894743116393 ) ) ;
#26066=AXIS2_PLACEMENT_3D ( 'NONE', #7714, #14323, #5695 ) ;
#26068=DIRECTION ( 'NONE',  ( 0.000000000000000000, -0.000000000000000000, -1.000000000000000000 ) ) ;
#26071=CARTESIAN_POINT ( 'NONE',  ( 134.9999999999998579, 220.0000000000000284, 100.0000000000000142 ) ) ;
#26073=CARTESIAN_POINT ( 'NONE',  ( -231.4586860447602703, 76.02675087360279349, 15.76935333479230117 ) ) ;
#26074=ORIENTED_EDGE ( 'NONE', *, *, #8028, .F. ) ;
#26080=CARTESIAN_POINT ( 'NONE',  ( -200.0000000000000284, 0.000000000000000000, 25.00000000000000000 ) ) ;
#26082=ORIENTED_EDGE ( 'NONE', *, *, #17635, .T. ) ;
#26083=CARTESIAN_POINT ( 'NONE',  ( -224.3418196798764086, 136.6081117166938839, 14.97424725141357271 ) ) ;
#26088=CARTESIAN_POINT ( 'NONE',  ( -12.24491960465745599, 29.64876300893806516, 95.00000000000000000 ) ) ;
#26092=LINE ( 'NONE', #13326, #8067 ) ;
#26093=VECTOR ( 'NONE', #14277, 1000.000000000000000 ) ;
#26096=CARTESIAN_POINT ( 'NONE',  ( 109.9999999999999147, 140.0000000000000000, -90.00000000000004263 ) ) ;
#26097=DIRECTION ( 'NONE',  ( 0.8018642810807398158, 0.5975062131282554700, 0.000000000000000000 ) ) ;
#26103=DIRECTION ( 'NONE',  ( 1.000000000000000000, 0.000000000000000000, 0.000000000000000000 ) ) ;
#26106=CIRCLE ( 'NONE', #23824, 1.000000000000000888 ) ;
#26107=CARTESIAN_POINT ( 'NONE',  ( 88.62124187923063801, 239.8086506234227784, -16.24979138472547291 ) ) ;
#26108=ORIENTED_EDGE ( 'NONE', *, *, #6149, .F. ) ;
#26109=ORIENTED_EDGE ( 'NONE', *, *, #830, .F. ) ;
#26110=CIRCLE ( 'NONE', #20104, 22.49999999999999289 ) ;
#26112=VERTEX_POINT ( 'NONE', #3505 ) ;
#26116=ADVANCED_FACE ( 'NONE', ( #3647 ), #19110, .T. ) ;
#26117=ORIENTED_EDGE ( 'NONE', *, *, #25535, .F. ) ;
#26118=VERTEX_POINT ( 'NONE', #3364 ) ;
#26119=VERTEX_POINT ( 'NONE', #1358 ) ;
#26120=DIRECTION ( 'NONE',  ( -1.000000000000000000, 0.000000000000000000, 0.000000000000000000 ) ) ;
#26122=FACE_OUTER_BOUND ( 'NONE', #7884, .T. ) ;
#26128=CARTESIAN_POINT ( 'NONE',  ( -40.77202656396519131, 129.1845453850527576, -17.01159430929711291 ) ) ;
#26132=LINE ( 'NONE', #19810, #27639 ) ;
#26135=CYLINDRICAL_SURFACE ( 'NONE', #9630, 58.59270260175150469 ) ;
#26139=ORIENTED_EDGE ( 'NONE', *, *, #24, .T. ) ;
#26140=CARTESIAN_POINT ( 'NONE',  ( -226.9732155144656360, 87.81596337922499629, -15.90667162794334466 ) ) ;
#26147=ORIENTED_EDGE ( 'NONE', *, *, #27368, .T. ) ;
#26148=CARTESIAN_POINT ( 'NONE',  ( 65.00000000000000000, -120.0250000000000625, 64.00000000000001421 ) ) ;
#26152=ORIENTED_EDGE ( 'NONE', *, *, #4570, .F. ) ;
#26153=CARTESIAN_POINT ( 'NONE',  ( 109.6721745451464045, 96.60743919220468001, -100.0000000000000142 ) ) ;
#26158=CARTESIAN_POINT ( 'NONE',  ( -215.0606129237200719, 86.58168940511831124, 21.65971791556373205 ) ) ;
#26159=ORIENTED_EDGE ( 'NONE', *, *, #8286, .T. ) ;
#26161=B_SPLINE_CURVE_WITH_KNOTS ( 'NONE', 3,
 ( #715, #5155, #2565, #26851, #4576, #9483, #22692, #26550, #17797, #18238, #20239, #18379, #11788, #20526, #15812, #13362, #851, #15948, #7319, #5007, #11202, #9335 ),
 .UNSPECIFIED., .F., .F.,
 ( 4, 2, 2, 2, 2, 2, 2, 2, 2, 2, 4 ),
 ( 0.000000000000000000, 0.1250000000000000000, 0.2500000000000000000, 0.3750000000000000000, 0.5000000000000000000, 0.6250000000000000000, 0.7500000000000000000, 0.8125000000000000000, 0.8750000000000001110, 0.9375000000000001110, 1.000000000000000000 ),
 .UNSPECIFIED. ) ;
#26162=DIRECTION ( 'NONE',  ( -0.9586565047779721516, -0.2845658198851048759, 0.000000000000000000 ) ) ;
#26163=DIRECTION ( 'NONE',  ( 1.000000000000000000, -0.000000000000000000, -0.000000000000000000 ) ) ;
#26164=DIRECTION ( 'NONE',  ( -0.000000000000000000, -0.000000000000000000, 1.000000000000000000 ) ) ;
#26167=CARTESIAN_POINT ( 'NONE',  ( 118.3245732435417068, 204.8512006320913486, 99.88685888571269800 ) ) ;
#26170=CARTESIAN_POINT ( 'NONE',  ( -63.57415822541634043, -18.01420295945611727, 95.00000000000000000 ) ) ;
#26172=PLANE ( 'NONE',  #8708 ) ;
#26173=CIRCLE ( 'NONE', #9210, 21.49999999999997868 ) ;
#26175=DIRECTION ( 'NONE',  ( 1.000000000000000000, 2.602085213965211135E-16, -0.000000000000000000 ) ) ;
#26176=B_SPLINE_CURVE_WITH_KNOTS ( 'NONE', 3,
 ( #13825, #2885, #9506, #7348, #9644, #3154, #18401, #5322, #27151, #16392, #11946, #5456, #14240, #22990, #16257, #3293, #20685, #20830, #9922, #18675, #7056, #15838, #21532, #14943, #25280, #16807, #25422, #5600, #12505, #18813, #5879, #16670, #7763, #18960, #7897, #25554, #25842, #8041 ),
 .UNSPECIFIED., .F., .F.,
 ( 4, 2, 2, 2, 2, 2, 2, 2, 2, 2, 2, 2, 2, 2, 2, 2, 2, 2, 4 ),
 ( 0.000000000000000000, 0.003178314472605698292, 0.004767471708908553943, 0.006356628945211410461, 0.007945786181514265245, 0.009534943417817123498, 0.01271325789042283480, 0.01430241512672566877, 0.01589157236302849927, 0.01906988683563421577, 0.02542651578084565225, 0.02860483025345133060, 0.03178314472605699853, 0.03813977367126838991, 0.04449640261647971884, 0.04767471708908538330, 0.04926387432538828492, 0.05005845294353974267, 0.05085303156169119349 ),
 .UNSPECIFIED. ) ;
#26180=LINE ( 'NONE', #17997, #554 ) ;
#26181=CARTESIAN_POINT ( 'NONE',  ( -187.3254023397375363, 105.2541933103603782, -31.76634463011786380 ) ) ;
#26185=EDGE_CURVE ( 'NONE', #230, #5960, #769, .T. ) ;
#26188=ORIENTED_EDGE ( 'NONE', *, *, #11307, .T. ) ;
#26189=ORIENTED_EDGE ( 'NONE', *, *, #18044, .F. ) ;
#26190=CARTESIAN_POINT ( 'NONE',  ( -3.611973201795212418, 132.7557511336061395, 15.88408374257556055 ) ) ;
#26191=AXIS2_PLACEMENT_3D ( 'NONE', #4155, #8623, #17373 ) ;
#26193=CARTESIAN_POINT ( 'NONE',  ( -225.7036482868739427, -91.18033988749901653, -18.91107291867258766 ) ) ;
#26196=CARTESIAN_POINT ( 'NONE',  ( -210.0000000000000000, -150.0000000000001990, 100.0000000000000142 ) ) ;
#26198=VERTEX_POINT ( 'NONE', #15145 ) ;
#26200=CARTESIAN_POINT ( 'NONE',  ( -2.862293735361731706E-14, 109.9999999999999858, 100.0000000000000142 ) ) ;
#26203=CARTESIAN_POINT ( 'NONE',  ( 113.5875366493131509, 226.9823751442990840, -97.68174538100610960 ) ) ;
#26207=AXIS2_PLACEMENT_3D ( 'NONE', #15345, #26375, #15916 ) ;
#26208=CARTESIAN_POINT ( 'NONE',  ( -77.29631966220712513, 4.740818392941735127, -15.00000000000000000 ) ) ;
#26215=CARTESIAN_POINT ( 'NONE',  ( -229.0277751032626838, 74.22523041939535915, 16.53402846819822614 ) ) ;
#26218=VERTEX_POINT ( 'NONE', #28325 ) ;
#26220=EDGE_CURVE ( 'NONE', #26801, #27657, #4423, .T. ) ;
#26225=DIRECTION ( 'NONE',  ( 0.000000000000000000, 0.000000000000000000, 1.000000000000000000 ) ) ;
#26227=CARTESIAN_POINT ( 'NONE',  ( 157.4999999999998579, 220.0000000000000284, 100.0000000000000142 ) ) ;
#26230=DIRECTION ( 'NONE',  ( 1.000000000000000000, 0.000000000000000000, 0.000000000000000000 ) ) ;
#26231=AXIS2_PLACEMENT_3D ( 'NONE', #11690, #18559, #20707 ) ;
#26233=EDGE_CURVE ( 'NONE', #24201, #20577, #318, .T. ) ;
#26234=AXIS2_PLACEMENT_3D ( 'NONE', #18033, #25197, #929 ) ;
#26236=CARTESIAN_POINT ( 'NONE',  ( 157.4999999999998579, 220.0000000000000284, -105.0000000000000284 ) ) ;
#26237=CARTESIAN_POINT ( 'NONE',  ( -209.0446251875730752, 89.43114028902917312, -24.28448859940165860 ) ) ;
#26245=CYLINDRICAL_SURFACE ( 'NONE', #14727, 2.000000000000000000 ) ;
#26246=EDGE_CURVE ( 'NONE', #12221, #24936, #11798, .T. ) ;
#26247=CARTESIAN_POINT ( 'NONE',  ( 112.0033315760181267, 140.0000000000000000, 96.14546719974917721 ) ) ;
#26254=CARTESIAN_POINT ( 'NONE',  ( -175.0000000000000000, -120.0250000000001762, 76.00000000000002842 ) ) ;
#26256=CARTESIAN_POINT ( 'NONE',  ( -1.286675988402057991, 135.5503650875635344, -13.59707690229856247 ) ) ;
#26258=AXIS2_PLACEMENT_3D ( 'NONE', #9204, #13667, #16106 ) ;
#26261=ORIENTED_EDGE ( 'NONE', *, *, #3680, .F. ) ;
#26268=CARTESIAN_POINT ( 'NONE',  ( -215.3445465745180343, 71.74628434702681545, 26.24848034640717032 ) ) ;
#26275=CIRCLE ( 'NONE', #9782, 55.86582179324592090 ) ;
#26278=AXIS2_PLACEMENT_3D ( 'NONE', #1244, #7717, #25096 ) ;
#26280=CARTESIAN_POINT ( 'NONE',  ( -38.15920525445427103, 129.9964506885557967, 15.32335565452434523 ) ) ;
#26281=EDGE_CURVE ( 'NONE', #4081, #14018, #23340, .T. ) ;
#26283=CARTESIAN_POINT ( 'NONE',  ( -169.4960802787495027, 115.4387886157293650, 26.69851561402025197 ) ) ;
#26285=ORIENTED_EDGE ( 'NONE', *, *, #22353, .T. ) ;
#26286=ORIENTED_EDGE ( 'NONE', *, *, #8000, .F. ) ;
#26288=CARTESIAN_POINT ( 'NONE',  ( -270.1025481742786951, -91.18033988749901653, 0.000000000000000000 ) ) ;
#26297=CARTESIAN_POINT ( 'NONE',  ( 104.4199312700659448, 89.58810137561040676, -100.0000000000000142 ) ) ;
#26300=CARTESIAN_POINT ( 'NONE',  ( -214.3655805135422838, 87.98073541835873357, 21.65873204582219813 ) ) ;
#26316=CYLINDRICAL_SURFACE ( 'NONE', #22172, 30.00000000000000000 ) ;
#26322=CARTESIAN_POINT ( 'NONE',  ( -192.2760768220978491, 101.7456562315031050, -32.00549636916782958 ) ) ;
#26323=ORIENTED_EDGE ( 'NONE', *, *, #22671, .F. ) ;
#26325=CARTESIAN_POINT ( 'NONE',  ( -114.8320768295896670, 71.54464929955101127, 82.80879831960035631 ) ) ;
#26329=ORIENTED_EDGE ( 'NONE', *, *, #17974, .F. ) ;
#26331=DIRECTION ( 'NONE',  ( 0.000000000000000000, 0.000000000000000000, -1.000000000000000000 ) ) ;
#26332=ADVANCED_FACE ( 'NONE', ( #8806 ), #4914, .T. ) ;
#26333=DIRECTION ( 'NONE',  ( 0.000000000000000000, -0.000000000000000000, -1.000000000000000000 ) ) ;
#26334=CARTESIAN_POINT ( 'NONE',  ( -217.2892621185082760, 109.4029876883478352, 12.99999999999999822 ) ) ;
#26341=EDGE_CURVE ( 'NONE', #20107, #8966, #22599, .T. ) ;
#26342=DIRECTION ( 'NONE',  ( 1.000000000000000000, -1.902611372570518757E-15, 0.000000000000000000 ) ) ;
#26350=PLANE ( 'NONE',  #20889 ) ;
#26355=CARTESIAN_POINT ( 'NONE',  ( -221.2437346188302172, 71.40151075288129334, 20.77520232899931685 ) ) ;
#26358=ORIENTED_EDGE ( 'NONE', *, *, #14843, .T. ) ;
#26359=ADVANCED_FACE ( 'NONE', ( #16282 ), #12263, .T. ) ;
#26364=CARTESIAN_POINT ( 'NONE',  ( -217.7546030100696157, 138.5587306369054659, 15.07876772300363477 ) ) ;
#26365=AXIS2_PLACEMENT_3D ( 'NONE', #13360, #13082, #22109 ) ;
#26366=CARTESIAN_POINT ( 'NONE',  ( 91.66503723322182395, 240.0531355366313448, 6.981029948440133914 ) ) ;
#26367=ADVANCED_FACE ( 'NONE', ( #13848 ), #9951, .T. ) ;
#26374=CARTESIAN_POINT ( 'NONE',  ( 89.99999999999994316, -70.00000000000001421, -25.00000000000000711 ) ) ;
#26375=DIRECTION ( 'NONE',  ( 0.000000000000000000, 0.000000000000000000, 1.000000000000000000 ) ) ;
#26380=ADVANCED_FACE ( 'NONE', ( #13704 ), #15919, .T. ) ;
#26382=VECTOR ( 'NONE', #6451, 1000.000000000000000 ) ;
#26384=ORIENTED_EDGE ( 'NONE', *, *, #3709, .F. ) ;
#26388=CARTESIAN_POINT ( 'NONE',  ( -24.84958620104691818, 129.2502933934031262, -15.64834371897906173 ) ) ;
#26393=ORIENTED_EDGE ( 'NONE', *, *, #4470, .T. ) ;
#26397=DIRECTION ( 'NONE',  ( -0.000000000000000000, -0.000000000000000000, -1.000000000000000000 ) ) ;
#26399=DIRECTION ( 'NONE',  ( -0.000000000000000000, 1.000000000000000000, -1.387778780781445429E-16 ) ) ;
#26400=VECTOR ( 'NONE', #14623, 1000.000000000000000 ) ;
#26405=CARTESIAN_POINT ( 'NONE',  ( -214.2313421016903021, 58.42887478691795167, 32.84133050938623910 ) ) ;
#26408=CARTESIAN_POINT ( 'NONE',  ( -76.25760768171835480, 221.6666220619077876, 12.99999999999999822 ) ) ;
#26414=CARTESIAN_POINT ( 'NONE',  ( -208.6312261275415665, 71.65289352654478705, 39.58303953460989533 ) ) ;
#26419=CARTESIAN_POINT ( 'NONE',  ( -169.3459405269803995, 115.5129628772605201, 26.63562761174981119 ) ) ;
#26420=FACE_OUTER_BOUND ( 'NONE', #10072, .T. ) ;
#26422=ORIENTED_EDGE ( 'NONE', *, *, #3536, .T. ) ;
#26424=EDGE_LOOP ( 'NONE', ( #6321, #2577, #21700, #16963 ) ) ;
#26425=CARTESIAN_POINT ( 'NONE',  ( -216.6285223362424119, 139.2238150404710382, -13.00000000000000000 ) ) ;
#26426=CARTESIAN_POINT ( 'NONE',  ( -160.5161435040798494, 120.3804527765386609, 22.28951900308576128 ) ) ;
#26428=AXIS2_PLACEMENT_3D ( 'NONE', #26200, #21611, #24062 ) ;
#26429=ADVANCED_FACE ( 'NONE', ( #336 ), #18287, .T. ) ;
#26430=CARTESIAN_POINT ( 'NONE',  ( 119.7545560452836639, 132.4900181920934870, -100.0000000000000142 ) ) ;
#26431=EDGE_CURVE ( 'NONE', #17375, #27481, #25035, .T. ) ;
#26432=CYLINDRICAL_SURFACE ( 'NONE', #17405, 22.49999999999999289 ) ;
#26434=CARTESIAN_POINT ( 'NONE',  ( -212.5539796181134591, 88.28323935596885974, 22.89445012289458603 ) ) ;
#26441=CARTESIAN_POINT ( 'NONE',  ( -218.8273392347107631, 140.3457761587572747, -14.99191580167153681 ) ) ;
#26447=CARTESIAN_POINT ( 'NONE',  ( -160.8326600028555902, 120.2355194873575073, 21.37420696376536711 ) ) ;
#26449=ORIENTED_EDGE ( 'NONE', *, *, #25377, .F. ) ;
#26452=CARTESIAN_POINT ( 'NONE',  ( -196.6099257382077496, 98.46903227932085656, -31.30702426071320943 ) ) ;
#26453=ORIENTED_EDGE ( 'NONE', *, *, #8348, .F. ) ;
#26454=EDGE_CURVE ( 'NONE', #11803, #8966, #2617, .T. ) ;
#26456=ORIENTED_EDGE ( 'NONE', *, *, #6112, .F. ) ;
#26460=DIRECTION ( 'NONE',  ( 0.000000000000000000, 1.000000000000000000, 0.000000000000000000 ) ) ;
#26469=CARTESIAN_POINT ( 'NONE',  ( -209.0137638338787269, 69.92154464606612407, -37.51858872986124283 ) ) ;
#26472=DIRECTION ( 'NONE',  ( 0.000000000000000000, 0.000000000000000000, 1.000000000000000000 ) ) ;
#26474=CYLINDRICAL_SURFACE ( 'NONE', #25173, 89.71075545852266941 ) ;
#26475=CARTESIAN_POINT ( 'NONE',  ( 65.00000000000000000, -120.0000000000000711, 63.97500000000001563 ) ) ;
#26476=CIRCLE ( 'NONE', #19627, 5.000000000000004441 ) ;
#26478=CARTESIAN_POINT ( 'NONE',  ( -225.0350560533458690, 62.39407306348317661, 8.837833373942171278 ) ) ;
#26483=ORIENTED_EDGE ( 'NONE', *, *, #6497, .T. ) ;
#26495=VERTEX_POINT ( 'NONE', #3466 ) ;
#26502=CARTESIAN_POINT ( 'NONE',  ( 93.26488863017658559, 240.2518291191169340, 7.855680688306072135 ) ) ;
#26503=EDGE_CURVE ( 'NONE', #1515, #23197, #18226, .T. ) ;
#26510=SPHERICAL_SURFACE ( 'NONE', #18195, 5.000000000000000000 ) ;
#26511=DIRECTION ( 'NONE',  ( 1.000000000000000000, 0.000000000000000000, 0.000000000000000000 ) ) ;
#26513=CARTESIAN_POINT ( 'NONE',  ( -143.6428522700808230, 71.54464929955099706, 83.00000000000001421 ) ) ;
#26514=DIRECTION ( 'NONE',  ( 0.6533458216954761699, -0.7570595995514904919, 0.000000000000000000 ) ) ;
#26516=PLANE ( 'NONE',  #11524 ) ;
#26525=CARTESIAN_POINT ( 'NONE',  ( 108.2753065237224774, 248.3531133182295321, -34.86527342668098584 ) ) ;
#26527=CARTESIAN_POINT ( 'NONE',  ( 134.9999999999998579, 220.0000000000000284, 90.00000000000002842 ) ) ;
#26530=AXIS2_PLACEMENT_3D ( 'NONE', #717, #18239, #15025 ) ;
#26534=ORIENTED_EDGE ( 'NONE', *, *, #13688, .T. ) ;
#26535=CARTESIAN_POINT ( 'NONE',  ( 134.9999999999998579, 220.0000000000000284, 99.00000000000001421 ) ) ;
#26540=CIRCLE ( 'NONE', #13255, 30.00000000000000000 ) ;
#26544=CARTESIAN_POINT ( 'NONE',  ( -226.6532499065066020, 62.99057865342218321, 8.245540320826911795 ) ) ;
#26545=PLANE ( 'NONE',  #22738 ) ;
#26548=LINE ( 'NONE', #6880, #14014 ) ;
#26550=CARTESIAN_POINT ( 'NONE',  ( 101.7779539749746931, 119.2876405404125393, 82.50000000030260594 ) ) ;
#26553=CIRCLE ( 'NONE', #17848, 10.00000000000000888 ) ;
#26554=CARTESIAN_POINT ( 'NONE',  ( 7.501147730487500276, 138.6545231272701528, 14.99999999999999467 ) ) ;
#26556=AXIS2_PLACEMENT_3D ( 'NONE', #4111, #12895, #4254 ) ;
#26557=CARTESIAN_POINT ( 'NONE',  ( 184.9999999999999147, -150.0000000000000284, -84.99999999999997158 ) ) ;
#26558=CARTESIAN_POINT ( 'NONE',  ( -28.05246235954390244, 188.0718642840173516, 12.99999999999999822 ) ) ;
#26560=EDGE_LOOP ( 'NONE', ( #20697, #6889, #22489, #20979, #19762, #13634, #3502, #19233 ) ) ;
#26561=FACE_OUTER_BOUND ( 'NONE', #44, .T. ) ;
#26564=DIRECTION ( 'NONE',  ( 0.000000000000000000, 0.000000000000000000, -1.000000000000000000 ) ) ;
#26567=AXIS2_PLACEMENT_3D ( 'NONE', #204, #8965, #4222 ) ;
#26568=CONICAL_SURFACE ( 'NONE', #21530, 18.91107291867258411, 0.08885387018394237668 ) ;
#26571=CARTESIAN_POINT ( 'NONE',  ( -158.3304926817754676, 121.3760726389792666, 21.42757541440370872 ) ) ;
#26574=CARTESIAN_POINT ( 'NONE',  ( -42.53273978471831640, 130.9733465240572627, 14.93735646117640847 ) ) ;
#26577=CIRCLE ( 'NONE', #10026, 14.64217782292691261 ) ;
#26584=CARTESIAN_POINT ( 'NONE',  ( -195.7913036700337841, 62.61587363931871408, -36.00381397819591456 ) ) ;
#26588=CARTESIAN_POINT ( 'NONE',  ( -223.0228900756071653, 134.9178336739567499, -12.97939780113087060 ) ) ;
#26591=VERTEX_POINT ( 'NONE', #14264 ) ;
#26593=CARTESIAN_POINT ( 'NONE',  ( -175.8417606860892874, 246.9430296707336652, 12.99999999999999822 ) ) ;
#26594=ADVANCED_FACE ( 'NONE', ( #1036 ), #20928, .F. ) ;
#26597=LINE ( 'NONE', #24746, #4366 ) ;
#26601=AXIS2_PLACEMENT_3D ( 'NONE', #23604, #12841, #1622 ) ;
#26602=CARTESIAN_POINT ( 'NONE',  ( -236.8177751472017007, 82.33896643611701904, 5.000000000000002665 ) ) ;
#26605=ORIENTED_EDGE ( 'NONE', *, *, #5098, .T. ) ;
#26609=ORIENTED_EDGE ( 'NONE', *, *, #8389, .T. ) ;
#26611=CARTESIAN_POINT ( 'NONE',  ( -266.5839533485339530, -91.18033988749901653, 0.000000000000000000 ) ) ;
#26612=AXIS2_PLACEMENT_3D ( 'NONE', #21758, #26617, #2200 ) ;
#26615=CARTESIAN_POINT ( 'NONE',  ( -7.828161053703414751, 131.1970564781817643, -16.31839186148043552 ) ) ;
#26617=DIRECTION ( 'NONE',  ( 0.000000000000000000, 1.000000000000000000, -0.000000000000000000 ) ) ;
#26619=LINE ( 'NONE', #9108, #8061 ) ;
#26630=EDGE_CURVE ( 'NONE', #14597, #25416, #9510, .T. ) ;
#26631=CARTESIAN_POINT ( 'NONE',  ( -175.0000000000000000, -120.0000000000001847, -69.99999999999998579 ) ) ;
#26632=FACE_OUTER_BOUND ( 'NONE', #26059, .T. ) ;
#26634=ORIENTED_EDGE ( 'NONE', *, *, #13201, .F. ) ;
#26637=AXIS2_PLACEMENT_3D ( 'NONE', #9617, #13944, #7317 ) ;
#26638=CARTESIAN_POINT ( 'NONE',  ( -222.0899288397881435, 71.52493653041949528, 20.17326427264749711 ) ) ;
#26640=DIRECTION ( 'NONE',  ( 0.000000000000000000, 0.000000000000000000, -1.000000000000000000 ) ) ;
#26642=VERTEX_POINT ( 'NONE', #26574 ) ;
#26643=CARTESIAN_POINT ( 'NONE',  ( 134.9999999999998579, 220.0000000000000284, 84.99999999999995737 ) ) ;
#26644=ORIENTED_EDGE ( 'NONE', *, *, #5300, .T. ) ;
#26645=CIRCLE ( 'NONE', #28023, 11.42311362948588105 ) ;
#26648=CARTESIAN_POINT ( 'NONE',  ( 105.1668099567775414, 241.3986356328032628, 28.65150506303233513 ) ) ;
#26654=CARTESIAN_POINT ( 'NONE',  ( 115.6411010564578561, 208.5333949360010308, 99.00000000000001421 ) ) ;
#26661=CARTESIAN_POINT ( 'NONE',  ( 119.9999999999999147, 203.2294901687515676, 100.0000000000000142 ) ) ;
#26665=VECTOR ( 'NONE', #13627, 1000.000000000000114 ) ;
#26670=ORIENTED_EDGE ( 'NONE', *, *, #22462, .T. ) ;
#26675=ORIENTED_EDGE ( 'NONE', *, *, #16351, .T. ) ;
#26678=VERTEX_POINT ( 'NONE', #22712 ) ;
#26681=VERTEX_POINT ( 'NONE', #24862 ) ;
#26687=ADVANCED_FACE ( 'NONE', ( #11805 ), #9502, .F. ) ;
#26689=CARTESIAN_POINT ( 'NONE',  ( -221.7690971916811407, 71.47334710437667127, 20.39711061091035305 ) ) ;
#26691=ADVANCED_FACE ( 'NONE', ( #15683 ), #22131, .F. ) ;
#26701=CARTESIAN_POINT ( 'NONE',  ( -210.0000000000000284, -3.238150488490040751E-14, 70.00000000000001421 ) ) ;
#26708=DIRECTION ( 'NONE',  ( 1.000000000000000000, 1.530283246943720875E-16, -0.000000000000000000 ) ) ;
#26712=CARTESIAN_POINT ( 'NONE',  ( -209.0165584120921096, 88.62137859748428070, -26.02317696115059320 ) ) ;
#26714=ORIENTED_EDGE ( 'NONE', *, *, #17792, .T. ) ;
#26717=CARTESIAN_POINT ( 'NONE',  ( -134.0236137306590365, 130.0100214678653003, 15.30004249603843469 ) ) ;
#26719=ORIENTED_EDGE ( 'NONE', *, *, #17819, .F. ) ;
#26721=EDGE_CURVE ( 'NONE', #10524, #27001, #24578, .T. ) ;
#26724=AXIS2_PLACEMENT_3D ( 'NONE', #26631, #18028, #20175 ) ;
#26727=CARTESIAN_POINT ( 'NONE',  ( -205.5899716318703554, 91.23091416471392279, 28.02219806143363812 ) ) ;
#26729=CIRCLE ( 'NONE', #6849, 9.999999999999982236 ) ;
#26734=DIRECTION ( 'NONE',  ( 0.000000000000000000, 0.000000000000000000, 1.000000000000000000 ) ) ;
#26735=CARTESIAN_POINT ( 'NONE',  ( -204.6417490964368540, 60.41478268044598110, -22.13567842568586030 ) ) ;
#26736=ORIENTED_EDGE ( 'NONE', *, *, #3905, .T. ) ;
#26738=CARTESIAN_POINT ( 'NONE',  ( 32.36067977499786252, -40.00000000000003553, 100.0000000000000142 ) ) ;
#26742=CIRCLE ( 'NONE', #24003, 22.49999999999999289 ) ;
#26745=EDGE_CURVE ( 'NONE', #21631, #14873, #18397, .T. ) ;
#26747=CARTESIAN_POINT ( 'NONE',  ( 79.99999999999994316, 1.480297366166874546E-14, -45.00000000000000000 ) ) ;
#26748=LINE ( 'NONE', #2318, #7113 ) ;
#26749=ORIENTED_EDGE ( 'NONE', *, *, #23521, .F. ) ;
#26752=ORIENTED_EDGE ( 'NONE', *, *, #5684, .T. ) ;
#26755=CARTESIAN_POINT ( 'NONE',  ( -202.3850906029173018, 93.73590935844725891, -29.14524087624419124 ) ) ;
#26759=EDGE_CURVE ( 'NONE', #26495, #4081, #4595, .T. ) ;
#26763=LINE ( 'NONE', #20578, #25196 ) ;
#26765=ADVANCED_FACE ( 'NONE', ( #20967 ), #10875, .F. ) ;
#26767=FACE_OUTER_BOUND ( 'NONE', #4480, .T. ) ;
#26773=CARTESIAN_POINT ( 'NONE',  ( -3.523879052116754895, 132.7919533277021742, -15.87505980800028560 ) ) ;
#26776=CARTESIAN_POINT ( 'NONE',  ( -230.8916957670046486, 130.8330661503598833, 15.00000000000000000 ) ) ;
#26779=CARTESIAN_POINT ( 'NONE',  ( -175.0000000000000000, -120.0000000000001705, 70.00000000000001421 ) ) ;
#26780=CARTESIAN_POINT ( 'NONE',  ( -190.0000000000000284, -40.00000000000004974, 80.00000000000001421 ) ) ;
#26784=CARTESIAN_POINT ( 'NONE',  ( -160.0000000000000284, 79.99999999999994316, 100.0000000000000142 ) ) ;
#26792=ORIENTED_EDGE ( 'NONE', *, *, #26829, .F. ) ;
#26793=AXIS2_PLACEMENT_3D ( 'NONE', #11049, #19803, #126 ) ;
#26801=VERTEX_POINT ( 'NONE', #20682 ) ;
#26802=EDGE_LOOP ( 'NONE', ( #2903, #7182, #4450, #10076 ) ) ;
#26804=ORIENTED_EDGE ( 'NONE', *, *, #22187, .T. ) ;
#26805=EDGE_CURVE ( 'NONE', #15968, #14227, #24182, .T. ) ;
#26806=CARTESIAN_POINT ( 'NONE',  ( 93.32984351717924199, 231.0185867901168137, 18.11991709984934573 ) ) ;
#26807=EDGE_CURVE ( 'NONE', #19092, #13809, #21246, .T. ) ;
#26809=CARTESIAN_POINT ( 'NONE',  ( -229.2498027451138967, 132.0565166830976978, -15.00000000000000000 ) ) ;
#26813=DIRECTION ( 'NONE',  ( -8.673617379884073683E-17, -1.000000000000000000, 0.000000000000000000 ) ) ;
#26818=CARTESIAN_POINT ( 'NONE',  ( 65.00000000000000000, -120.0000000000000995, -76.02499999999999147 ) ) ;
#26829=EDGE_CURVE ( 'NONE', #15645, #970, #15023, .T. ) ;
#26830=CARTESIAN_POINT ( 'NONE',  ( -40.40953891503691153, 0.000000000000000000, 99.00000000000000000 ) ) ;
#26833=ORIENTED_EDGE ( 'NONE', *, *, #5425, .F. ) ;
#26836=CARTESIAN_POINT ( 'NONE',  ( -190.0000000000000284, 59.99999999999995026, 110.0000000000000284 ) ) ;
#26838=DIRECTION ( 'NONE',  ( 8.659560562354934091E-17, 0.7071067811865474617, -0.7071067811865476838 ) ) ;
#26841=DIRECTION ( 'NONE',  ( 1.000000000000000000, -0.000000000000000000, -0.000000000000000000 ) ) ;
#26843=CARTESIAN_POINT ( 'NONE',  ( -230.0306293838742988, 64.31401865985674249, 16.82661551914410225 ) ) ;
#26846=DIRECTION ( 'NONE',  ( -1.000000000000000000, -0.000000000000000000, -0.000000000000000000 ) ) ;
#26851=CARTESIAN_POINT ( 'NONE',  ( 108.2273028572102760, 129.5338070841179672, 88.59375000028596503 ) ) ;
#26853=CARTESIAN_POINT ( 'NONE',  ( -13.62884545128598823, 130.9145211729554603, 16.37206327941867201 ) ) ;
#26860=CARTESIAN_POINT ( 'NONE',  ( -200.0000000000000284, -91.18033988749901653, 0.000000000000000000 ) ) ;
#26861=CARTESIAN_POINT ( 'NONE',  ( 33.10302365956999182, 203.2034914284457159, 15.00000000000000000 ) ) ;
#26863=VERTEX_POINT ( 'NONE', #14513 ) ;
#26865=EDGE_CURVE ( 'NONE', #19837, #18244, #7227, .T. ) ;
#26872=VECTOR ( 'NONE', #25362, 1000.000000000000114 ) ;
#26877=ORIENTED_EDGE ( 'NONE', *, *, #11713, .T. ) ;
#26883=FACE_OUTER_BOUND ( 'NONE', #17354, .T. ) ;
#26884=CARTESIAN_POINT ( 'NONE',  ( -210.9349024751243178, 73.41979635535319915, -32.58420779144454826 ) ) ;
#26888=CARTESIAN_POINT ( 'NONE',  ( -229.2498027451138967, 132.0565166830976978, -15.00000000000000178 ) ) ;
#26894=LINE ( 'NONE', #20284, #21205 ) ;
#26895=CARTESIAN_POINT ( 'NONE',  ( -143.2374437020967264, 68.51688903468615877, 83.00000000000001421 ) ) ;
#26898=ORIENTED_EDGE ( 'NONE', *, *, #27579, .T. ) ;
#26906=DIRECTION ( 'NONE',  ( 0.000000000000000000, 0.000000000000000000, 1.000000000000000000 ) ) ;
#26914=CARTESIAN_POINT ( 'NONE',  ( 1.655276743323666810, 135.1741146306952430, -15.36901953696933987 ) ) ;
#26915=CIRCLE ( 'NONE', #9937, 1.999999999999994893 ) ;
#26916=DIRECTION ( 'NONE',  ( 0.8018642810807398158, 0.5975062131282554700, -0.000000000000000000 ) ) ;
#26923=DIRECTION ( 'NONE',  ( 1.000000000000000000, 0.000000000000000000, 0.000000000000000000 ) ) ;
#26930=CARTESIAN_POINT ( 'NONE',  ( -224.2511286692390229, 62.13136325095025825, -9.143584677369513969 ) ) ;
#26932=ORIENTED_EDGE ( 'NONE', *, *, #7639, .T. ) ;
#26933=FACE_OUTER_BOUND ( 'NONE', #28149, .T. ) ;
#26935=AXIS2_PLACEMENT_3D ( 'NONE', #763, #9529, #27039 ) ;
#26936=LINE ( 'NONE', #20610, #15287 ) ;
#26944=ORIENTED_EDGE ( 'NONE', *, *, #18787, .T. ) ;
#26945=ORIENTED_EDGE ( 'NONE', *, *, #1695, .T. ) ;
#26947=FACE_OUTER_BOUND ( 'NONE', #9812, .T. ) ;
#26948=DIRECTION ( 'NONE',  ( -0.000000000000000000, 1.000000000000000000, -1.387778780781445429E-16 ) ) ;
#26949=CIRCLE ( 'NONE', #21446, 5.000000000000004441 ) ;
#26950=CARTESIAN_POINT ( 'NONE',  ( 109.9999999999999147, 137.0808454112663810, -89.99999999930710715 ) ) ;
#26952=CARTESIAN_POINT ( 'NONE',  ( 8.117852850209656523, 141.5785587194356481, 12.99999999999999822 ) ) ;
#26953=DIRECTION ( 'NONE',  ( -0.000000000000000000, -0.000000000000000000, 1.000000000000000000 ) ) ;
#26954=CARTESIAN_POINT ( 'NONE',  ( 87.50000000000029843, 230.0000000000000284, -15.95262490344447492 ) ) ;
#26956=DIRECTION ( 'NONE',  ( 1.000000000000000000, 0.000000000000000000, 0.000000000000000000 ) ) ;
#26957=DIRECTION ( 'NONE',  ( -0.7123733896039576852, -0.6147814225729698601, -0.3384788859638417913 ) ) ;
#26958=EDGE_LOOP ( 'NONE', ( #9944, #27735, #20171, #27546, #24818, #26082, #18768, #23260 ) ) ;
#26965=AXIS2_PLACEMENT_3D ( 'NONE', #11949, #13827, #7352 ) ;
#26972=ORIENTED_EDGE ( 'NONE', *, *, #23624, .F. ) ;
#26974=CARTESIAN_POINT ( 'NONE',  ( -160.8326600028555902, 120.2355194873575073, 21.37420696376536711 ) ) ;
#26975=LINE ( 'NONE', #18082, #3314 ) ;
#26976=CARTESIAN_POINT ( 'NONE',  ( -62.43823629548968768, 134.9066984251663825, -13.78087915458745627 ) ) ;
#26977=CARTESIAN_POINT ( 'NONE',  ( 33.10302365956999182, 203.2034914284457159, -13.00000000000000000 ) ) ;
#26978=CARTESIAN_POINT ( 'NONE',  ( -195.7913036700337841, 62.61587363931871408, 36.00381397819591456 ) ) ;
#26981=CARTESIAN_POINT ( 'NONE',  ( -62.43610812620287476, 134.9063932224630094, -13.78094890389263938 ) ) ;
#26989=CARTESIAN_POINT ( 'NONE',  ( 0.8462782258048142658, 136.6959233578304236, 15.12258877882598007 ) ) ;
#26992=EDGE_CURVE ( 'NONE', #4186, #13809, #5391, .T. ) ;
#26994=VERTEX_POINT ( 'NONE', #13209 ) ;
#26996=CARTESIAN_POINT ( 'NONE',  ( -217.9749057636497582, 86.24598930254806817, -19.84474727259476978 ) ) ;
#26997=EDGE_CURVE ( 'NONE', #11481, #11333, #17776, .T. ) ;
#26998=EDGE_CURVE ( 'NONE', #18102, #8949, #19153, .T. ) ;
#27001=VERTEX_POINT ( 'NONE', #6165 ) ;
#27002=VERTEX_POINT ( 'NONE', #19523 ) ;
#27005=CARTESIAN_POINT ( 'NONE',  ( -135.0977962388534763, 129.7097216771591661, 16.78759912078217553 ) ) ;
#27017=CARTESIAN_POINT ( 'NONE',  ( -214.0051257764050945, 55.38571953469315901, -43.60894023861363422 ) ) ;
#27023=DIRECTION ( 'NONE',  ( 1.000000000000000000, 0.000000000000000000, 0.000000000000000000 ) ) ;
#27024=CARTESIAN_POINT ( 'NONE',  ( 124.9999999999998579, 220.0000000000000284, 90.00000000000002842 ) ) ;
#27028=EDGE_CURVE ( 'NONE', #7114, #15531, #26949, .T. ) ;
#27029=DIRECTION ( 'NONE',  ( 0.9960550913260673989, 1.086714821493789192E-17, 0.08873699929240025375 ) ) ;
#27036=ORIENTED_EDGE ( 'NONE', *, *, #11141, .T. ) ;
#27039=DIRECTION ( 'NONE',  ( 0.000000000000000000, 0.000000000000000000, -1.000000000000000000 ) ) ;
#27040=CIRCLE ( 'NONE', #10518, 5.000000000000004441 ) ;
#27046=LINE ( 'NONE', #1185, #5643 ) ;
#27050=CARTESIAN_POINT ( 'NONE',  ( -22.99863117501815069, 128.1622734824785823, -17.43423781283663132 ) ) ;
#27054=ADVANCED_FACE ( 'NONE', ( #15223 ), #21954, .T. ) ;
#27055=VERTEX_POINT ( 'NONE', #2263 ) ;
#27056=AXIS2_PLACEMENT_3D ( 'NONE', #6418, #9001, #28369 ) ;
#27058=CARTESIAN_POINT ( 'NONE',  ( -227.3657730843237346, 133.9833936510272565, 14.99191580167116733 ) ) ;
#27074=EDGE_CURVE ( 'NONE', #27404, #9161, #4001, .T. ) ;
#27075=CARTESIAN_POINT ( 'NONE',  ( 96.24937469161466197, 240.9969810907205954, 9.998609732053244770 ) ) ;
#27076=VERTEX_POINT ( 'NONE', #28398 ) ;
#27080=AXIS2_PLACEMENT_3D ( 'NONE', #12900, #23243, #25530 ) ;
#27081=EDGE_LOOP ( 'NONE', ( #8885, #6971, #17419, #3109, #15607 ) ) ;
#27084=DIRECTION ( 'NONE',  ( 1.000000000000000000, 0.000000000000000000, 0.000000000000000000 ) ) ;
#27085=AXIS2_PLACEMENT_3D ( 'NONE', #16307, #10117, #25475 ) ;
#27095=LINE ( 'NONE', #26513, #21955 ) ;
#27102=ORIENTED_EDGE ( 'NONE', *, *, #2904, .F. ) ;
#27104=AXIS2_PLACEMENT_3D ( 'NONE', #4045, #12555, #21296 ) ;
#27107=EDGE_LOOP ( 'NONE', ( #14064, #23251, #2004, #9207 ) ) ;
#27108=DIRECTION ( 'NONE',  ( -0.000000000000000000, -0.000000000000000000, 1.000000000000000000 ) ) ;
#27115=DIRECTION ( 'NONE',  ( 0.000000000000000000, 0.000000000000000000, 1.000000000000000000 ) ) ;
#27119=EDGE_CURVE ( 'NONE', #6791, #23180, #9032, .T. ) ;
#27122=CIRCLE ( 'NONE', #15207, 3.532530335305414493 ) ;
#27123=CARTESIAN_POINT ( 'NONE',  ( -207.6173544636101553, 75.51556044650348554, 42.73482814336003344 ) ) ;
#27125=CARTESIAN_POINT ( 'NONE',  ( -96.56864860929032091, 136.1733035486019787, -13.53429741579593681 ) ) ;
#27126=CARTESIAN_POINT ( 'NONE',  ( 79.99999999999997158, 106.9649888129831794, -83.29453619103985318 ) ) ;
#27128=EDGE_CURVE ( 'NONE', #12401, #11179, #24200, .T. ) ;
#27133=CARTESIAN_POINT ( 'NONE',  ( -201.6741895288615183, 93.98653502690473260, 30.48002917746099172 ) ) ;
#27134=CARTESIAN_POINT ( 'NONE',  ( -221.3650667873343139, -91.18033988749901653, 0.000000000000000000 ) ) ;
#27136=ORIENTED_EDGE ( 'NONE', *, *, #27140, .T. ) ;
#27137=AXIS2_PLACEMENT_3D ( 'NONE', #22077, #13760, #6844 ) ;
#27139=ORIENTED_EDGE ( 'NONE', *, *, #16504, .T. ) ;
#27140=EDGE_CURVE ( 'NONE', #3426, #18280, #26476, .T. ) ;
#27142=ORIENTED_EDGE ( 'NONE', *, *, #14327, .F. ) ;
#27143=AXIS2_PLACEMENT_3D ( 'NONE', #23536, #28110, #15063 ) ;
#27144=CARTESIAN_POINT ( 'NONE',  ( 134.9999999999998579, 220.0000000000000284, -90.00000000000002842 ) ) ;
#27145=CARTESIAN_POINT ( 'NONE',  ( -82.76390570603551566, 134.7701287218720552, 15.45937173543416066 ) ) ;
#27151=CARTESIAN_POINT ( 'NONE',  ( 94.28023193196015939, 231.3879991501505060, -18.61206014455101254 ) ) ;
#27154=ADVANCED_FACE ( 'NONE', ( #17783 ), #1712, .T. ) ;
#27155=CYLINDRICAL_SURFACE ( 'NONE', #11253, 5.000000000000004441 ) ;
#27156=AXIS2_PLACEMENT_3D ( 'NONE', #12150, #22636, #16033 ) ;
#27158=CARTESIAN_POINT ( 'NONE',  ( -215.6254804987312070, 60.26473849368080948, -13.41209097273894457 ) ) ;
#27164=VERTEX_POINT ( 'NONE', #5140 ) ;
#27165=DIRECTION ( 'NONE',  ( 0.5555587585212683477, 0.8314772792026894344, -0.000000000000000000 ) ) ;
#27166=CARTESIAN_POINT ( 'NONE',  ( -231.0952835391969415, 75.72709865442921284, 15.86948571459985047 ) ) ;
#27170=ORIENTED_EDGE ( 'NONE', *, *, #26039, .T. ) ;
#27173=CARTESIAN_POINT ( 'NONE',  ( 82.68942924499303615, 110.0997128786253683, 70.07812500014873081 ) ) ;
#27174=CARTESIAN_POINT ( 'NONE',  ( 79.99999999999990052, 140.0000000000000000, 15.00000000000000000 ) ) ;
#27178=DIRECTION ( 'NONE',  ( 1.000000000000000000, 0.000000000000000000, 0.000000000000000000 ) ) ;
#27180=DIRECTION ( 'NONE',  ( 1.000000000000000000, 0.000000000000000000, 0.000000000000000000 ) ) ;
#27182=ORIENTED_EDGE ( 'NONE', *, *, #7852, .F. ) ;
#27188=CARTESIAN_POINT ( 'NONE',  ( -279.3160071107327553, -91.18033988749901653, 0.000000000000000000 ) ) ;
#27190=CARTESIAN_POINT ( 'NONE',  ( -4.592061942444369826, 132.3627631488751604, -15.98545474231262098 ) ) ;
#27196=TOROIDAL_SURFACE ( 'NONE', #7919, 66.76834224489934400, 2.000000000000000000 ) ;
#27198=DIRECTION ( 'NONE',  ( 0.000000000000000000, -1.000000000000000000, -0.000000000000000000 ) ) ;
#27202=DIRECTION ( 'NONE',  ( 1.224646799147353207E-16, 1.000000000000000000, -0.000000000000000000 ) ) ;
#27207=CARTESIAN_POINT ( 'NONE',  ( 65.00000000000000000, -120.0000000000000995, -69.99999999999998579 ) ) ;
#27212=CARTESIAN_POINT ( 'NONE',  ( 102.1959223267361239, 244.1336238956074851, 16.70134980617025633 ) ) ;
#27218=EDGE_CURVE ( 'NONE', #3825, #10815, #23277, .T. ) ;
#27221=AXIS2_PLACEMENT_3D ( 'NONE', #18757, #7983, #1233 ) ;
#27222=CARTESIAN_POINT ( 'NONE',  ( 109.8801565119851205, 257.7417414023682340, 41.08725989918679034 ) ) ;
#27224=FACE_OUTER_BOUND ( 'NONE', #6607, .T. ) ;
#27229=EDGE_CURVE ( 'NONE', #23180, #8916, #11376, .T. ) ;
#27232=CARTESIAN_POINT ( 'NONE',  ( -236.8177751472017007, 82.33896643611701904, -15.00000000000000000 ) ) ;
#27233=CARTESIAN_POINT ( 'NONE',  ( -203.1779787704217313, 93.05164332230201296, -15.00000000000000000 ) ) ;
#27236=CARTESIAN_POINT ( 'NONE',  ( 134.9999999999998579, 220.0000000000000284, -105.0000000000000284 ) ) ;
#27237=CARTESIAN_POINT ( 'NONE',  ( 32.36067977499787673, 79.99999999999998579, 100.0000000000000142 ) ) ;
#27239=TOROIDAL_SURFACE ( 'NONE', #8429, 19.29759039828519818, 4.355764593064427537 ) ;
#27243=ORIENTED_EDGE ( 'NONE', *, *, #2274, .F. ) ;
#27244=DIRECTION ( 'NONE',  ( 1.000000000000000000, 0.000000000000000000, 0.000000000000000000 ) ) ;
#27245=ORIENTED_EDGE ( 'NONE', *, *, #22541, .F. ) ;
#27250=CARTESIAN_POINT ( 'NONE',  ( -149.5572648096271848, 124.9576791546268311, 17.81785897815565534 ) ) ;
#27251=TOROIDAL_SURFACE ( 'NONE', #5690, 14.95564396479129243, 3.532530335305412716 ) ;
#27253=CYLINDRICAL_SURFACE ( 'NONE', #8373, 30.00000000000000000 ) ;
#27254=CARTESIAN_POINT ( 'NONE',  ( -47.91567955387318989, 130.8829598292664969, -16.39210129961528040 ) ) ;
#27256=CARTESIAN_POINT ( 'NONE',  ( -13.76394398213074766, 130.8819511421725963, 14.96772766278609090 ) ) ;
#27259=CARTESIAN_POINT ( 'NONE',  ( -127.8584414339096185, 131.6633539443355687, -14.66583002116424517 ) ) ;
#27260=ADVANCED_FACE ( 'NONE', ( #1254 ), #23749, .T. ) ;
#27261=ADVANCED_FACE ( 'NONE', ( #3114 ), #20935, .T. ) ;
#27263=CARTESIAN_POINT ( 'NONE',  ( -205.2934542684511712, 91.43051335233271004, -27.40145609480763156 ) ) ;
#27268=CARTESIAN_POINT ( 'NONE',  ( 89.77759941121082932, 81.13568025369244197, -100.0000000000000142 ) ) ;
#27269=PLANE ( 'NONE',  #2414 ) ;
#27273=EDGE_CURVE ( 'NONE', #18153, #27001, #12195, .T. ) ;
#27279=EDGE_CURVE ( 'NONE', #25901, #6688, #16774, .T. ) ;
#27288=LINE ( 'NONE', #7628, #474 ) ;
#27292=CARTESIAN_POINT ( 'NONE',  ( -212.6433224921749456, 72.57850140501174963, -29.69533576542902154 ) ) ;
#27295=CYLINDRICAL_SURFACE ( 'NONE', #13898, 22.49999999999999289 ) ;
#27301=ORIENTED_EDGE ( 'NONE', *, *, #7852, .T. ) ;
#27312=CARTESIAN_POINT ( 'NONE',  ( 82.68942924499074820, 110.0997128786250840, -70.07812500014861712 ) ) ;
#27318=DIRECTION ( 'NONE',  ( -0.000000000000000000, -0.000000000000000000, -1.000000000000000000 ) ) ;
#27321=CARTESIAN_POINT ( 'NONE',  ( -38.50748414645865125, 128.7743013786471238, -17.17767432558748908 ) ) ;
#27322=AXIS2_PLACEMENT_3D ( 'NONE', #21643, #17469, #4673 ) ;
#27325=CARTESIAN_POINT ( 'NONE',  ( -207.5044420441007276, 75.59897387903043864, -45.00000000000000000 ) ) ;
#27330=TOROIDAL_SURFACE ( 'NONE', #3486, 33.76444293738737912, 9.999999999999996447 ) ;
#27337=CARTESIAN_POINT ( 'NONE',  ( -141.6428522700808230, 17.24192588826928585, 83.00000000000001421 ) ) ;
#27341=EDGE_CURVE ( 'NONE', #17217, #18102, #22954, .T. ) ;
#27343=EDGE_CURVE ( 'NONE', #17857, #4054, #6385, .T. ) ;
#27344=ADVANCED_FACE ( 'NONE', ( #25245 ), #12333, .F. ) ;
#27345=CARTESIAN_POINT ( 'NONE',  ( -127.2554728363764696, 130.3923307403294416, 16.55011143430600740 ) ) ;
#27347=CARTESIAN_POINT ( 'NONE',  ( 107.4212975031135642, 250.1603648754377502, 27.81198034436183164 ) ) ;
#27348=ORIENTED_EDGE ( 'NONE', *, *, #17194, .T. ) ;
#27350=EDGE_LOOP ( 'NONE', ( #9138, #9845, #2498, #12884 ) ) ;
#27353=ORIENTED_EDGE ( 'NONE', *, *, #23621, .F. ) ;
#27356=CARTESIAN_POINT ( 'NONE',  ( 109.4601507141017009, 253.2495769758999984, 39.14599534723758012 ) ) ;
#27358=DIRECTION ( 'NONE',  ( -0.000000000000000000, -0.000000000000000000, 1.000000000000000000 ) ) ;
#27362=CARTESIAN_POINT ( 'NONE',  ( 124.9999999999998579, 220.0000000000000284, 99.00000000000001421 ) ) ;
#27365=LINE ( 'NONE', #7574, #23108 ) ;
#27368=EDGE_CURVE ( 'NONE', #25995, #17824, #15047, .T. ) ;
#27369=CARTESIAN_POINT ( 'NONE',  ( 108.2137533302215360, 251.6609783837992040, -30.47578649309999577 ) ) ;
#27371=CARTESIAN_POINT ( 'NONE',  ( 33.10302365956999182, 203.2034914284457159, -13.00000000000000000 ) ) ;
#27380=ADVANCED_FACE ( 'NONE', ( #1675, #8146 ), #15044, .T. ) ;
#27383=ORIENTED_EDGE ( 'NONE', *, *, #21453, .F. ) ;
#27384=CARTESIAN_POINT ( 'NONE',  ( -82.71680601032872460, 136.4209726650630330, 13.49001633003910960 ) ) ;
#27385=VECTOR ( 'NONE', #12364, 1000.000000000000000 ) ;
#27388=CARTESIAN_POINT ( 'NONE',  ( -77.56758787812782430, 136.3063890311531736, -15.17881120916173110 ) ) ;
#27389=CARTESIAN_POINT ( 'NONE',  ( -1.260211142396240103, 135.5645450900976527, 13.59434970638475804 ) ) ;
#27390=CARTESIAN_POINT ( 'NONE',  ( -214.2457779686714900, 55.07866962813993439, 44.91461755630199804 ) ) ;
#27397=VERTEX_POINT ( 'NONE', #25662 ) ;
#27401=CARTESIAN_POINT ( 'NONE',  ( 144.9999999999998863, 220.0000000000000284, -90.00000000000002842 ) ) ;
#27404=VERTEX_POINT ( 'NONE', #14907 ) ;
#27405=AXIS2_PLACEMENT_3D ( 'NONE', #10164, #23372, #7449 ) ;
#27406=CIRCLE ( 'NONE', #3089, 414.0408555545579929 ) ;
#27411=EDGE_CURVE ( 'NONE', #23124, #20650, #9621, .T. ) ;
#27422=CARTESIAN_POINT ( 'NONE',  ( -68.57415822541635464, -18.01420295945611727, 100.0000000000000000 ) ) ;
#27426=CARTESIAN_POINT ( 'NONE',  ( -214.1728591254723142, 55.16903133821739402, -44.30008786503535845 ) ) ;
#27428=CARTESIAN_POINT ( 'NONE',  ( 179.9999999999999147, 330.0000000000000000, 100.0000000000000142 ) ) ;
#27432=ORIENTED_EDGE ( 'NONE', *, *, #23729, .T. ) ;
#27442=CARTESIAN_POINT ( 'NONE',  ( -227.8378063125350366, 130.6400894613935577, -13.00000000000000178 ) ) ;
#27443=CARTESIAN_POINT ( 'NONE',  ( 79.99999999999991473, 140.0000000000000000, 45.00000000000000000 ) ) ;
#27444=ORIENTED_EDGE ( 'NONE', *, *, #26220, .T. ) ;
#27445=EDGE_LOOP ( 'NONE', ( #9568, #14637, #26152 ) ) ;
#27446=CARTESIAN_POINT ( 'NONE',  ( 85.90765579575543143, 110.5723347142871091, -70.58593750016461854 ) ) ;
#27447=CARTESIAN_POINT ( 'NONE',  ( 109.5123478387949234, 253.5801691942621403, 39.43342786172818393 ) ) ;
#27449=FACE_OUTER_BOUND ( 'NONE', #7587, .T. ) ;
#27450=ORIENTED_EDGE ( 'NONE', *, *, #10194, .F. ) ;
#27451=CARTESIAN_POINT ( 'NONE',  ( -230.8465493730670346, 92.52399884504492888, 12.99999999980437160 ) ) ;
#27452=ORIENTED_EDGE ( 'NONE', *, *, #13849, .F. ) ;
#27455=AXIS2_PLACEMENT_3D ( 'NONE', #17979, #26734, #15842 ) ;
#27458=CARTESIAN_POINT ( 'NONE',  ( -40.48090269740500702, 130.4480578055027706, -16.52329147365227868 ) ) ;
#27463=CARTESIAN_POINT ( 'NONE',  ( -200.0139728499287060, 95.39988079771768525, -31.09496554298159765 ) ) ;
#27465=CARTESIAN_POINT ( 'NONE',  ( 134.9999999999998579, -327.2004514666934369, 84.99999999999995737 ) ) ;
#27466=ADVANCED_FACE ( 'NONE', ( #9243 ), #22745, .F. ) ;
#27467=CARTESIAN_POINT ( 'NONE',  ( 134.9999999999998579, 220.0000000000000284, -100.0000000000000142 ) ) ;
#27471=CARTESIAN_POINT ( 'NONE',  ( 116.8899838958982400, 233.3643110186103229, 99.51050955275449894 ) ) ;
#27476=DIRECTION ( 'NONE',  ( -0.000000000000000000, 1.000000000000000000, -1.387778780781445429E-16 ) ) ;
#27477=VERTEX_POINT ( 'NONE', #20298 ) ;
#27481=VERTEX_POINT ( 'NONE', #22879 ) ;
#27483=DIRECTION ( 'NONE',  ( 1.000000000000000000, 1.541976423090495880E-16, 0.000000000000000000 ) ) ;
#27486=EDGE_LOOP ( 'NONE', ( #9087, #25517, #19941, #22263 ) ) ;
#27487=AXIS2_PLACEMENT_3D ( 'NONE', #20684, #1004, #27558 ) ;
#27489=ORIENTED_EDGE ( 'NONE', *, *, #13000, .F. ) ;
#27490=ORIENTED_EDGE ( 'NONE', *, *, #24991, .F. ) ;
#27492=CARTESIAN_POINT ( 'NONE',  ( 109.5201339680880324, 255.4997179839102444, 37.19466046298244777 ) ) ;
#27500=CIRCLE ( 'NONE', #11016, 60.00000000000001421 ) ;
#27501=CARTESIAN_POINT ( 'NONE',  ( 134.9999999999998579, 220.0000000000000284, -100.0000000000000142 ) ) ;
#27503=EDGE_CURVE ( 'NONE', #5099, #4881, #26763, .T. ) ;
#27507=LINE ( 'NONE', #27233, #25841 ) ;
#27508=ORIENTED_EDGE ( 'NONE', *, *, #1128, .F. ) ;
#27509=CARTESIAN_POINT ( 'NONE',  ( -6.855911443193040355, 133.1088201606621624, 14.22081536340692942 ) ) ;
#27510=CYLINDRICAL_SURFACE ( 'NONE', #9645, 22.49999999999999289 ) ;
#27512=LINE ( 'NONE', #21198, #15074 ) ;
#27513=CARTESIAN_POINT ( 'NONE',  ( -146.6428522700808230, 74.54464929955099706, 83.00000000000001421 ) ) ;
#27517=EDGE_LOOP ( 'NONE', ( #13202, #20752, #6190, #25074 ) ) ;
#27520=ORIENTED_EDGE ( 'NONE', *, *, #19271, .T. ) ;
#27528=EDGE_CURVE ( 'NONE', #23088, #8776, #21070, .T. ) ;
#27529=CARTESIAN_POINT ( 'NONE',  ( -208.0231409554068875, 75.22252239880569391, 40.22632386312260167 ) ) ;
#27530=DIRECTION ( 'NONE',  ( -0.000000000000000000, 0.000000000000000000, 1.000000000000000000 ) ) ;
#27535=CARTESIAN_POINT ( 'NONE',  ( -214.1330451156402148, 86.77492310787303609, 22.28634443271844745 ) ) ;
#27542=CARTESIAN_POINT ( 'NONE',  ( -76.25760768171836901, 154.8982798170083299, -13.00000000000000000 ) ) ;
#27546=ORIENTED_EDGE ( 'NONE', *, *, #26829, .T. ) ;
#27547=ORIENTED_EDGE ( 'NONE', *, *, #25316, .T. ) ;
#27548=ORIENTED_EDGE ( 'NONE', *, *, #25672, .F. ) ;
#27549=AXIS2_PLACEMENT_3D ( 'NONE', #21290, #1609, #10379 ) ;
#27553=ORIENTED_EDGE ( 'NONE', *, *, #23729, .F. ) ;
#27558=DIRECTION ( 'NONE',  ( 0.6140342761796242499, -0.7892793597178155984, 0.000000000000000000 ) ) ;
#27560=DIRECTION ( 'NONE',  ( -0.000000000000000000, -0.000000000000000000, 1.000000000000000000 ) ) ;
#27564=DIRECTION ( 'NONE',  ( -0.000000000000000000, -0.000000000000000000, -1.000000000000000000 ) ) ;
#27566=CIRCLE ( 'NONE', #20692, 6.000000000000005329 ) ;
#27568=CARTESIAN_POINT ( 'NONE',  ( 134.9999999999998579, 220.0000000000000284, -90.00000000000002842 ) ) ;
#27573=CARTESIAN_POINT ( 'NONE',  ( -195.0817138475443357, 99.65346455659198455, 32.12633496786403953 ) ) ;
#27574=AXIS2_PLACEMENT_3D ( 'NONE', #6710, #24109, #15636 ) ;
#27578=ORIENTED_EDGE ( 'NONE', *, *, #24891, .F. ) ;
#27579=EDGE_CURVE ( 'NONE', #5481, #15436, #24965, .T. ) ;
#27580=ORIENTED_EDGE ( 'NONE', *, *, #12210, .F. ) ;
#27581=CARTESIAN_POINT ( 'NONE',  ( 104.4199312700443016, 89.58810137558876363, 100.0000000000000142 ) ) ;
#27583=ORIENTED_EDGE ( 'NONE', *, *, #22723, .T. ) ;
#27588=CARTESIAN_POINT ( 'NONE',  ( 109.8784069490710920, 256.7826562374864352, 42.21284981969159844 ) ) ;
#27593=VECTOR ( 'NONE', #17704, 1000.000000000000000 ) ;
#27596=CIRCLE ( 'NONE', #15246, 5.000000000000004441 ) ;
#27599=CARTESIAN_POINT ( 'NONE',  ( -43.02437977270766112, 129.7200458115293031, -16.81627168235288394 ) ) ;
#27602=CARTESIAN_POINT ( 'NONE',  ( -112.3221550338875687, 17.24192588826928585, 80.00000000000001421 ) ) ;
#27609=DIRECTION ( 'NONE',  ( 1.000000000000000000, 0.000000000000000000, 0.000000000000000000 ) ) ;
#27613=ORIENTED_EDGE ( 'NONE', *, *, #8905, .F. ) ;
#27614=AXIS2_PLACEMENT_3D ( 'NONE', #4900, #9222, #13690 ) ;
#27629=CARTESIAN_POINT ( 'NONE',  ( -68.57415822541635464, -23.01420295945612082, 95.00000000000000000 ) ) ;
#27630=ORIENTED_EDGE ( 'NONE', *, *, #17635, .F. ) ;
#27635=DIRECTION ( 'NONE',  ( 1.000000000000000000, 0.000000000000000000, 0.000000000000000000 ) ) ;
#27639=VECTOR ( 'NONE', #4435, 1000.000000000000000 ) ;
#27643=DIRECTION ( 'NONE',  ( 0.000000000000000000, 0.000000000000000000, 1.000000000000000000 ) ) ;
#27648=FACE_OUTER_BOUND ( 'NONE', #17039, .T. ) ;
#27650=DIRECTION ( 'NONE',  ( 0.000000000000000000, 0.000000000000000000, -1.000000000000000000 ) ) ;
#27653=ORIENTED_EDGE ( 'NONE', *, *, #17172, .T. ) ;
#27657=VERTEX_POINT ( 'NONE', #19127 ) ;
#27658=CARTESIAN_POINT ( 'NONE',  ( -254.3350114625770289, -91.18033988749901653, 0.000000000000000000 ) ) ;
#27660=AXIS2_PLACEMENT_3D ( 'NONE', #17764, #26957, #26514 ) ;
#27668=DIRECTION ( 'NONE',  ( 0.9960550913260672878, 0.000000000000000000, -0.08873699929240064233 ) ) ;
#27669=CARTESIAN_POINT ( 'NONE',  ( -152.1970234707412146, 122.9096046473621868, -20.33815154695436078 ) ) ;
#27670=AXIS2_PLACEMENT_3D ( 'NONE', #23554, #6022, #14797 ) ;
#27676=EDGE_CURVE ( 'NONE', #27404, #7140, #1784, .T. ) ;
#27678=CARTESIAN_POINT ( 'NONE',  ( -216.6938019150388186, 86.34331246501530188, 20.61264131666953503 ) ) ;
#27684=ADVANCED_FACE ( 'NONE', ( #21423 ), #8260, .T. ) ;
#27695=EDGE_CURVE ( 'NONE', #20120, #970, #24866, .T. ) ;
#27698=AXIS2_PLACEMENT_3D ( 'NONE', #177, #24449, #8937 ) ;
#27702=DIRECTION ( 'NONE',  ( -0.000000000000000000, 1.000000000000000000, -1.387778780781445429E-16 ) ) ;
#27703=CARTESIAN_POINT ( 'NONE',  ( -180.0000000000000284, -40.00000000000004974, 70.00000000000001421 ) ) ;
#27704=DIRECTION ( 'NONE',  ( -0.000000000000000000, -0.000000000000000000, -1.000000000000000000 ) ) ;
#27710=CYLINDRICAL_SURFACE ( 'NONE', #23807, 30.00000000000000000 ) ;
#27714=ORIENTED_EDGE ( 'NONE', *, *, #1241, .T. ) ;
#27715=CARTESIAN_POINT ( 'NONE',  ( -191.5190414516356441, 102.2994403167507329, 32.46908855772340985 ) ) ;
#27726=ORIENTED_EDGE ( 'NONE', *, *, #18724, .T. ) ;
#27728=VECTOR ( 'NONE', #6306, 1000.000000000000000 ) ;
#27735=ORIENTED_EDGE ( 'NONE', *, *, #6908, .T. ) ;
#27736=CARTESIAN_POINT ( 'NONE',  ( -231.9378824387731015, 93.53122965655664700, 14.99999999999999289 ) ) ;
#27741=DIRECTION ( 'NONE',  ( -0.2500000000000127121, 0.000000000000000000, -0.9682458365518510357 ) ) ;
#27745=CARTESIAN_POINT ( 'NONE',  ( -201.6488700512677212, 93.99433454770324659, -30.47120949752622820 ) ) ;
#27749=DIRECTION ( 'NONE',  ( 1.000000000000000000, 0.000000000000000000, -0.000000000000000000 ) ) ;
#27752=VERTEX_POINT ( 'NONE', #15499 ) ;
#27758=CARTESIAN_POINT ( 'NONE',  ( -209.0203365101457109, 89.44154586134021656, 24.30531738582797274 ) ) ;
#27764=CARTESIAN_POINT ( 'NONE',  ( -157.8108137764193373, 120.7058031521935391, 21.99230116549754399 ) ) ;
#27766=ORIENTED_EDGE ( 'NONE', *, *, #12133, .F. ) ;
#27767=ORIENTED_EDGE ( 'NONE', *, *, #24014, .T. ) ;
#27771=EDGE_CURVE ( 'NONE', #25890, #27860, #26110, .T. ) ;
#27772=VECTOR ( 'NONE', #12481, 1000.000000000000000 ) ;
#27775=AXIS2_PLACEMENT_3D ( 'NONE', #21465, #10558, #6100 ) ;
#27784=CARTESIAN_POINT ( 'NONE',  ( -231.0952835391973963, 75.72709865443405874, -15.86948571459950053 ) ) ;
#27785=EDGE_CURVE ( 'NONE', #18799, #3986, #23947, .T. ) ;
#27786=CYLINDRICAL_SURFACE ( 'NONE', #305, 5.000000000000000888 ) ;
#27788=DIRECTION ( 'NONE',  ( 1.000000000000000000, 0.000000000000000000, 0.000000000000000000 ) ) ;
#27797=AXIS2_PLACEMENT_3D ( 'NONE', #26643, #2224, #373 ) ;
#27798=CARTESIAN_POINT ( 'NONE',  ( -236.8177751472017007, 82.33896643611701904, 15.00000000000000000 ) ) ;
#27801=ORIENTED_EDGE ( 'NONE', *, *, #26805, .T. ) ;
#27808=CARTESIAN_POINT ( 'NONE',  ( -47.91415621944423719, 130.8825976540551608, -16.39223340224337733 ) ) ;
#27810=CARTESIAN_POINT ( 'NONE',  ( -127.4043536527376688, 130.3575739508328013, -16.56241948173741463 ) ) ;
#27811=AXIS2_PLACEMENT_3D ( 'NONE', #20333, #18329, #20189 ) ;
#27814=CARTESIAN_POINT ( 'NONE',  ( 32.36067977499786252, -40.00000000000003553, 100.0000000000000142 ) ) ;
#27815=CARTESIAN_POINT ( 'NONE',  ( -230.8931271727480805, 92.61283034429897043, -15.05361674725927301 ) ) ;
#27817=CARTESIAN_POINT ( 'NONE',  ( -226.2800442625073174, 87.57925215467369640, 16.13539826775552299 ) ) ;
#27823=EDGE_CURVE ( 'NONE', #13440, #1333, #26577, .T. ) ;
#27825=EDGE_CURVE ( 'NONE', #1063, #3920, #16889, .T. ) ;
#27829=CARTESIAN_POINT ( 'NONE',  ( 104.2862437451156126, 245.6633304404597595, -27.19020029359707991 ) ) ;
#27830=EDGE_LOOP ( 'NONE', ( #13134, #13774, #3010 ) ) ;
#27834=CIRCLE ( 'NONE', #19131, 6.025000000000002132 ) ;
#27836=ORIENTED_EDGE ( 'NONE', *, *, #25848, .T. ) ;
#27848=EDGE_CURVE ( 'NONE', #7637, #17545, #7729, .T. ) ;
#27850=EDGE_CURVE ( 'NONE', #27055, #7931, #20553, .T. ) ;
#27851=FACE_OUTER_BOUND ( 'NONE', #11396, .T. ) ;
#27852=CARTESIAN_POINT ( 'NONE',  ( -146.6428522700808230, 69.54464929955099706, 83.00000000000001421 ) ) ;
#27856=CARTESIAN_POINT ( 'NONE',  ( 109.9999999999999005, 3.816391647148972452E-14, 100.0000000000000142 ) ) ;
#27857=ORIENTED_EDGE ( 'NONE', *, *, #18909, .F. ) ;
#27859=ORIENTED_EDGE ( 'NONE', *, *, #23217, .F. ) ;
#27860=VERTEX_POINT ( 'NONE', #9311 ) ;
#27867=DIRECTION ( 'NONE',  ( 1.000000000000000000, 0.000000000000000000, 0.000000000000000000 ) ) ;
#27868=CARTESIAN_POINT ( 'NONE',  ( -186.8771810018902499, 105.5597884250916678, -31.69226466690710353 ) ) ;
#27875=CIRCLE ( 'NONE', #13706, 9.999999999999985789 ) ;
#27876=DIRECTION ( 'NONE',  ( 0.000000000000000000, 0.000000000000000000, -1.000000000000000000 ) ) ;
#27878=CARTESIAN_POINT ( 'NONE',  ( -42.53273978471831640, 130.9733465240572627, -14.93735646117640492 ) ) ;
#27880=DIRECTION ( 'NONE',  ( 1.850371707708594316E-16, -1.000000000000000000, 0.000000000000000000 ) ) ;
#27883=ORIENTED_EDGE ( 'NONE', *, *, #13572, .F. ) ;
#27885=EDGE_CURVE ( 'NONE', #5248, #18456, #27875, .T. ) ;
#27886=CIRCLE ( 'NONE', #22864, 10.00000000000000888 ) ;
#27889=CARTESIAN_POINT ( 'NONE',  ( -180.0000000000000284, -50.00000000000004263, 98.28427124746191623 ) ) ;
#27892=LINE ( 'NONE', #8095, #4737 ) ;
#27902=CARTESIAN_POINT ( 'NONE',  ( -241.9743096803475453, -91.18033988749901653, 0.000000000000000000 ) ) ;
#27906=ORIENTED_EDGE ( 'NONE', *, *, #12211, .T. ) ;
#27914=CARTESIAN_POINT ( 'NONE',  ( 119.9999999999999005, 203.2294901687515960, -100.0000000000000142 ) ) ;
#27916=CARTESIAN_POINT ( 'NONE',  ( -216.3288264717409106, 60.34946693787968286, -12.99564918865353569 ) ) ;
#27922=DIRECTION ( 'NONE',  ( -0.000000000000000000, 1.000000000000000000, -1.387778780781445429E-16 ) ) ;
#27923=CARTESIAN_POINT ( 'NONE',  ( 112.5004877479093892, 221.0403377251794836, -96.61493133138624501 ) ) ;
#27928=LINE ( 'NONE', #6113, #6999 ) ;
#27929=SPHERICAL_SURFACE ( 'NONE', #19717, 5.000000000000000000 ) ;
#27930=DIRECTION ( 'NONE',  ( 0.000000000000000000, -1.000000000000000000, 0.000000000000000000 ) ) ;
#27932=ORIENTED_EDGE ( 'NONE', *, *, #508, .F. ) ;
#27933=CIRCLE ( 'NONE', #7334, 9.999999999999996447 ) ;
#27944=ORIENTED_EDGE ( 'NONE', *, *, #67, .T. ) ;
#27945=CARTESIAN_POINT ( 'NONE',  ( 113.9142275403300459, 212.0873699598490134, 97.94883453769585913 ) ) ;
#27949=FACE_OUTER_BOUND ( 'NONE', #4311, .T. ) ;
#27950=VECTOR ( 'NONE', #14619, 1000.000000000000000 ) ;
#27953=CARTESIAN_POINT ( 'NONE',  ( 28.53653844984206955, -43.59399515434488137, 99.78583825828528120 ) ) ;
#27954=CARTESIAN_POINT ( 'NONE',  ( -216.2184996979340497, 87.78057762432685251, -20.45253552124680851 ) ) ;
#27956=CARTESIAN_POINT ( 'NONE',  ( -233.2943309833541718, 92.06151970357194614, 15.00000000000000000 ) ) ;
#27962=EDGE_CURVE ( 'NONE', #16662, #4224, #17871, .T. ) ;
#27965=CARTESIAN_POINT ( 'NONE',  ( -279.3160071107327553, -91.18033988749907337, 0.000000000000000000 ) ) ;
#27969=CIRCLE ( 'NONE', #22949, 33.76444293738739333 ) ;
#27971=CARTESIAN_POINT ( 'NONE',  ( 94.98941689213211248, 231.7050943134732108, -19.00901305069148961 ) ) ;
#27975=EDGE_CURVE ( 'NONE', #18824, #13911, #27512, .T. ) ;
#27976=ORIENTED_EDGE ( 'NONE', *, *, #11863, .T. ) ;
#27977=EDGE_LOOP ( 'NONE', ( #24013, #17453, #14903, #1199 ) ) ;
#27979=ORIENTED_EDGE ( 'NONE', *, *, #1295, .F. ) ;
#27985=ADVANCED_FACE ( 'NONE', ( #25229 ), #1239, .T. ) ;
#27989=CARTESIAN_POINT ( 'NONE',  ( 134.9999999999998579, 220.0000000000000284, -99.00000000000001421 ) ) ;
#27990=CARTESIAN_POINT ( 'NONE',  ( -107.3221550338875687, 22.24192588826928585, 83.00000000000001421 ) ) ;
#27991=CYLINDRICAL_SURFACE ( 'NONE', #4252, 16.46313063346208239 ) ;
#27992=CARTESIAN_POINT ( 'NONE',  ( -38.26150398323100887, 130.0131485130493729, 16.67769045341279011 ) ) ;
#27994=EDGE_CURVE ( 'NONE', #1940, #6895, #16003, .T. ) ;
#27999=AXIS2_PLACEMENT_3D ( 'NONE', #25592, #7802, #7940 ) ;
#28006=CARTESIAN_POINT ( 'NONE',  ( 82.91040908012763566, 80.00000000660637056, 100.0000000000000142 ) ) ;
#28008=ORIENTED_EDGE ( 'NONE', *, *, #26454, .F. ) ;
#28011=CARTESIAN_POINT ( 'NONE',  ( 105.2480867101029531, 123.6573351780301095, -85.93750000029402258 ) ) ;
#28012=EDGE_CURVE ( 'NONE', #8519, #23293, #6338, .T. ) ;
#28017=CARTESIAN_POINT ( 'NONE',  ( 113.4920585194047078, 104.4775165427241319, 100.0000000000000142 ) ) ;
#28019=DIRECTION ( 'NONE',  ( 0.000000000000000000, 0.000000000000000000, 1.000000000000000000 ) ) ;
#28023=AXIS2_PLACEMENT_3D ( 'NONE', #2454, #4756, #4607 ) ;
#28025=CYLINDRICAL_SURFACE ( 'NONE', #15993, 22.49999999999999289 ) ;
#28029=CARTESIAN_POINT ( 'NONE',  ( -180.0000000000000284, -70.00000000000004263, 70.00000000000000000 ) ) ;
#28030=ORIENTED_EDGE ( 'NONE', *, *, #16693, .T. ) ;
#28032=CARTESIAN_POINT ( 'NONE',  ( -254.4816742664885965, 103.7585653882801182, 5.000000000000002665 ) ) ;
#28035=VERTEX_POINT ( 'NONE', #4238 ) ;
#28038=AXIS2_PLACEMENT_3D ( 'NONE', #9077, #19991, #323 ) ;
#28039=CARTESIAN_POINT ( 'NONE',  ( 65.00000000000000000, -120.0000000000000995, -69.99999999999998579 ) ) ;
#28040=CARTESIAN_POINT ( 'NONE',  ( -174.7479038800345563, 112.7071446407698403, -28.86810097183760959 ) ) ;
#28043=CIRCLE ( 'NONE', #27156, 6.204828372381208546 ) ;
#28044=VECTOR ( 'NONE', #16862, 1000.000000000000000 ) ;
#28045=EDGE_LOOP ( 'NONE', ( #1634, #5222, #26972, #19194 ) ) ;
#28047=DIRECTION ( 'NONE',  ( 0.5804519453834686704, -0.8142945039115434547, 0.000000000000000000 ) ) ;
#28051=ORIENTED_EDGE ( 'NONE', *, *, #24162, .T. ) ;
#28052=EDGE_LOOP ( 'NONE', ( #14228, #27139, #26609, #19084 ) ) ;
#28053=LINE ( 'NONE', #25495, #20331 ) ;
#28054=FACE_OUTER_BOUND ( 'NONE', #7582, .T. ) ;
#28056=CARTESIAN_POINT ( 'NONE',  ( -207.5044420441007560, 75.59897387903042443, 45.00000000000000000 ) ) ;
#28057=CARTESIAN_POINT ( 'NONE',  ( 119.1248245724174524, 204.0122708680763424, -100.0000000000000000 ) ) ;
#28059=CARTESIAN_POINT ( 'NONE',  ( -235.5446291276663828, 67.70753763449675944, -5.872244511705135395 ) ) ;
#28065=DIRECTION ( 'NONE',  ( 0.000000000000000000, 0.000000000000000000, 1.000000000000000000 ) ) ;
#28066=CARTESIAN_POINT ( 'NONE',  ( 113.1867617905510173, 225.5391268416508694, -97.32202223992345580 ) ) ;
#28073=DIRECTION ( 'NONE',  ( 0.000000000000000000, 0.000000000000000000, -1.000000000000000000 ) ) ;
#28075=FACE_OUTER_BOUND ( 'NONE', #15364, .T. ) ;
#28078=DIRECTION ( 'NONE',  ( -0.000000000000000000, -0.000000000000000000, -1.000000000000000000 ) ) ;
#28082=AXIS2_PLACEMENT_3D ( 'NONE', #5286, #14068, #20654 ) ;
#28084=CARTESIAN_POINT ( 'NONE',  ( -77.63961834651543370, 136.2561492527889015, 15.18776799126392163 ) ) ;
#28085=CIRCLE ( 'NONE', #26724, 6.025000000000002132 ) ;
#28086=EDGE_CURVE ( 'NONE', #26198, #9545, #1936, .T. ) ;
#28089=AXIS2_PLACEMENT_3D ( 'NONE', #21833, #10915, #5607 ) ;
#28090=CARTESIAN_POINT ( 'NONE',  ( -219.9082363642798441, 137.1815813412079308, 12.98324324887168402 ) ) ;
#28091=CARTESIAN_POINT ( 'NONE',  ( -155.5576584249185146, 121.6218958557625740, -21.26367854068186958 ) ) ;
#28095=CARTESIAN_POINT ( 'NONE',  ( -142.3432792462832310, 127.5062405277896147, -16.40804776362093875 ) ) ;
#28098=CARTESIAN_POINT ( 'NONE',  ( -212.5557490532361840, 88.28325300605492032, -22.89340189428408578 ) ) ;
#28107=AXIS2_PLACEMENT_3D ( 'NONE', #16238, #5303, #14084 ) ;
#28108=CARTESIAN_POINT ( 'NONE',  ( 114.9638101962909360, 140.0000000000000000, 98.73786388354261589 ) ) ;
#28109=LINE ( 'NONE', #24240, #3876 ) ;
#28110=DIRECTION ( 'NONE',  ( -0.000000000000000000, 1.000000000000000000, -1.387778780781445429E-16 ) ) ;
#28112=EDGE_LOOP ( 'NONE', ( #5491, #11631 ) ) ;
#28115=EDGE_CURVE ( 'NONE', #3252, #2009, #8698, .T. ) ;
#28116=CARTESIAN_POINT ( 'NONE',  ( 105.5907556405606158, 242.1385898947462465, -29.32397797500748737 ) ) ;
#28119=VERTEX_POINT ( 'NONE', #6815 ) ;
#28120=ORIENTED_EDGE ( 'NONE', *, *, #23521, .T. ) ;
#28124=CARTESIAN_POINT ( 'NONE',  ( 0.000000000000000000, 0.000000000000000000, 25.00000000000000000 ) ) ;
#28134=CARTESIAN_POINT ( 'NONE',  ( 109.9999999999999005, 240.0000000000000284, -5.000000000000004441 ) ) ;
#28138=CARTESIAN_POINT ( 'NONE',  ( -207.7351949253619239, 74.89624901011349323, 43.85536788017862619 ) ) ;
#28143=CARTESIAN_POINT ( 'NONE',  ( -188.7947732573136648, 104.2412161718895476, 31.96204269770191431 ) ) ;
#28149=EDGE_LOOP ( 'NONE', ( #12428, #15608, #19338, #5732 ) ) ;
#28155=CARTESIAN_POINT ( 'NONE',  ( 106.3487426207649236, 91.82653269718771583, -100.0000000000000142 ) ) ;
#28156=MANIFOLD_SOLID_BREP ( 'Cut-Extrude13', #9978 ) ;
#28161=CARTESIAN_POINT ( 'NONE',  ( -216.9923549404892071, 86.31376438289755981, 20.42942837940906742 ) ) ;
#28175=CARTESIAN_POINT ( 'NONE',  ( -40.40953891503691153, 0.000000000000000000, 99.00000000000000000 ) ) ;
#28177=CARTESIAN_POINT ( 'NONE',  ( -180.7604701752530332, 109.5394202030439317, 30.00180410819614352 ) ) ;
#28178=CARTESIAN_POINT ( 'NONE',  ( -43.02437977270766822, 129.7200458115293031, -16.81627168235288394 ) ) ;
#28182=ORIENTED_EDGE ( 'NONE', *, *, #17846, .T. ) ;
#28184=CARTESIAN_POINT ( 'NONE',  ( -155.5799833640026577, 121.6126019772860474, 21.27136890865478946 ) ) ;
#28185=CARTESIAN_POINT ( 'NONE',  ( -172.9314056506308361, 113.6797141081297298, -28.12266984373487588 ) ) ;
#28189=DIRECTION ( 'NONE',  ( -0.000000000000000000, -0.000000000000000000, -1.000000000000000000 ) ) ;
#28192=ORIENTED_EDGE ( 'NONE', *, *, #14537, .F. ) ;
#28193=DIRECTION ( 'NONE',  ( 0.000000000000000000, 0.000000000000000000, -1.000000000000000000 ) ) ;
#28197=DIRECTION ( 'NONE',  ( 0.2499999999999988898, 0.000000000000000000, -0.9682458365518545884 ) ) ;
#28202=CARTESIAN_POINT ( 'NONE',  ( -222.1142713348111783, 61.47487629661259945, -10.02481564198514619 ) ) ;
#28204=CARTESIAN_POINT ( 'NONE',  ( 112.4999999999998863, 220.0000000000000284, -99.00000000000001421 ) ) ;
#28212=CARTESIAN_POINT ( 'NONE',  ( 89.99999999999994316, -40.00000000000002132, -70.00000000000001421 ) ) ;
#28214=EDGE_CURVE ( 'NONE', #17712, #5857, #5235, .T. ) ;
#28216=FACE_OUTER_BOUND ( 'NONE', #4000, .T. ) ;
#28220=VERTEX_POINT ( 'NONE', #14024 ) ;
#28225=CIRCLE ( 'NONE', #15875, 58.90601976618767566 ) ;
#28226=EDGE_LOOP ( 'NONE', ( #25269, #17803, #16077, #7915 ) ) ;
#28231=DIRECTION ( 'NONE',  ( 1.000000000000000000, 0.000000000000000000, 0.000000000000000000 ) ) ;
#28235=CARTESIAN_POINT ( 'NONE',  ( -160.0000000000000568, 90.00000000000001421, 110.0000000000000284 ) ) ;
#28240=CARTESIAN_POINT ( 'NONE',  ( -224.4622899665858711, 89.01046014348733593, -16.48139453409665833 ) ) ;
#28242=CIRCLE ( 'NONE', #3011, 5.000000000000000888 ) ;
#28244=CARTESIAN_POINT ( 'NONE',  ( 89.99999999999994316, -90.00000000000001421, -70.00000000000001421 ) ) ;
#28246=FACE_OUTER_BOUND ( 'NONE', #16937, .T. ) ;
#28247=VECTOR ( 'NONE', #11149, 1000.000000000000000 ) ;
#28248=ORIENTED_EDGE ( 'NONE', *, *, #1563, .T. ) ;
#28249=CARTESIAN_POINT ( 'NONE',  ( 79.99999999999992895, 110.0000000000000000, 45.00000000000000000 ) ) ;
#28251=DIRECTION ( 'NONE',  ( -1.000000000000000000, 0.000000000000000000, 0.000000000000000000 ) ) ;
#28256=ADVANCED_FACE ( 'NONE', ( #26933 ), #11434, .F. ) ;
#28257=CARTESIAN_POINT ( 'NONE',  ( 89.37316688736883918, 230.0797033051251788, -16.48577246127781493 ) ) ;
#28259=CARTESIAN_POINT ( 'NONE',  ( -38.16446318061785092, 129.9977304598137948, -15.32283089668279530 ) ) ;
#28262=ORIENTED_EDGE ( 'NONE', *, *, #52, .F. ) ;
#28266=DIRECTION ( 'NONE',  ( 0.000000000000000000, 0.000000000000000000, 1.000000000000000000 ) ) ;
#28275=CARTESIAN_POINT ( 'NONE',  ( 89.99999999999988631, 260.0000000000000000, 15.00000000000000000 ) ) ;
#28276=DIRECTION ( 'NONE',  ( 0.000000000000000000, -0.000000000000000000, 1.000000000000000000 ) ) ;
#28282=AXIS2_PLACEMENT_3D ( 'NONE', #27902, #9985, #1767 ) ;
#28283=DIRECTION ( 'NONE',  ( -0.000000000000000000, 1.000000000000000000, -0.000000000000000000 ) ) ;
#28287=ORIENTED_EDGE ( 'NONE', *, *, #21515, .T. ) ;
#28291=LINE ( 'NONE', #11221, #13901 ) ;
#28293=ORIENTED_EDGE ( 'NONE', *, *, #26503, .T. ) ;
#28294=EDGE_CURVE ( 'NONE', #15527, #18881, #14570, .T. ) ;
#28295=CARTESIAN_POINT ( 'NONE',  ( 104.1118574116271418, 122.0584436054305684, -99.99999999997839950 ) ) ;
#28299=CARTESIAN_POINT ( 'NONE',  ( -217.9474420836749289, 87.77798100153485450, 17.55735672534662228 ) ) ;
#28300=ORIENTED_EDGE ( 'NONE', *, *, #27823, .T. ) ;
#28303=DIRECTION ( 'NONE',  ( 0.000000000000000000, 0.000000000000000000, -1.000000000000000000 ) ) ;
#28306=CARTESIAN_POINT ( 'NONE',  ( 116.8936292565948776, 206.6308718070802684, 99.51164200157786865 ) ) ;
#28313=AXIS2_PLACEMENT_3D ( 'NONE', #2168, #26163, #28303 ) ;
#28314=EDGE_CURVE ( 'NONE', #2370, #14118, #14765, .T. ) ;
#28315=CARTESIAN_POINT ( 'NONE',  ( -164.5581833258768825, 118.4903777742713658, 22.95450677488445024 ) ) ;
#28316=CARTESIAN_POINT ( 'NONE',  ( -221.7385414042798573, 88.25646530137930768, 15.53772012378376566 ) ) ;
#28318=ORIENTED_EDGE ( 'NONE', *, *, #23327, .F. ) ;
#28320=CARTESIAN_POINT ( 'NONE',  ( -190.0000000000000284, -40.00000000000004974, 110.0000000000000284 ) ) ;
#28321=CARTESIAN_POINT ( 'NONE',  ( -186.6633805910676642, 105.4812463994875884, -32.52244268913835867 ) ) ;
#28325=CARTESIAN_POINT ( 'NONE',  ( 144.9999999999998863, 220.0000000000000284, -90.00000000000002842 ) ) ;
#28326=CARTESIAN_POINT ( 'NONE',  ( 4.996003610813208850E-14, -120.0000000000001137, 25.00000000000000000 ) ) ;
#28330=LINE ( 'NONE', #197, #11637 ) ;
#28332=CIRCLE ( 'NONE', #20545, 30.49120955644046660 ) ;
#28333=TOROIDAL_SURFACE ( 'NONE', #17794, 14.95564396479129243, 3.532530335305412716 ) ;
#28334=CARTESIAN_POINT ( 'NONE',  ( 134.9999999999998579, 220.0000000000000284, -90.00000000000002842 ) ) ;
#28337=CARTESIAN_POINT ( 'NONE',  ( 20.92655468430566756, 155.3461090732848220, -15.00000000000000000 ) ) ;
#28347=CARTESIAN_POINT ( 'NONE',  ( -28.05246235954390244, 188.0718642840173516, -15.00000000000000000 ) ) ;
#28363=DIRECTION ( 'NONE',  ( 0.000000000000000000, 0.000000000000000000, 1.000000000000000000 ) ) ;
#28366=AXIS2_PLACEMENT_3D ( 'NONE', #5328, #9371, #24588 ) ;
#28369=DIRECTION ( 'NONE',  ( 0.000000000000000000, 0.000000000000000000, 1.000000000000000000 ) ) ;
#28370=DIRECTION ( 'NONE',  ( -0.6787614006938686995, -0.7343588774761953264, 0.000000000000000000 ) ) ;
#28371=AXIS2_PLACEMENT_3D ( 'NONE', #14952, #1854, #24137 ) ;
#28373=CARTESIAN_POINT ( 'NONE',  ( -215.0361879928736073, 86.55905346095244113, -21.66337491047849895 ) ) ;
#28377=DIRECTION ( 'NONE',  ( 1.000000000000000000, 8.673617379884036705E-17, 0.000000000000000000 ) ) ;
#28378=CARTESIAN_POINT ( 'NONE',  ( -189.8086322075389774, 92.49158130768422836, -13.00000000000000000 ) ) ;
#28387=CARTESIAN_POINT ( 'NONE',  ( 88.44954299047357438, 230.0000000005625225, -16.19779584935188055 ) ) ;
#28389=CARTESIAN_POINT ( 'NONE',  ( -23.72680257353332678, 129.3221895177523777, -15.61617233342094302 ) ) ;
#28390=ORIENTED_EDGE ( 'NONE', *, *, #27273, .T. ) ;
#28391=AXIS2_PLACEMENT_3D ( 'NONE', #18152, #26906, #7658 ) ;
#28394=EDGE_CURVE ( 'NONE', #20507, #6925, #2359, .T. ) ;
#28395=EDGE_LOOP ( 'NONE', ( #12254, #27036, #14289, #2262, #10732, #25943, #12271, #6287, #12252, #9599, #2620, #16347, #9672, #20074, #4815 ) ) ;
#28396=ORIENTED_EDGE ( 'NONE', *, *, #27074, .F. ) ;
#28398=CARTESIAN_POINT ( 'NONE',  ( 89.99999999999994316, -40.00000000000002842, -100.0000000000000142 ) ) ;
#28399=CARTESIAN_POINT ( 'NONE',  ( -40.48066117626728300, 130.4479960067108095, 16.52331096680928368 ) ) ;
#28449=COLOUR_RGB('Off White',0.89,0.88,0.83);
#28450=FILL_AREA_STYLE_COLOUR('',#28449);
#28451=FILL_AREA_STYLE('',(#28450));
#28452=SURFACE_STYLE_FILL_AREA(#28451);
#28453=SURFACE_SIDE_STYLE('',(#28452));
#28454=SURFACE_STYLE_USAGE(.BOTH.,#28453);
#28455=PRESENTATION_STYLE_ASSIGNMENT((#28454));
ENDSEC;
END-ISO-10303-21;
